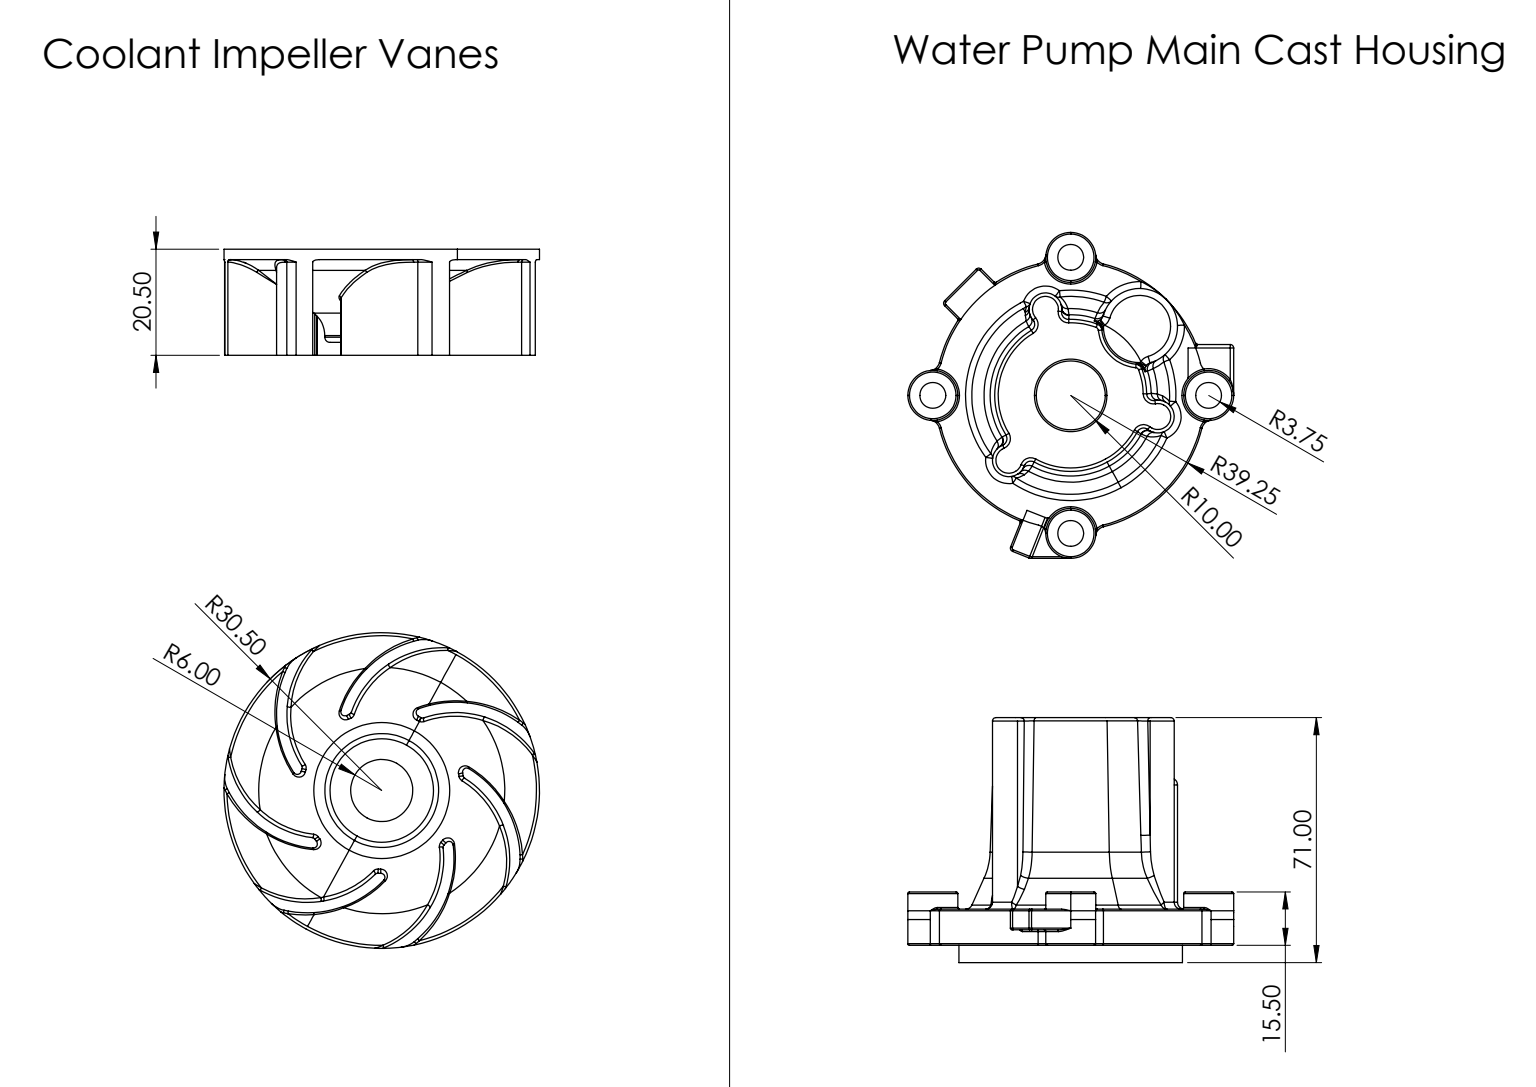
ISO-10303-21;
HEADER;
FILE_DESCRIPTION (('STEP AP214'),
    '1' );
FILE_NAME ('Water Pump Main Cast Housing.step',
    '2026-10-09T13:19:41',
    ( '' ),
    ( '' ),
    'SwSTEP 2.0',
    'SolidWorks 2026',
    '' );
FILE_SCHEMA (( 'AUTOMOTIVE_DESIGN' ));
ENDSEC;

DATA;
#2=DIRECTION ( 'NONE',  ( -1.000000000000000000, 0.000000000000000000, -1.110223024630000146E-15 ) ) ;
#4=CARTESIAN_POINT ( 'NONE',  ( 36.82697894980000086, -80.49999984420000487, -13.57704391360000074 ) ) ;
#5=CARTESIAN_POINT ( 'NONE',  ( 11.49840686428493441, -72.20801872445015590, -27.07840416834825348 ) ) ;
#6=CARTESIAN_POINT ( 'NONE',  ( -18.42950098929999925, -19.15770089200000115, 12.27996177870000061 ) ) ;
#7=ORIENTED_EDGE ( 'NONE', *, *, #8559, .F. ) ;
#11=DIRECTION ( 'NONE',  ( 0.000000000000000000, -1.000000000000000000, 0.000000000000000000 ) ) ;
#15=AXIS2_PLACEMENT_3D ( 'NONE', #13983, #16160, #22740 ) ;
#21=ADVANCED_FACE ( 'NONE', ( #16761 ), #3074, .F. ) ;
#23=CARTESIAN_POINT ( 'NONE',  ( -13.70187146130000144, -57.41946977620000325, 20.98050236089999743 ) ) ;
#24=CARTESIAN_POINT ( 'NONE',  ( -21.94602169939999925, -74.00000000000000000, -32.01791432939999993 ) ) ;
#30=CARTESIAN_POINT ( 'NONE',  ( -7.249922261819999214, -74.00000000000000000, 40.03357376379999977 ) ) ;
#32=CARTESIAN_POINT ( 'NONE',  ( 47.25000000000000000, -79.07667144713899177, -0.2614142261083034491 ) ) ;
#33=ORIENTED_EDGE ( 'NONE', *, *, #25582, .F. ) ;
#35=CARTESIAN_POINT ( 'NONE',  ( 41.00000000000000000, -82.25000000000000000, -10.20110288159999890 ) ) ;
#40=CARTESIAN_POINT ( 'NONE',  ( -38.65569705749999940, -74.00000000000000000, 7.472970580910000216 ) ) ;
#43=ORIENTED_EDGE ( 'NONE', *, *, #10677, .T. ) ;
#49=CARTESIAN_POINT ( 'NONE',  ( 7.691676892869999449, -59.03425911290000272, -22.18797527670000136 ) ) ;
#50=CARTESIAN_POINT ( 'NONE',  ( -12.44168150949999863, -68.42644193349998716, -23.76792160109999585 ) ) ;
#51=CARTESIAN_POINT ( 'NONE',  ( 23.24173891719999929, -63.62917541130000387, -7.733004683649999045 ) ) ;
#52=CARTESIAN_POINT ( 'NONE',  ( 26.61465604159999998, -68.28989644159999273, 0.1578853838729999959 ) ) ;
#53=CARTESIAN_POINT ( 'NONE',  ( 40.75609756099999714, -80.50000000000000000, -7.713029007999999465 ) ) ;
#55=ADVANCED_FACE ( 'NONE', ( #15109 ), #24277, .F. ) ;
#57=FACE_OUTER_BOUND ( 'NONE', #7313, .T. ) ;
#59=ORIENTED_EDGE ( 'NONE', *, *, #8938, .T. ) ;
#63=CIRCLE ( 'NONE', #7047, 3.000000000000002665 ) ;
#65=CARTESIAN_POINT ( 'NONE',  ( 19.49531202280000031, -22.51609091130000095, -8.976487791660000326 ) ) ;
#66=CARTESIAN_POINT ( 'NONE',  ( 22.75333808661257606, -19.47282734142590499, 1.034408943893888599 ) ) ;
#68=ORIENTED_EDGE ( 'NONE', *, *, #28286, .T. ) ;
#69=CARTESIAN_POINT ( 'NONE',  ( 26.87524702870645044, -72.43548166874914784, -11.03468220454692883 ) ) ;
#71=CARTESIAN_POINT ( 'NONE',  ( 8.702528184260000188, -36.35983078039999583, -21.11894135150000196 ) ) ;
#73=PLANE ( 'NONE',  #14194 ) ;
#74=CARTESIAN_POINT ( 'NONE',  ( 22.07903221200000132, -19.15751145089999952, 0.09883320182290000755 ) ) ;
#80=CARTESIAN_POINT ( 'NONE',  ( 7.120909764619999412E-15, -73.00000000000000000, 40.00000000000000000 ) ) ;
#86=TOROIDAL_SURFACE ( 'NONE', #19140, 38.75000000000000000, 0.5000000000000000000 ) ;
#89=CARTESIAN_POINT ( 'NONE',  ( 36.71918983540000880, -74.79610922010000706, -14.73254090590000054 ) ) ;
#90=VECTOR ( 'NONE', #20251, 1000.000000000000000 ) ;
#93=CARTESIAN_POINT ( 'NONE',  ( -13.96596450430000047, -64.58097845250000546, 21.73803617189999926 ) ) ;
#94=CARTESIAN_POINT ( 'NONE',  ( 7.237400523855146872, -74.28469014324819852, 40.42867112560485054 ) ) ;
#96=CARTESIAN_POINT ( 'NONE',  ( 27.02683049547185234, -19.50000000000000000, 2.817888817433860993 ) ) ;
#98=FACE_OUTER_BOUND ( 'NONE', #13994, .T. ) ;
#101=B_SPLINE_CURVE_WITH_KNOTS ( 'NONE', 5,
 ( #4962, #12492, #15099, #10442, #8409, #5814 ),
 .UNSPECIFIED., .F., .F.,
 ( 6, 6 ),
 ( 0.000000000000000000, 1.000000000000000000 ),
 .UNSPECIFIED. ) ;
#102=CARTESIAN_POINT ( 'NONE',  ( 7.432628554159999013, -73.95638562449998687, -39.04162410920000070 ) ) ;
#105=DIRECTION ( 'NONE',  ( -0.7071067811865457964, 0.000000000000000000, -0.7071067811865492381 ) ) ;
#107=CARTESIAN_POINT ( 'NONE',  ( -16.95867319479999935, -74.50000000000000000, 44.10460184009999551 ) ) ;
#108=B_SPLINE_CURVE_WITH_KNOTS ( 'NONE', 3,
 ( #24628, #17928, #4072, #26234, #6261, #26822 ),
 .UNSPECIFIED., .F., .F.,
 ( 4, 2, 4 ),
 ( 0.000000000000000000, 0.5000000000000000000, 1.000000000000000000 ),
 .UNSPECIFIED. ) ;
#110=CARTESIAN_POINT ( 'NONE',  ( -10.71874886979999886, -18.50000000000000000, -18.09957584549999865 ) ) ;
#113=CARTESIAN_POINT ( 'NONE',  ( -13.91698628299999996, -74.00000000000000000, 36.28539016370000070 ) ) ;
#114=FACE_OUTER_BOUND ( 'NONE', #18535, .T. ) ;
#117=ORIENTED_EDGE ( 'NONE', *, *, #9091, .F. ) ;
#120=DIRECTION ( 'NONE',  ( 0.000000000000000000, -1.000000000000000000, 0.000000000000000000 ) ) ;
#122=CARTESIAN_POINT ( 'NONE',  ( 20.98382983661468160, -19.47636826822539646, 9.463978915456744190 ) ) ;
#123=CARTESIAN_POINT ( 'NONE',  ( 23.35514555854173224, -63.53090568636451962, -7.475128354575953260 ) ) ;
#127=CARTESIAN_POINT ( 'NONE',  ( -32.18237743670000128, -74.02983596709999858, -21.99383679990000218 ) ) ;
#131=CARTESIAN_POINT ( 'NONE',  ( -16.95867319479999935, -79.50000000000000000, 44.10460184009999551 ) ) ;
#132=CARTESIAN_POINT ( 'NONE',  ( 19.86285231560000142, -35.99517856170000130, -9.398749189900000189 ) ) ;
#133=CARTESIAN_POINT ( 'NONE',  ( -35.88566914520000495, -79.50000000000000000, -26.69328098980000163 ) ) ;
#134=VERTEX_POINT ( 'NONE', #18050 ) ;
#138=CARTESIAN_POINT ( 'NONE',  ( 30.45033996220000105, -72.00000000000000000, 1.805359716810000181 ) ) ;
#141=CARTESIAN_POINT ( 'NONE',  ( -22.28727701460000077, -80.19684096389998729, -32.37890396869999421 ) ) ;
#142=TOROIDAL_SURFACE ( 'NONE', #23843, 43.34897771020000334, 20.00000000000000000 ) ;
#144=LINE ( 'NONE', #2612, #25776 ) ;
#146=AXIS2_PLACEMENT_3D ( 'NONE', #12009, #28037, #9963 ) ;
#147=ORIENTED_EDGE ( 'NONE', *, *, #2522, .F. ) ;
#150=DIRECTION ( 'NONE',  ( 0.000000000000000000, -1.000000000000000000, 0.000000000000000000 ) ) ;
#151=CARTESIAN_POINT ( 'NONE',  ( -21.99783282880000002, -74.36373701399999447, -32.65606203760000170 ) ) ;
#153=CARTESIAN_POINT ( 'NONE',  ( -27.04683438039999999, -80.00000000000000000, -36.23922253580000330 ) ) ;
#155=CARTESIAN_POINT ( 'NONE',  ( -18.45398243510000214, -18.61794786970000359, 11.31880357350000033 ) ) ;
#160=CARTESIAN_POINT ( 'NONE',  ( 9.189959902346380716, -37.98173178281364670, -22.48186365736571801 ) ) ;
#173=CARTESIAN_POINT ( 'NONE',  ( 5.151434834259999649E-15, -84.50000000000000000, 40.00000000000000000 ) ) ;
#175=EDGE_LOOP ( 'NONE', ( #20884, #12154, #22401, #5530, #9489 ) ) ;
#176=CARTESIAN_POINT ( 'NONE',  ( -12.68423258129999986, -57.45864775709999606, 20.28109956510000345 ) ) ;
#178=VERTEX_POINT ( 'NONE', #329 ) ;
#184=CARTESIAN_POINT ( 'NONE',  ( -11.05730518689999897, -18.50000000000000000, -18.25363368680000065 ) ) ;
#187=FACE_OUTER_BOUND ( 'NONE', #28080, .T. ) ;
#191=EDGE_CURVE ( 'NONE', #3233, #22412, #10451, .T. ) ;
#192=DIRECTION ( 'NONE',  ( 1.000000000000000000, 0.000000000000000000, 0.000000000000000000 ) ) ;
#195=ORIENTED_EDGE ( 'NONE', *, *, #12887, .F. ) ;
#197=CARTESIAN_POINT ( 'NONE',  ( 27.03525773600000193, -69.21553441180000732, 0.3672064477150000505 ) ) ;
#199=CARTESIAN_POINT ( 'NONE',  ( 26.01146028782885011, -74.32246178234187539, -29.34981677889942375 ) ) ;
#200=CARTESIAN_POINT ( 'NONE',  ( 21.14593590499999820, -36.00000000000000000, -10.72085360310000013 ) ) ;
#202=CARTESIAN_POINT ( 'NONE',  ( -11.49099129190000035, -57.47122623430000488, -20.56185124510000151 ) ) ;
#203=EDGE_CURVE ( 'NONE', #6901, #22316, #21214, .T. ) ;
#204=AXIS2_PLACEMENT_3D ( 'NONE', #18687, #25805, #7624 ) ;
#205=B_SPLINE_CURVE_WITH_KNOTS ( 'NONE', 3,
 ( #6928, #20469, #27325, #4883 ),
 .UNSPECIFIED., .F., .F.,
 ( 4, 4 ),
 ( 0.000000000000000000, 1.000000000000000000 ),
 .UNSPECIFIED. ) ;
#206=FACE_OUTER_BOUND ( 'NONE', #10971, .T. ) ;
#208=CYLINDRICAL_SURFACE ( 'NONE', #19119, 0.5000000000000004441 ) ;
#209=ORIENTED_EDGE ( 'NONE', *, *, #22626, .F. ) ;
#212=VERTEX_POINT ( 'NONE', #28690 ) ;
#213=AXIS2_PLACEMENT_3D ( 'NONE', #15083, #23991, #4026 ) ;
#214=CARTESIAN_POINT ( 'NONE',  ( 36.70830968599999977, -79.00000000000000000, -14.75000000000000000 ) ) ;
#219=ORIENTED_EDGE ( 'NONE', *, *, #4229, .F. ) ;
#220=CARTESIAN_POINT ( 'NONE',  ( -3.592524684419479364, -80.18584070972035249, 46.36824188645663014 ) ) ;
#222=CARTESIAN_POINT ( 'NONE',  ( 9.433208476599999059, -36.00000000000000000, -19.93952380609999864 ) ) ;
#223=DIRECTION ( 'NONE',  ( 0.000000000000000000, 1.000000000000000000, 0.000000000000000000 ) ) ;
#226=DIRECTION ( 'NONE',  ( 0.000000000000000000, -1.000000000000000000, 0.000000000000000000 ) ) ;
#227=CARTESIAN_POINT ( 'NONE',  ( 7.460698725479999927E-15, -73.50000000000000000, 40.00000000000000000 ) ) ;
#228=AXIS2_PLACEMENT_3D ( 'NONE', #18983, #14038, #961 ) ;
#232=CARTESIAN_POINT ( 'NONE',  ( -47.25000000000000000, -77.00000000000000000, 3.352534721190000231E-15 ) ) ;
#234=EDGE_CURVE ( 'NONE', #8501, #14143, #28325, .T. ) ;
#236=B_SPLINE_CURVE_WITH_KNOTS ( 'NONE', 5,
 ( #24946, #20125, #22766, #18392, #22315, #639, #13265, #8890, #20574 ),
 .UNSPECIFIED., .F., .F.,
 ( 6, 3, 6 ),
 ( 54.79316277730000451, 55.82679151939999684, 65.31895145690000959 ),
 .UNSPECIFIED. ) ;
#237=CARTESIAN_POINT ( 'NONE',  ( 21.68248887209999864, -36.72282065030000098, -8.793944725010000241 ) ) ;
#238=CARTESIAN_POINT ( 'NONE',  ( -13.11191196370000078, -67.01088404460000447, -22.48946444609999773 ) ) ;
#239=AXIS2_PLACEMENT_3D ( 'NONE', #11995, #25424, #7660 ) ;
#241=CARTESIAN_POINT ( 'NONE',  ( 47.25000000000000000, -82.25000000000000000, 7.327133149349999745E-15 ) ) ;
#242=ORIENTED_EDGE ( 'NONE', *, *, #1523, .T. ) ;
#243=EDGE_CURVE ( 'NONE', #2786, #26473, #23537, .T. ) ;
#246=ORIENTED_EDGE ( 'NONE', *, *, #20790, .F. ) ;
#247=CARTESIAN_POINT ( 'NONE',  ( -14.67079199249999988, -67.87586507669998070, 22.52608771310000080 ) ) ;
#248=CARTESIAN_POINT ( 'NONE',  ( -14.08829788499999935, -63.05022673990000470, 21.64331597370000182 ) ) ;
#249=CARTESIAN_POINT ( 'NONE',  ( 7.244026535080238638, -74.18384006186305157, 40.29424782664090543 ) ) ;
#252=CARTESIAN_POINT ( 'NONE',  ( 20.27618985420000186, -36.00000000000000000, -9.807089787700000727 ) ) ;
#253=CARTESIAN_POINT ( 'NONE',  ( 19.26180799268026078, -18.95847994163547767, 10.44830257471190471 ) ) ;
#254=CARTESIAN_POINT ( 'NONE',  ( -7.325370793560000315, -19.50000000000000000, -24.94672208400000102 ) ) ;
#256=CARTESIAN_POINT ( 'NONE',  ( 20.51180957029163565, -19.46799463732224922, -8.054242869036199792 ) ) ;
#262=ORIENTED_EDGE ( 'NONE', *, *, #10555, .F. ) ;
#266=CIRCLE ( 'NONE', #3945, 6.749999999999999112 ) ;
#267=CARTESIAN_POINT ( 'NONE',  ( 20.31209251039999941, -39.36414254479999641, 10.36558011049999983 ) ) ;
#269=CARTESIAN_POINT ( 'NONE',  ( -7.237400523910141104, -74.28469014252485181, -40.42867112467618540 ) ) ;
#270=CARTESIAN_POINT ( 'NONE',  ( 19.55635611740000002, -19.15716910929999628, 10.13489318640000114 ) ) ;
#271=CARTESIAN_POINT ( 'NONE',  ( -32.83566817454328657, -79.62152845406559720, -22.22906645665674219 ) ) ;
#277=CARTESIAN_POINT ( 'NONE',  ( 21.85414229151949073, -19.48999941750866327, 9.596093625701307417 ) ) ;
#278=CARTESIAN_POINT ( 'NONE',  ( 22.95684285356151122, -62.19234181365079195, -7.315910207710417446 ) ) ;
#279=ORIENTED_EDGE ( 'NONE', *, *, #17232, .T. ) ;
#280=CARTESIAN_POINT ( 'NONE',  ( -37.29988270759999835, -74.00000000000000000, -26.69328098980000163 ) ) ;
#281=ORIENTED_EDGE ( 'NONE', *, *, #28769, .F. ) ;
#285=ORIENTED_EDGE ( 'NONE', *, *, #19460, .T. ) ;
#287=EDGE_CURVE ( 'NONE', #8306, #13803, #18426, .T. ) ;
#288=EDGE_LOOP ( 'NONE', ( #10036, #21342, #22222, #19692, #5253 ) ) ;
#291=DIRECTION ( 'NONE',  ( 0.000000000000000000, -1.000000000000000000, 0.000000000000000000 ) ) ;
#293=DIRECTION ( 'NONE',  ( 0.9704142011833033488, 0.000000000000000000, -0.2414462220490755373 ) ) ;
#297=EDGE_CURVE ( 'NONE', #22756, #7089, #25863, .T. ) ;
#300=VERTEX_POINT ( 'NONE', #17646 ) ;
#301=EDGE_CURVE ( 'NONE', #178, #23662, #773, .T. ) ;
#304=CARTESIAN_POINT ( 'NONE',  ( 0.000000000000000000, -18.50000000000000000, 0.000000000000000000 ) ) ;
#305=CARTESIAN_POINT ( 'NONE',  ( -21.75993564049999662, -74.26505820949999759, -32.61013845149999923 ) ) ;
#311=CARTESIAN_POINT ( 'NONE',  ( 23.49021206360000136, -61.37513324760000444, 10.53893526849999951 ) ) ;
#312=DIRECTION ( 'NONE',  ( 0.9952295494196654602, 0.000000000000000000, -0.09756097560976667582 ) ) ;
#315=CARTESIAN_POINT ( 'NONE',  ( 47.13373881900000129, -79.60558632359999365, -1.850014393339999952 ) ) ;
#319=ORIENTED_EDGE ( 'NONE', *, *, #5451, .T. ) ;
#321=VERTEX_POINT ( 'NONE', #13849 ) ;
#322=CARTESIAN_POINT ( 'NONE',  ( 22.48431106502128785, -26.11410610478370131, 9.982359961558207928 ) ) ;
#323=CARTESIAN_POINT ( 'NONE',  ( 32.39999999999999858, -89.50000000000000000, 3.967724586379999025E-15 ) ) ;
#329=CARTESIAN_POINT ( 'NONE',  ( 32.25000000000000000, -74.00000000000000000, 1.484822157706350179E-15 ) ) ;
#330=DIRECTION ( 'NONE',  ( -0.9993816408608721114, 0.000000000000000000, 0.03516156865429608674 ) ) ;
#331=EDGE_CURVE ( 'NONE', #2214, #4550, #8167, .T. ) ;
#332=CARTESIAN_POINT ( 'NONE',  ( -10.44633092189999957, -19.46971296670000129, -20.02005348129999973 ) ) ;
#333=ORIENTED_EDGE ( 'NONE', *, *, #19304, .T. ) ;
#334=ADVANCED_FACE ( 'NONE', ( #7744 ), #22137, .T. ) ;
#336=CARTESIAN_POINT ( 'NONE',  ( -20.38472824830307317, -61.37133910092857292, 12.44426916512128223 ) ) ;
#338=ORIENTED_EDGE ( 'NONE', *, *, #4914, .F. ) ;
#341=CARTESIAN_POINT ( 'NONE',  ( -22.62548402540000225, -71.48510949040000639, 17.99032368389999803 ) ) ;
#342=ORIENTED_EDGE ( 'NONE', *, *, #9374, .T. ) ;
#345=CARTESIAN_POINT ( 'NONE',  ( 25.28766026403006961, -74.25610482756999886, -29.93611247388432162 ) ) ;
#346=CARTESIAN_POINT ( 'NONE',  ( -19.90266458460165566, -57.44036973094087273, 14.20824301555132152 ) ) ;
#347=CARTESIAN_POINT ( 'NONE',  ( 22.71963930829999967, -57.44066855169999997, -9.099147364980002095 ) ) ;
#361=DIRECTION ( 'NONE',  ( 0.000000000000000000, -1.000000000000000000, 0.000000000000000000 ) ) ;
#363=CARTESIAN_POINT ( 'NONE',  ( 8.154561305720001485, -36.99980119890000196, -21.51307946880000088 ) ) ;
#364=EDGE_CURVE ( 'NONE', #27046, #11872, #7856, .T. ) ;
#365=CARTESIAN_POINT ( 'NONE',  ( 8.054097215812880961, -19.46843057288947421, -20.48836643782571443 ) ) ;
#378=CARTESIAN_POINT ( 'NONE',  ( 26.29305724443631220, -63.71690337527751069, 1.488180441977877466 ) ) ;
#381=CARTESIAN_POINT ( 'NONE',  ( -10.61287167059999881, -19.46510050329999686, 19.30934957549999709 ) ) ;
#383=CARTESIAN_POINT ( 'NONE',  ( 36.31166979920000415, -74.62997809459999132, -14.90098611910000059 ) ) ;
#387=CARTESIAN_POINT ( 'NONE',  ( -12.68423313600000135, -57.45864720369999645, 20.28110700490000085 ) ) ;
#388=CARTESIAN_POINT ( 'NONE',  ( -1.314504061159999897E-13, -19.50000000000000000, -1.119104808819999722E-13 ) ) ;
#390=CARTESIAN_POINT ( 'NONE',  ( 18.71434861636577907, -18.49999996077436037, 10.15134080778569370 ) ) ;
#392=B_SPLINE_CURVE_WITH_KNOTS ( 'NONE', 5,
 ( #381, #18132, #9225, #11262, #10956, #27029 ),
 .UNSPECIFIED., .F., .F.,
 ( 6, 6 ),
 ( 0.000000000000000000, 1.000000000000000000 ),
 .UNSPECIFIED. ) ;
#394=ORIENTED_EDGE ( 'NONE', *, *, #12962, .T. ) ;
#395=CARTESIAN_POINT ( 'NONE',  ( -7.253647055860000137, -74.31845592130000000, -40.32201634399999790 ) ) ;
#396=CARTESIAN_POINT ( 'NONE',  ( 30.63887047069549752, -74.17816095543288668, -24.34389095944435155 ) ) ;
#404=DIRECTION ( 'NONE',  ( 0.000000000000000000, 0.000000000000000000, -1.000000000000000000 ) ) ;
#405=CARTESIAN_POINT ( 'NONE',  ( 7.670973119660000172, -34.59820496239999699, -21.21808926809999818 ) ) ;
#409=CARTESIAN_POINT ( 'NONE',  ( -1.598721155459999804E-14, -84.50000000000000000, 7.105427357599999217E-15 ) ) ;
#413=CARTESIAN_POINT ( 'NONE',  ( -12.08584015490000141, -69.49854784190000601, -25.11440668759999895 ) ) ;
#414=CARTESIAN_POINT ( 'NONE',  ( -9.356041104380000917, -74.50000000000000000, -37.60355029590000697 ) ) ;
#419=EDGE_CURVE ( 'NONE', #9997, #22379, #25806, .T. ) ;
#423=B_SPLINE_CURVE_WITH_KNOTS ( 'NONE', 5,
 ( #28794, #10856, #8982, #22117, #26629, #17888, #2016, #26198, #19767 ),
 .UNSPECIFIED., .F., .F.,
 ( 6, 3, 6 ),
 ( 0.000000000000000000, 0.2815520576815128129, 1.000000000000000000 ),
 .UNSPECIFIED. ) ;
#425=B_SPLINE_CURVE_WITH_KNOTS ( 'NONE', 3,
 ( #6749, #17383, #15612, #10933, #24370, #2227, #8482, #26130 ),
 .UNSPECIFIED., .F., .F.,
 ( 4, 2, 2, 4 ),
 ( 0.000000000000000000, 0.5000000000000000000, 0.7500000000000000000, 1.000000000000000000 ),
 .UNSPECIFIED. ) ;
#426=CARTESIAN_POINT ( 'NONE',  ( -10.50000000000000000, -89.00000000000000000, 6.411537967209999764E-15 ) ) ;
#428=ORIENTED_EDGE ( 'NONE', *, *, #14886, .F. ) ;
#431=ORIENTED_EDGE ( 'NONE', *, *, #22851, .T. ) ;
#434=CARTESIAN_POINT ( 'NONE',  ( 47.03393487260000683, -74.30497055530000239, -1.819362492409999810 ) ) ;
#437=CARTESIAN_POINT ( 'NONE',  ( -11.33957729739370635, -60.31986010322346203, 20.76858926670032446 ) ) ;
#442=CARTESIAN_POINT ( 'NONE',  ( 36.44627168800000305, -74.06782051840001202, -14.22901210950000106 ) ) ;
#444=CARTESIAN_POINT ( 'NONE',  ( -39.96417052329999819, -74.08839659379999887, 7.268571389559999929 ) ) ;
#445=CARTESIAN_POINT ( 'NONE',  ( -21.96029098729999873, -74.01681409379999366, -32.14278154310000701 ) ) ;
#448=TOROIDAL_SURFACE ( 'NONE', #14380, 3.500000000000000000, 0.5000000000000000000 ) ;
#451=CARTESIAN_POINT ( 'NONE',  ( -18.42673315119999700, -19.46723765599999822, 12.71460005940000038 ) ) ;
#452=VERTEX_POINT ( 'NONE', #2600 ) ;
#453=CIRCLE ( 'NONE', #16705, 25.14975229270000057 ) ;
#455=DIRECTION ( 'NONE',  ( 0.9952295494196655712, 0.000000000000000000, -0.09756097560976655092 ) ) ;
#458=CARTESIAN_POINT ( 'NONE',  ( 23.02872706139999792, -64.78279487710000240, 10.89319034239999873 ) ) ;
#461=CYLINDRICAL_SURFACE ( 'NONE', #14611, 7.250000000000004441 ) ;
#462=EDGE_LOOP ( 'NONE', ( #7534, #13266, #11753, #16100 ) ) ;
#464=CARTESIAN_POINT ( 'NONE',  ( -14.29547445250000060, -74.00000000000000000, 45.69901703040000029 ) ) ;
#466=CARTESIAN_POINT ( 'NONE',  ( -11.32870268019999926, -60.33034294469999992, -22.21640803110000206 ) ) ;
#468=CARTESIAN_POINT ( 'NONE',  ( 25.82404717150000195, -69.73911356650000926, -8.782782835009999900 ) ) ;
#469=DIRECTION ( 'NONE',  ( 1.000000000000000000, 0.000000000000000000, 0.000000000000000000 ) ) ;
#470=ORIENTED_EDGE ( 'NONE', *, *, #14294, .F. ) ;
#471=CARTESIAN_POINT ( 'NONE',  ( 7.815970093360001426E-15, -84.50000000000000000, -40.00000000000000000 ) ) ;
#472=TOROIDAL_SURFACE ( 'NONE', #16728, 1.500000000000000000, 0.5000000000000000000 ) ;
#473=ORIENTED_EDGE ( 'NONE', *, *, #11539, .F. ) ;
#478=CIRCLE ( 'NONE', #7895, 3.000000000000000000 ) ;
#479=CIRCLE ( 'NONE', #4152, 28.68388914670000034 ) ;
#480=PLANE ( 'NONE',  #18583 ) ;
#482=CARTESIAN_POINT ( 'NONE',  ( -10.10487300439999991, -18.62107971969999909, -21.27518202489999766 ) ) ;
#483=CARTESIAN_POINT ( 'NONE',  ( 21.51792335492191199, -37.40300027226001589, -7.702379948524843201 ) ) ;
#486=CARTESIAN_POINT ( 'NONE',  ( -20.39638010391581702, -61.43221488831640897, 12.45288284519579314 ) ) ;
#495=CARTESIAN_POINT ( 'NONE',  ( -20.45998242170000125, -52.56313962710000709, 14.78974999389999923 ) ) ;
#496=CARTESIAN_POINT ( 'NONE',  ( -19.95527577780000072, -57.47855601759999900, 12.14622656770000120 ) ) ;
#498=CARTESIAN_POINT ( 'NONE',  ( 22.40625751809999855, -60.56287431679999855, -8.064917839230000496 ) ) ;
#499=EDGE_CURVE ( 'NONE', #18811, #12707, #22077, .T. ) ;
#500=CARTESIAN_POINT ( 'NONE',  ( 27.49606017789999868, -67.46051290640001241, 1.934794646639999893 ) ) ;
#501=CARTESIAN_POINT ( 'NONE',  ( -10.27945668490000131, -18.50000000000000000, 18.70272521329999904 ) ) ;
#504=EDGE_LOOP ( 'NONE', ( #699, #16423, #5514, #12046 ) ) ;
#505=CARTESIAN_POINT ( 'NONE',  ( 10.20110288159999890, -74.50000000000000000, -41.00000000000000000 ) ) ;
#510=CARTESIAN_POINT ( 'NONE',  ( 7.323170304809999642, -73.87254094300001839, 39.07240670449999698 ) ) ;
#515=CARTESIAN_POINT ( 'NONE',  ( 26.80884837331130655, -72.62863614316471228, -10.52387429041271538 ) ) ;
#517=CARTESIAN_POINT ( 'NONE',  ( 8.994939661169999212, -36.15004583290000539, -20.77616074780000233 ) ) ;
#518=CARTESIAN_POINT ( 'NONE',  ( 8.620126422187169624, -19.47938362974832316, -19.97534244429069616 ) ) ;
#522=CARTESIAN_POINT ( 'NONE',  ( 36.28164458690000060, -74.50000000000000000, -14.97346873880000118 ) ) ;
#524=CARTESIAN_POINT ( 'NONE',  ( -2.568686407175419184, -19.48618186047746548, -23.50321383691693100 ) ) ;
#525=CYLINDRICAL_SURFACE ( 'NONE', #18143, 7.249999999999999112 ) ;
#527=DIRECTION ( 'NONE',  ( 1.000000000000000000, 0.000000000000000000, 0.000000000000000000 ) ) ;
#528=CARTESIAN_POINT ( 'NONE',  ( -39.10791602276640333, -73.54003775238672347, 7.198125313980217932 ) ) ;
#529=DIRECTION ( 'NONE',  ( -0.2414462220490760924, 0.000000000000000000, -0.9704142011833030157 ) ) ;
#532=ORIENTED_EDGE ( 'NONE', *, *, #4377, .T. ) ;
#533=ADVANCED_FACE ( 'NONE', ( #11147 ), #17891, .T. ) ;
#534=CARTESIAN_POINT ( 'NONE',  ( 36.25731322790000632, -74.69416361989999587, -15.03231676859999943 ) ) ;
#535=CARTESIAN_POINT ( 'NONE',  ( -22.29222582179728107, -79.74578553650356127, -32.80938733156981613 ) ) ;
#537=AXIS2_PLACEMENT_3D ( 'NONE', #16966, #27223, #1016 ) ;
#538=EDGE_CURVE ( 'NONE', #11457, #18344, #12745, .T. ) ;
#540=CARTESIAN_POINT ( 'NONE',  ( -11.41594931139999858, -19.46510050329999686, -18.84569254350000023 ) ) ;
#541=CARTESIAN_POINT ( 'NONE',  ( 19.99082350619999815, -35.29518274429999991, -8.963945870050000764 ) ) ;
#544=DIRECTION ( 'NONE',  ( 0.000000000000000000, -1.000000000000000000, 0.000000000000000000 ) ) ;
#548=CARTESIAN_POINT ( 'NONE',  ( 21.56931449510000220, -36.56979901409999911, -6.850353628320000610 ) ) ;
#553=LINE ( 'NONE', #19920, #16709 ) ;
#554=DIRECTION ( 'NONE',  ( 1.000000000000000000, 0.000000000000000000, 0.000000000000000000 ) ) ;
#556=AXIS2_PLACEMENT_3D ( 'NONE', #15444, #1512, #21732 ) ;
#559=VECTOR ( 'NONE', #7059, 1000.000000000000000 ) ;
#560=CARTESIAN_POINT ( 'NONE',  ( -13.82310862920000005, -74.00000000000000000, 36.20061004779999791 ) ) ;
#561=CARTESIAN_POINT ( 'NONE',  ( -21.72229115340000050, -67.06690763590000870, 14.40139912269999911 ) ) ;
#563=EDGE_LOOP ( 'NONE', ( #25536, #17511, #4054, #11653 ) ) ;
#564=CARTESIAN_POINT ( 'NONE',  ( -12.47289874710000035, -69.87861895790000233, -24.46965691790000363 ) ) ;
#565=EDGE_CURVE ( 'NONE', #21465, #19989, #2562, .T. ) ;
#566=DIRECTION ( 'NONE',  ( 0.000000000000000000, 1.000000000000000000, 0.000000000000000000 ) ) ;
#568=DIRECTION ( 'NONE',  ( 0.000000000000000000, -1.000000000000000000, 0.000000000000000000 ) ) ;
#569=CARTESIAN_POINT ( 'NONE',  ( 7.135467692469593892, -73.63089972761061119, -38.71641001238787538 ) ) ;
#574=EDGE_CURVE ( 'NONE', #4330, #15463, #9981, .T. ) ;
#580=ORIENTED_EDGE ( 'NONE', *, *, #6138, .F. ) ;
#582=CARTESIAN_POINT ( 'NONE',  ( -16.86265888959999870, -79.50000000000000000, 45.21850545039999503 ) ) ;
#583=CARTESIAN_POINT ( 'NONE',  ( 10.08829703670000022, -36.00000000000000000, -20.49602678049999938 ) ) ;
#585=CARTESIAN_POINT ( 'NONE',  ( 7.246063797170706700, -73.82871504787716788, -39.75929607700521018 ) ) ;
#586=CARTESIAN_POINT ( 'NONE',  ( -11.50280172684225732, -61.70151683873936577, 21.01880821135103972 ) ) ;
#587=ORIENTED_EDGE ( 'NONE', *, *, #16283, .F. ) ;
#588=CARTESIAN_POINT ( 'NONE',  ( 22.44118743278407280, -65.00127796776330058, 11.39886732859506502 ) ) ;
#591=CARTESIAN_POINT ( 'NONE',  ( -2.675358685650000012, -67.79480919600000277, -26.71434926430000090 ) ) ;
#592=PLANE ( 'NONE',  #25559 ) ;
#593=CARTESIAN_POINT ( 'NONE',  ( -15.48552837409999938, -71.82739780379999672, 23.60563397449999812 ) ) ;
#595=DIRECTION ( 'NONE',  ( 1.000000000000000000, 0.000000000000000000, 0.000000000000000000 ) ) ;
#597=CARTESIAN_POINT ( 'NONE',  ( 25.46032906830000186, -64.78279197330000727, 0.8694561931790000253 ) ) ;
#598=CARTESIAN_POINT ( 'NONE',  ( -21.94602169939999925, -74.00000000000000000, -32.01791432939999993 ) ) ;
#600=CARTESIAN_POINT ( 'NONE',  ( -19.61617179850000170, -45.99935878759999497, 11.93235644279999974 ) ) ;
#601=VECTOR ( 'NONE', #24406, 1000.000000000000000 ) ;
#603=CARTESIAN_POINT ( 'NONE',  ( -18.66344010299999923, -18.85523519099999845, 11.44727505870000073 ) ) ;
#607=EDGE_CURVE ( 'NONE', #27919, #28507, #7827, .T. ) ;
#608=DIRECTION ( 'NONE',  ( 0.3388759126238506392, 0.000000000000000000, -0.9408310772095872521 ) ) ;
#609=CARTESIAN_POINT ( 'NONE',  ( 8.964388214039999525, -35.14340553630000130, -19.96644199109999818 ) ) ;
#611=DIRECTION ( 'NONE',  ( 0.000000000000000000, 1.000000000000000000, 0.000000000000000000 ) ) ;
#613=CARTESIAN_POINT ( 'NONE',  ( 47.25000000000000000, -79.00000000000000000, -7.713829575100000215E-13 ) ) ;
#615=CARTESIAN_POINT ( 'NONE',  ( -11.81677247600000058, -62.06858034060000762, -21.05646513629999816 ) ) ;
#616=CARTESIAN_POINT ( 'NONE',  ( 25.13747520559999771, -67.81660459209999203, -9.975487151870000346 ) ) ;
#617=CARTESIAN_POINT ( 'NONE',  ( 9.475766568499999210, -35.50000000000000000, -19.97576656850000276 ) ) ;
#619=DIRECTION ( 'NONE',  ( 0.000000000000000000, 1.000000000000000000, 0.000000000000000000 ) ) ;
#624=AXIS2_PLACEMENT_3D ( 'NONE', #1463, #10304, #17029 ) ;
#625=CARTESIAN_POINT ( 'NONE',  ( -2.579145438419999881, -53.53226321310000202, -25.13754169039999908 ) ) ;
#626=EDGE_CURVE ( 'NONE', #27517, #13659, #27786, .T. ) ;
#628=CARTESIAN_POINT ( 'NONE',  ( -10.49491320851042708, -19.48298603870330581, -20.96686108838342832 ) ) ;
#631=CARTESIAN_POINT ( 'NONE',  ( 47.24130919904909121, -79.14360025649037311, -0.4895094584727857079 ) ) ;
#634=CARTESIAN_POINT ( 'NONE',  ( -20.38860325545200070, -61.39165777032547311, 12.44713039966608292 ) ) ;
#635=DIRECTION ( 'NONE',  ( 0.000000000000000000, 1.000000000000000000, 0.000000000000000000 ) ) ;
#637=DIRECTION ( 'NONE',  ( -1.000000000000000000, 0.000000000000000000, 0.000000000000000000 ) ) ;
#639=CARTESIAN_POINT ( 'NONE',  ( 7.235472567440000446, -61.68715554919999988, -22.75972229710000150 ) ) ;
#643=DIRECTION ( 'NONE',  ( 0.000000000000000000, 1.000000000000000000, 0.000000000000000000 ) ) ;
#644=CARTESIAN_POINT ( 'NONE',  ( 22.30843460160000191, -36.00000000000000000, -11.28235740200000059 ) ) ;
#645=CARTESIAN_POINT ( 'NONE',  ( 23.70193923009999892, -61.68490361759999985, -9.613352042829999888 ) ) ;
#647=CARTESIAN_POINT ( 'NONE',  ( 25.12978992150000224, -65.01950800350000748, 0.1513709550449999774 ) ) ;
#648=DIRECTION ( 'NONE',  ( 1.000000000000000000, 0.000000000000000000, 0.000000000000000000 ) ) ;
#650=CARTESIAN_POINT ( 'NONE',  ( -19.68803156824991163, -18.87168151093004198, 14.53288012867929702 ) ) ;
#654=CARTESIAN_POINT ( 'NONE',  ( 7.135467526410000261, -73.50000000000000000, 38.71641004229999794 ) ) ;
#655=CARTESIAN_POINT ( 'NONE',  ( 7.383549334360000493, -18.50000000000000000, -19.69582310909999734 ) ) ;
#656=CARTESIAN_POINT ( 'NONE',  ( 23.35112319427650007, -19.48210987405916583, 1.375628917947436136 ) ) ;
#659=CARTESIAN_POINT ( 'NONE',  ( 9.018047497980001381, -36.17942459150000190, -20.85226661109999924 ) ) ;
#660=AXIS2_PLACEMENT_3D ( 'NONE', #6377, #25920, #4047 ) ;
#663=EDGE_CURVE ( 'NONE', #10505, #5317, #25363, .T. ) ;
#666=CARTESIAN_POINT ( 'NONE',  ( 21.48302338326642413, -36.56890885472610364, -7.253824468342653375 ) ) ;
#668=DIRECTION ( 'NONE',  ( -0.7071067811865470176, 0.000000000000000000, 0.7071067811865480168 ) ) ;
#671=CARTESIAN_POINT ( 'NONE',  ( -0.8441209747499999194, -45.99930305819999887, -22.94698520209999870 ) ) ;
#674=DIRECTION ( 'NONE',  ( 0.000000000000000000, 1.000000000000000000, 0.000000000000000000 ) ) ;
#675=AXIS2_PLACEMENT_3D ( 'NONE', #1404, #7809, #1680 ) ;
#676=CARTESIAN_POINT ( 'NONE',  ( 41.00000000000000000, -74.50000000000000000, 10.20110288159999890 ) ) ;
#677=CARTESIAN_POINT ( 'NONE',  ( 22.20693316850000087, -40.71455396009999816, -8.968806686309999776 ) ) ;
#678=CARTESIAN_POINT ( 'NONE',  ( 19.97576656849999921, -72.00000000000000000, -19.97576656849999921 ) ) ;
#680=ORIENTED_EDGE ( 'NONE', *, *, #13024, .F. ) ;
#681=CARTESIAN_POINT ( 'NONE',  ( 36.59408416780000550, -74.85684975549999365, -14.74361069959999959 ) ) ;
#682=CARTESIAN_POINT ( 'NONE',  ( -32.66809844459999823, -74.41869006989999491, -22.00101410510000122 ) ) ;
#684=AXIS2_PLACEMENT_3D ( 'NONE', #27269, #20999, #20718 ) ;
#686=CARTESIAN_POINT ( 'NONE',  ( 9.004237477329999351, -35.65077419509999146, -19.54737253879999770 ) ) ;
#687=CARTESIAN_POINT ( 'NONE',  ( 23.18812391385057126, -58.58546841852697895, 10.40058855015711892 ) ) ;
#688=CARTESIAN_POINT ( 'NONE',  ( 20.11250903250000022, -36.00000000000000000, -9.561259576869998611 ) ) ;
#689=CARTESIAN_POINT ( 'NONE',  ( 21.16767063019999995, -36.23936169889999803, -8.913590358700000493 ) ) ;
#693=ORIENTED_EDGE ( 'NONE', *, *, #2892, .T. ) ;
#699=ORIENTED_EDGE ( 'NONE', *, *, #16855, .F. ) ;
#700=EDGE_CURVE ( 'NONE', #27146, #28156, #13733, .T. ) ;
#702=DIRECTION ( 'NONE',  ( 0.000000000000000000, 0.000000000000000000, -1.000000000000000000 ) ) ;
#705=CARTESIAN_POINT ( 'NONE',  ( -7.250038883930940870, -73.95086734744796786, -39.95935625309049755 ) ) ;
#706=ADVANCED_FACE ( 'NONE', ( #3044 ), #14624, .F. ) ;
#707=CARTESIAN_POINT ( 'NONE',  ( -14.57729759870000130, -74.12911414260001663, 36.26887511289999821 ) ) ;
#708=CARTESIAN_POINT ( 'NONE',  ( -21.87632299289999693, -67.55173099820000004, 16.08189821899999927 ) ) ;
#710=ORIENTED_EDGE ( 'NONE', *, *, #14232, .F. ) ;
#711=CARTESIAN_POINT ( 'NONE',  ( -12.46915732870000149, -70.42119542689999889, -24.73933575500000259 ) ) ;
#712=CARTESIAN_POINT ( 'NONE',  ( 8.142471319829999388, -22.47117226119999955, -20.59194991089999860 ) ) ;
#713=DIRECTION ( 'NONE',  ( 0.9295286103719528903, 0.000000000000000000, 0.3687499999999813705 ) ) ;
#714=CARTESIAN_POINT ( 'NONE',  ( 19.96073932771978221, -19.46608320370787482, 9.833604944531050052 ) ) ;
#716=ORIENTED_EDGE ( 'NONE', *, *, #14608, .F. ) ;
#717=CIRCLE ( 'NONE', #12731, 2.000000035459998493 ) ;
#719=CARTESIAN_POINT ( 'NONE',  ( -2.487950882160000265, -57.83919435140000331, -24.63540447140000111 ) ) ;
#723=VERTEX_POINT ( 'NONE', #5055 ) ;
#728=CARTESIAN_POINT ( 'NONE',  ( 21.09474350280000010, -36.06031159909999673, -9.858094216790000530 ) ) ;
#729=ADVANCED_FACE ( 'NONE', ( #27924 ), #23339, .F. ) ;
#730=CARTESIAN_POINT ( 'NONE',  ( 47.14031554959999681, -74.51859318479999672, -1.361887490440000015 ) ) ;
#732=CARTESIAN_POINT ( 'NONE',  ( 7.250349464191871540, -73.96150430845511892, -39.97648509748324130 ) ) ;
#733=CARTESIAN_POINT ( 'NONE',  ( -11.45517213598250095, -61.33682282352064874, 20.94728758455344675 ) ) ;
#734=EDGE_CURVE ( 'NONE', #9200, #23505, #24513, .T. ) ;
#735=CARTESIAN_POINT ( 'NONE',  ( 24.22382764319999993, -64.24504439390000243, 10.76339940740000145 ) ) ;
#737=CARTESIAN_POINT ( 'NONE',  ( -2.901733356760000326, -65.28594186040000125, -26.69036142120000221 ) ) ;
#738=ADVANCED_FACE ( 'NONE', ( #6191 ), #18923, .F. ) ;
#741=ORIENTED_EDGE ( 'NONE', *, *, #6844, .T. ) ;
#742=EDGE_CURVE ( 'NONE', #12644, #2204, #16508, .T. ) ;
#743=CARTESIAN_POINT ( 'NONE',  ( 36.61501056740000593, -74.18926003920000767, -14.42630212289999925 ) ) ;
#745=CARTESIAN_POINT ( 'NONE',  ( 25.05740514639999716, -58.84796781909999908, 1.374148744239999997 ) ) ;
#746=CARTESIAN_POINT ( 'NONE',  ( -20.94815322850000072, -63.05060005210000185, 15.10280677179999920 ) ) ;
#750=CARTESIAN_POINT ( 'NONE',  ( 36.73784911806745868, -74.38638021456385729, -14.53963971729679017 ) ) ;
#751=ORIENTED_EDGE ( 'NONE', *, *, #16283, .T. ) ;
#753=CARTESIAN_POINT ( 'NONE',  ( 20.73451516309999931, -60.34941021230000047, 11.32693620240000065 ) ) ;
#754=CARTESIAN_POINT ( 'NONE',  ( -2.664535259099999805E-15, -84.00000000000000000, -40.00000000000000000 ) ) ;
#756=CARTESIAN_POINT ( 'NONE',  ( -4.459621975350000156, -72.00000000000000000, -28.73485931899999812 ) ) ;
#757=ORIENTED_EDGE ( 'NONE', *, *, #538, .T. ) ;
#758=CARTESIAN_POINT ( 'NONE',  ( 46.85840109400000131, -80.01819416290000220, -2.680681327329999863 ) ) ;
#759=CARTESIAN_POINT ( 'NONE',  ( -11.12510688389999913, -19.15751128430000350, 19.07158749389999741 ) ) ;
#760=CARTESIAN_POINT ( 'NONE',  ( -12.19871700799999914, -59.03921360480000402, -19.98710743599999873 ) ) ;
#761=CARTESIAN_POINT ( 'NONE',  ( 37.10328156088058194, -79.93994609586795264, -14.09141366765611636 ) ) ;
#762=CARTESIAN_POINT ( 'NONE',  ( 24.78973582949999965, -64.24504403269999386, -10.08507979989999903 ) ) ;
#766=DIRECTION ( 'NONE',  ( -1.000000000000000000, 0.000000000000000000, -1.224606353820000075E-16 ) ) ;
#768=CARTESIAN_POINT ( 'NONE',  ( 22.78965548680000097, -53.78538132969999452, 10.19408277159999976 ) ) ;
#771=CARTESIAN_POINT ( 'NONE',  ( 45.89652019488737977, -80.18584073604786511, -4.323399995959095854 ) ) ;
#773=CIRCLE ( 'NONE', #24460, 7.750000000000000000 ) ;
#774=ORIENTED_EDGE ( 'NONE', *, *, #17934, .T. ) ;
#775=FACE_OUTER_BOUND ( 'NONE', #22718, .T. ) ;
#776=CARTESIAN_POINT ( 'NONE',  ( 40.00000000000000000, -80.50000000000000000, 0.000000000000000000 ) ) ;
#777=CARTESIAN_POINT ( 'NONE',  ( 13.75178900340000077, -72.82938648530000592, 25.17248092229999656 ) ) ;
#778=CARTESIAN_POINT ( 'NONE',  ( -10.38787484979999931, -19.16887642500000055, -20.73616781340000159 ) ) ;
#779=CARTESIAN_POINT ( 'NONE',  ( 46.40218322401350548, -80.00000000000000000, -4.271240362889383135 ) ) ;
#780=ORIENTED_EDGE ( 'NONE', *, *, #25866, .T. ) ;
#781=CARTESIAN_POINT ( 'NONE',  ( -32.25831118210000170, -80.18584106479998752, -22.46797580029999963 ) ) ;
#782=CARTESIAN_POINT ( 'NONE',  ( -20.68567502208468767, -62.76183479546326538, 12.67672343809073254 ) ) ;
#783=CARTESIAN_POINT ( 'NONE',  ( 46.25000000000000000, -74.00000000000000000, -4.582575694960000057 ) ) ;
#785=ORIENTED_EDGE ( 'NONE', *, *, #21487, .T. ) ;
#787=DIRECTION ( 'NONE',  ( 1.000000000000000000, 0.000000000000000000, 0.000000000000000000 ) ) ;
#789=CARTESIAN_POINT ( 'NONE',  ( -16.04004518150000180, -79.50000000000000000, 40.43303297039999933 ) ) ;
#792=CARTESIAN_POINT ( 'NONE',  ( -19.54048411309999977, -52.63055504180000099, 12.61913916920000034 ) ) ;
#794=CARTESIAN_POINT ( 'NONE',  ( -19.68647263592396257, -57.47571017175199160, 12.70082573817182592 ) ) ;
#796=ADVANCED_FACE ( 'NONE', ( #21061 ), #26133, .F. ) ;
#797=CARTESIAN_POINT ( 'NONE',  ( 26.57205606840000200, -68.20221627489999605, 0.6012252253150000003 ) ) ;
#798=ORIENTED_EDGE ( 'NONE', *, *, #9993, .T. ) ;
#799=CARTESIAN_POINT ( 'NONE',  ( 20.49657866619999780, -57.47855601759999900, 11.20866246179999948 ) ) ;
#800=DIRECTION ( 'NONE',  ( 1.000000000000000000, 0.000000000000000000, -1.165696672470000011E-15 ) ) ;
#804=CYLINDRICAL_SURFACE ( 'NONE', #2762, 4.750000000000001776 ) ;
#806=EDGE_CURVE ( 'NONE', #21652, #15706, #7691, .T. ) ;
#809=FACE_OUTER_BOUND ( 'NONE', #5937, .T. ) ;
#812=CYLINDRICAL_SURFACE ( 'NONE', #25089, 3.749999999999996447 ) ;
#814=CARTESIAN_POINT ( 'NONE',  ( -40.29424782663165416, -74.18384006185542034, 7.244026535080610785 ) ) ;
#817=ORIENTED_EDGE ( 'NONE', *, *, #25510, .T. ) ;
#818=CARTESIAN_POINT ( 'NONE',  ( -2.235159051901111749, -19.47504441211092896, -22.82101578340120795 ) ) ;
#819=CYLINDRICAL_SURFACE ( 'NONE', #10657, 0.4999999999999967804 ) ;
#820=CARTESIAN_POINT ( 'NONE',  ( -2.495716009669999735, -52.58489974409999945, -24.49317771890000017 ) ) ;
#822=FACE_OUTER_BOUND ( 'NONE', #17874, .T. ) ;
#823=CARTESIAN_POINT ( 'NONE',  ( 21.79230230059999940, -37.95144147500000287, -8.472395268590000583 ) ) ;
#826=EDGE_LOOP ( 'NONE', ( #24817, #21134, #2537, #3950, #25575 ) ) ;
#827=CARTESIAN_POINT ( 'NONE',  ( -32.69645381549999286, -74.45114023669999881, -21.71458329279999688 ) ) ;
#830=ADVANCED_FACE ( 'NONE', ( #5326 ), #25668, .F. ) ;
#831=CARTESIAN_POINT ( 'NONE',  ( -13.39422214930000088, -65.52751332760001901, 21.76797051860000209 ) ) ;
#832=CARTESIAN_POINT ( 'NONE',  ( 20.42417383799999797, -34.94312134569999984, -8.791129100729998314 ) ) ;
#834=EDGE_CURVE ( 'NONE', #24358, #3863, #28590, .T. ) ;
#835=CARTESIAN_POINT ( 'NONE',  ( -1.158253037810001107, -52.63055504179944677, -23.23212522879996556 ) ) ;
#836=CARTESIAN_POINT ( 'NONE',  ( 18.48933855830000184, -18.50000000000000000, 10.02928721039999971 ) ) ;
#839=ORIENTED_EDGE ( 'NONE', *, *, #4007, .T. ) ;
#845=CARTESIAN_POINT ( 'NONE',  ( -7.243718123969999922, -73.71457659610000235, 39.57993253109999898 ) ) ;
#847=CIRCLE ( 'NONE', #11969, 3.500000000000003109 ) ;
#849=CARTESIAN_POINT ( 'NONE',  ( -21.66710847110000060, -65.28157844300000079, 15.85023555240000093 ) ) ;
#851=B_SPLINE_SURFACE_WITH_KNOTS ( 'NONE', 5, 5, ( 
 ( #9154, #9307, #24622, #7287, #11483, #27396 ),
 ( #27108, #18362, #11342, #26963, #9456, #7147 ),
 ( #20248, #7000, #20389, #758, #9603, #18502 ),
 ( #7444, #315, #4654, #13978, #13830, #13530 ),
 ( #24773, #18061, #4810, #18210, #24919, #11631 ),
 ( #16304, #4949, #22735, #2776, #20541, #613 ) ),
 .UNSPECIFIED., .F., .F., .F.,
 ( 6, 6 ),
 ( 6, 6 ),
 ( 5.157533855050000504, 12.02487295920000143 ),
 ( 0.000000000000000000, 0.5000000000000000000 ),
 .UNSPECIFIED. ) ;
#853=CARTESIAN_POINT ( 'NONE',  ( -12.27142156090000036, -72.55115057349999574, -25.88050564190000102 ) ) ;
#854=CARTESIAN_POINT ( 'NONE',  ( 7.670974394469999957, -34.59820524359999894, -21.21808786259999735 ) ) ;
#858=ORIENTED_EDGE ( 'NONE', *, *, #20790, .T. ) ;
#860=EDGE_LOOP ( 'NONE', ( #15145, #21340, #10745, #11214 ) ) ;
#861=EDGE_CURVE ( 'NONE', #22467, #9596, #19286, .T. ) ;
#862=EDGE_CURVE ( 'NONE', #12242, #19473, #26277, .T. ) ;
#864=AXIS2_PLACEMENT_3D ( 'NONE', #14681, #1447, #3755 ) ;
#865=EDGE_CURVE ( 'NONE', #22913, #452, #1848, .T. ) ;
#868=ADVANCED_FACE ( 'NONE', ( #21197 ), #23938, .T. ) ;
#870=CARTESIAN_POINT ( 'NONE',  ( -20.32218854209832060, -45.95049969750532171, 14.70359657038399170 ) ) ;
#871=ORIENTED_EDGE ( 'NONE', *, *, #18136, .T. ) ;
#873=CARTESIAN_POINT ( 'NONE',  ( 21.87060598609999928, -37.33944922150000423, -8.721288104830000165 ) ) ;
#875=ORIENTED_EDGE ( 'NONE', *, *, #26119, .T. ) ;
#876=CARTESIAN_POINT ( 'NONE',  ( 7.245634850458852583, -74.15297958040834203, -40.25190969039465472 ) ) ;
#879=CARTESIAN_POINT ( 'NONE',  ( -14.59919365920000089, -79.49999999010000806, 36.80099835649999562 ) ) ;
#880=CARTESIAN_POINT ( 'NONE',  ( -1.061008937839999833, -66.63438074019998680, -25.83911337500000016 ) ) ;
#881=FACE_OUTER_BOUND ( 'NONE', #22917, .T. ) ;
#883=CARTESIAN_POINT ( 'NONE',  ( 36.54773082250000016, -74.06528849890000288, -14.18451747229999960 ) ) ;
#885=CARTESIAN_POINT ( 'NONE',  ( 23.41606623399999876, -59.03785532109999679, -0.2656050083209999801 ) ) ;
#886=CARTESIAN_POINT ( 'NONE',  ( -20.94814304569999663, -64.78279493969998271, 14.49686735409999905 ) ) ;
#887=ORIENTED_EDGE ( 'NONE', *, *, #2613, .F. ) ;
#889=CARTESIAN_POINT ( 'NONE',  ( -2.199195337949999995, -18.50000000000000000, -21.72398268019999890 ) ) ;
#890=CARTESIAN_POINT ( 'NONE',  ( 36.58027808493192623, -74.13071341588579344, -14.24617784392711428 ) ) ;
#892=CARTESIAN_POINT ( 'NONE',  ( -12.57512920220000119, -18.50000000000000000, 18.22246578589999899 ) ) ;
#894=CARTESIAN_POINT ( 'NONE',  ( 8.963580768319998171, -35.44265701029999605, -20.01429411819999871 ) ) ;
#896=EDGE_CURVE ( 'NONE', #22615, #26338, #2075, .T. ) ;
#897=CARTESIAN_POINT ( 'NONE',  ( -13.44405788329999929, -68.28990366489999531, 22.97003105929999833 ) ) ;
#898=VERTEX_POINT ( 'NONE', #25850 ) ;
#899=EDGE_CURVE ( 'NONE', #18945, #25813, #27579, .T. ) ;
#903=CARTESIAN_POINT ( 'NONE',  ( -11.09626372079999967, -18.85488200820000060, 18.94417954700000450 ) ) ;
#904=CARTESIAN_POINT ( 'NONE',  ( -11.93805380160000063, -59.03785532109999679, -20.14610571120000060 ) ) ;
#905=FACE_OUTER_BOUND ( 'NONE', #21357, .T. ) ;
#907=EDGE_CURVE ( 'NONE', #16270, #7945, #3697, .T. ) ;
#908=ORIENTED_EDGE ( 'NONE', *, *, #7129, .F. ) ;
#910=ORIENTED_EDGE ( 'NONE', *, *, #10616, .T. ) ;
#911=( GEOMETRIC_REPRESENTATION_CONTEXT ( 3 ) GLOBAL_UNCERTAINTY_ASSIGNED_CONTEXT ( ( #21125 ) ) GLOBAL_UNIT_ASSIGNED_CONTEXT ( ( #27847, #5964, #28255 ) ) REPRESENTATION_CONTEXT ( 'NONE', 'WORKASPACE' ) );
#912=CARTESIAN_POINT ( 'NONE',  ( -11.61449144829999902, -19.46147648009999997, 19.01640067170000137 ) ) ;
#916=CARTESIAN_POINT ( 'NONE',  ( 39.12175830329999826, -73.75838856969998858, 7.250123850439999629 ) ) ;
#917=CARTESIAN_POINT ( 'NONE',  ( -10.51912179628067179, -19.48459656375596083, -21.06649659360595805 ) ) ;
#919=CARTESIAN_POINT ( 'NONE',  ( 26.64667610715658341, -68.06111924181846007, 1.045321110801250342 ) ) ;
#920=CARTESIAN_POINT ( 'NONE',  ( 9.822722921346285219, -62.32592447406135960, -24.20923697715459255 ) ) ;
#921=ORIENTED_EDGE ( 'NONE', *, *, #8543, .F. ) ;
#922=TOROIDAL_SURFACE ( 'NONE', #1351, 3.500000000000000000, 0.5000000000000000000 ) ;
#923=CARTESIAN_POINT ( 'NONE',  ( -32.73892504640000567, -79.66744423050000989, -22.13232332860000184 ) ) ;
#928=CARTESIAN_POINT ( 'NONE',  ( -2.207587960610000177, -80.12576929450000307, 46.98911235669999797 ) ) ;
#929=CARTESIAN_POINT ( 'NONE',  ( 7.687068830730000357, -29.55373640999999907, -21.02495470140000222 ) ) ;
#930=LINE ( 'NONE', #25388, #17766 ) ;
#931=EDGE_LOOP ( 'NONE', ( #13783, #10024, #26286, #1881 ) ) ;
#934=CARTESIAN_POINT ( 'NONE',  ( -18.92959878400000306, -32.71502530480000104, 13.33075250369999942 ) ) ;
#935=SPHERICAL_SURFACE ( 'NONE', #9109, 2.000000494509999616 ) ;
#937=CARTESIAN_POINT ( 'NONE',  ( 22.38224740400000101, -58.97930424469999622, -8.613459702469999257 ) ) ;
#939=CARTESIAN_POINT ( 'NONE',  ( 26.59217027070000228, -67.24447298400001216, 1.343207599729999924 ) ) ;
#944=AXIS2_PLACEMENT_3D ( 'NONE', #27835, #25652, #10173 ) ;
#946=DIRECTION ( 'NONE',  ( 0.000000000000000000, -1.000000000000000000, 0.000000000000000000 ) ) ;
#947=DIRECTION ( 'NONE',  ( -0.000000000000000000, 1.000000000000000000, 0.000000000000000000 ) ) ;
#948=CARTESIAN_POINT ( 'NONE',  ( -7.325370793560000315, -19.50000000000000000, -24.94672208400000102 ) ) ;
#949=CARTESIAN_POINT ( 'NONE',  ( 21.79230281499999933, -37.95144146749999692, -8.472394310150001218 ) ) ;
#952=DIRECTION ( 'NONE',  ( 0.000000000000000000, 0.000000000000000000, -1.000000000000000000 ) ) ;
#953=CARTESIAN_POINT ( 'NONE',  ( 47.16788169050000334, -74.59616887820000386, -1.399136062990000040 ) ) ;
#956=CARTESIAN_POINT ( 'NONE',  ( 40.65853658540000026, -84.50000000000000000, -6.717799458580000049 ) ) ;
#957=CARTESIAN_POINT ( 'NONE',  ( -36.23922253580000330, -74.50000000000000000, -27.04683438039999999 ) ) ;
#960=EDGE_LOOP ( 'NONE', ( #25413, #1869, #2126, #4112 ) ) ;
#961=DIRECTION ( 'NONE',  ( 0.3687499999999825917, 0.000000000000000000, -0.9295286103719523352 ) ) ;
#962=EDGE_CURVE ( 'NONE', #25324, #23580, #23376, .T. ) ;
#966=CARTESIAN_POINT ( 'NONE',  ( -14.24982662769999919, -74.06193868690000670, 36.58417219249999874 ) ) ;
#968=CARTESIAN_POINT ( 'NONE',  ( -2.594576081490000075, -26.05152176759999705, -23.77804158390000211 ) ) ;
#969=CARTESIAN_POINT ( 'NONE',  ( 41.00000000000000000, -84.50000000000000000, -10.20110288159999890 ) ) ;
#970=CIRCLE ( 'NONE', #26038, 7.750000000000000000 ) ;
#972=CARTESIAN_POINT ( 'NONE',  ( 40.70731707320000226, -82.25000000000000000, 7.215414233289999757 ) ) ;
#973=CARTESIAN_POINT ( 'NONE',  ( 22.03392159830000097, -53.29669431010000125, -7.317502146920000783 ) ) ;
#981=DIRECTION ( 'NONE',  ( 1.000000000000000000, 0.000000000000000000, 0.000000000000000000 ) ) ;
#982=CARTESIAN_POINT ( 'NONE',  ( 36.82697894980000086, -80.49999984420000487, -13.57704391360000074 ) ) ;
#985=CARTESIAN_POINT ( 'NONE',  ( -16.49390888960000368, -77.00000000000000000, 44.28897684009999836 ) ) ;
#986=AXIS2_PLACEMENT_3D ( 'NONE', #22602, #25076, #15579 ) ;
#991=ORIENTED_EDGE ( 'NONE', *, *, #7736, .F. ) ;
#993=EDGE_CURVE ( 'NONE', #10427, #13587, #7237, .T. ) ;
#994=CARTESIAN_POINT ( 'NONE',  ( -7.228306055930000085, -73.78142915380000488, 38.95667586449999931 ) ) ;
#996=CARTESIAN_POINT ( 'NONE',  ( 20.30102379280000235, -72.00000000000000000, -30.97095677779999789 ) ) ;
#1000=CARTESIAN_POINT ( 'NONE',  ( 8.118248377169999586, -31.57154383349999804, -20.94291994239999966 ) ) ;
#1001=CARTESIAN_POINT ( 'NONE',  ( 0.000000000000000000, -18.50000000000000000, 0.000000000000000000 ) ) ;
#1005=ORIENTED_EDGE ( 'NONE', *, *, #21842, .F. ) ;
#1006=AXIS2_PLACEMENT_3D ( 'NONE', #8762, #26564, #6605 ) ;
#1008=AXIS2_PLACEMENT_3D ( 'NONE', #14537, #28360, #12892 ) ;
#1010=CARTESIAN_POINT ( 'NONE',  ( -2.487211299430000189, -58.24783479010000065, -24.65535445909999979 ) ) ;
#1014=ORIENTED_EDGE ( 'NONE', *, *, #20847, .T. ) ;
#1016=DIRECTION ( 'NONE',  ( -0.2414462220490755373, 0.000000000000000000, -0.9704142011833033488 ) ) ;
#1018=VERTEX_POINT ( 'NONE', #11526 ) ;
#1022=AXIS2_PLACEMENT_3D ( 'NONE', #25105, #14175, #648 ) ;
#1023=AXIS2_PLACEMENT_3D ( 'NONE', #5325, #23241, #26231 ) ;
#1024=CARTESIAN_POINT ( 'NONE',  ( -14.40567825890000009, -79.99130678609999734, 36.71221731090000873 ) ) ;
#1027=CARTESIAN_POINT ( 'NONE',  ( -0.9701699858879999638, -66.11532834579999474, -25.60589938009999855 ) ) ;
#1028=AXIS2_PLACEMENT_3D ( 'NONE', #28773, #22096, #8961 ) ;
#1030=CARTESIAN_POINT ( 'NONE',  ( -16.27748161719999942, -72.55114741090000052, 23.56761092880000064 ) ) ;
#1031=ORIENTED_EDGE ( 'NONE', *, *, #24472, .F. ) ;
#1032=EDGE_CURVE ( 'NONE', #16440, #21679, #3049, .T. ) ;
#1035=CARTESIAN_POINT ( 'NONE',  ( 25.24156424050000069, -64.93834664010000779, 0.4035716298300000560 ) ) ;
#1036=CARTESIAN_POINT ( 'NONE',  ( 36.26491344080000090, -73.99869055300000298, -14.02738897890000125 ) ) ;
#1038=CARTESIAN_POINT ( 'NONE',  ( 7.347638122930000545E-15, -79.00000000000000000, -40.00000000000000000 ) ) ;
#1039=ADVANCED_FACE ( 'NONE', ( #9787 ), #6268, .T. ) ;
#1040=CARTESIAN_POINT ( 'NONE',  ( -7.288905194729153436, -73.99994620308055460, 39.62752846077490432 ) ) ;
#1042=EDGE_LOOP ( 'NONE', ( #18545, #11786 ) ) ;
#1044=FACE_OUTER_BOUND ( 'NONE', #23374, .T. ) ;
#1046=CARTESIAN_POINT ( 'NONE',  ( 36.71918983540000880, -74.79610922010000706, -14.73254090590000054 ) ) ;
#1049=VECTOR ( 'NONE', #16313, 1000.000000000000000 ) ;
#1053=CARTESIAN_POINT ( 'NONE',  ( 47.25000000000000000, -75.00000000000000000, -1.242228542250000064E-12 ) ) ;
#1055=CARTESIAN_POINT ( 'NONE',  ( -10.70549402610000023, -27.06641747000000109, 19.56133743230000022 ) ) ;
#1061=CARTESIAN_POINT ( 'NONE',  ( 40.03809227200000009, -73.97913911259999509, 7.260235792989999659 ) ) ;
#1062=CARTESIAN_POINT ( 'NONE',  ( -10.64840607053500854, -19.46749811384168893, -19.68096147938357277 ) ) ;
#1063=CARTESIAN_POINT ( 'NONE',  ( 24.98800475346121175, -67.64340390318518814, -8.269946471920237130 ) ) ;
#1065=VECTOR ( 'NONE', #27100, 1000.000000000000000 ) ;
#1066=CARTESIAN_POINT ( 'NONE',  ( 46.77002716385706549, -79.85430130744032340, -3.262371211140790539 ) ) ;
#1068=ADVANCED_FACE ( 'NONE', ( #9500, #27594, #25400, #14021, #7488, #27729 ), #16055, .F. ) ;
#1069=CARTESIAN_POINT ( 'NONE',  ( -32.70203577369999692, -80.13412001289999864, -21.70611439569999845 ) ) ;
#1070=CARTESIAN_POINT ( 'NONE',  ( -41.00000000000000000, -74.50000000000000000, 10.20110288159999890 ) ) ;
#1072=ORIENTED_EDGE ( 'NONE', *, *, #1722, .F. ) ;
#1073=CARTESIAN_POINT ( 'NONE',  ( -3.653527383279999707, -80.06168500389999565, 46.47637748780000067 ) ) ;
#1074=CARTESIAN_POINT ( 'NONE',  ( -13.17060483900000101, -68.28989248250000799, -23.12790341000000183 ) ) ;
#1077=CARTESIAN_POINT ( 'NONE',  ( -6.717799458580000049, -84.00000000000000000, -40.65853658540000026 ) ) ;
#1078=CARTESIAN_POINT ( 'NONE',  ( -19.73214627109999952, -19.39383846099999786, 14.41763749569999931 ) ) ;
#1080=CARTESIAN_POINT ( 'NONE',  ( 29.01006767000000153, -74.25055803479999383, -26.50048742260000267 ) ) ;
#1081=CARTESIAN_POINT ( 'NONE',  ( -14.92146038114265316, -71.38375628612867274, 23.72383756696897450 ) ) ;
#1082=CARTESIAN_POINT ( 'NONE',  ( 26.61464584169999981, -68.28989939179999169, 0.1578490469770000015 ) ) ;
#1086=LINE ( 'NONE', #18838, #1922 ) ;
#1087=CARTESIAN_POINT ( 'NONE',  ( -38.81101221975856674, -73.50000015768027595, -7.152485405736775270 ) ) ;
#1088=CARTESIAN_POINT ( 'NONE',  ( 20.73023592270000037, -36.12634066420000067, -8.988673776420000650 ) ) ;
#1089=DIRECTION ( 'NONE',  ( -0.3447001089730665213, 0.000000000000000000, 0.9387128607161809857 ) ) ;
#1090=ORIENTED_EDGE ( 'NONE', *, *, #9403, .T. ) ;
#1091=CARTESIAN_POINT ( 'NONE',  ( 46.25000000000000000, -74.00000000000000000, -4.582575694960000057 ) ) ;
#1092=CARTESIAN_POINT ( 'NONE',  ( -15.70782602609999756, -68.38632221809999123, 23.02257119289999920 ) ) ;
#1093=FACE_OUTER_BOUND ( 'NONE', #11606, .T. ) ;
#1094=CARTESIAN_POINT ( 'NONE',  ( 6.890073352990000011, -40.75155002679999683, -21.70991749099999879 ) ) ;
#1096=EDGE_LOOP ( 'NONE', ( #26180, #28223, #1259, #7233 ) ) ;
#1097=ADVANCED_FACE ( 'NONE', ( #2970 ), #25823, .T. ) ;
#1098=CARTESIAN_POINT ( 'NONE',  ( -39.84605369636123129, -73.88016183364008782, 7.248366623731184788 ) ) ;
#1099=CARTESIAN_POINT ( 'NONE',  ( 24.39453504989999999, -19.39368411259999903, 1.460252184429999822 ) ) ;
#1102=CARTESIAN_POINT ( 'NONE',  ( 19.92601281039999961, -18.61945110180000285, -8.242644266630000160 ) ) ;
#1106=AXIS2_PLACEMENT_3D ( 'NONE', #6041, #26597, #12868 ) ;
#1107=CARTESIAN_POINT ( 'NONE',  ( -2.573836319060000211, -39.29539198449999304, -24.78771587189999792 ) ) ;
#1109=EDGE_CURVE ( 'NONE', #25360, #10596, #7633, .T. ) ;
#1112=CARTESIAN_POINT ( 'NONE',  ( 21.84994998139999822, -44.93330283399999558, -6.931585813899999948 ) ) ;
#1116=CARTESIAN_POINT ( 'NONE',  ( -32.73892506530000190, -74.45114023669999881, -22.13232332709999994 ) ) ;
#1118=VECTOR ( 'NONE', #7360, 1000.000000000000000 ) ;
#1120=CARTESIAN_POINT ( 'NONE',  ( 20.76917594449999882, -34.61672939740000032, -8.508194273930000051 ) ) ;
#1121=CARTESIAN_POINT ( 'NONE',  ( 7.135467526410000261, -73.50000000000000000, 38.71641004229999794 ) ) ;
#1124=AXIS2_PLACEMENT_3D ( 'NONE', #20115, #24488, #15589 ) ;
#1126=CARTESIAN_POINT ( 'NONE',  ( 20.15266352549999951, -28.56548694950000211, -8.805377537309999170 ) ) ;
#1130=ORIENTED_EDGE ( 'NONE', *, *, #22043, .T. ) ;
#1133=EDGE_CURVE ( 'NONE', #17770, #10479, #13657, .T. ) ;
#1137=AXIS2_PLACEMENT_3D ( 'NONE', #6987, #7132, #23919 ) ;
#1139=DIRECTION ( 'NONE',  ( 1.256627704189999682E-15, 0.000000000000000000, 1.000000000000000000 ) ) ;
#1140=CARTESIAN_POINT ( 'NONE',  ( 25.08083557389999996, -74.00200704200000246, -30.10596417070000186 ) ) ;
#1141=EDGE_CURVE ( 'NONE', #11892, #3141, #15331, .T. ) ;
#1144=PLANE ( 'NONE',  #4134 ) ;
#1146=DIRECTION ( 'NONE',  ( 1.000000000000000000, 0.000000000000000000, 0.000000000000000000 ) ) ;
#1147=ORIENTED_EDGE ( 'NONE', *, *, #17104, .T. ) ;
#1153=CARTESIAN_POINT ( 'NONE',  ( 9.270563563040001398, -37.35781407409999844, -22.45851363030000059 ) ) ;
#1155=ORIENTED_EDGE ( 'NONE', *, *, #25039, .F. ) ;
#1156=B_SPLINE_CURVE_WITH_KNOTS ( 'NONE', 5,
 ( #23277, #12450, #10265, #1421, #25605, #23417 ),
 .UNSPECIFIED., .F., .F.,
 ( 6, 6 ),
 ( 0.000000000000000000, 1.000000000000000000 ),
 .UNSPECIFIED. ) ;
#1161=CARTESIAN_POINT ( 'NONE',  ( 0.000000000000000000, -82.50000000000000000, 0.000000000000000000 ) ) ;
#1162=CARTESIAN_POINT ( 'NONE',  ( 9.009289338599998587, -35.83210504610000413, -20.15582154950000060 ) ) ;
#1164=CARTESIAN_POINT ( 'NONE',  ( -21.99985828019999801, -74.00000000000000000, -31.89935321680000158 ) ) ;
#1165=VERTEX_POINT ( 'NONE', #25529 ) ;
#1168=CARTESIAN_POINT ( 'NONE',  ( 24.90432507590000455, -60.33034294479999460, 1.297259702619999899 ) ) ;
#1169=CARTESIAN_POINT ( 'NONE',  ( -20.31915794119999674, -62.12743832499999996, 12.73748489189999944 ) ) ;
#1172=CARTESIAN_POINT ( 'NONE',  ( 23.93312658989999875, -65.07443093669999712, -7.727579958389999781 ) ) ;
#1173=CARTESIAN_POINT ( 'NONE',  ( -7.258712132442814990, -74.00006796125886410, 39.81159221151552430 ) ) ;
#1175=VERTEX_POINT ( 'NONE', #1628 ) ;
#1176=B_SPLINE_CURVE_WITH_KNOTS ( 'NONE', 3,
 ( #23554, #16856, #14788, #12593, #8521, #3457, #12323, #25746, #6787, #4303, #11276, #20033, #22529, #19876, #28761, #256, #17713 ),
 .UNSPECIFIED., .F., .F.,
 ( 4, 2, 2, 2, 1, 1, 1, 2, 2, 4 ),
 ( 0.000000000000000000, 0.2499999999998541722, 0.3749999999997812861, 0.4374999999997471467, 0.4687499999997326028, 0.4843749999997279954, 0.4921874999997256639, 0.4960937499997272182, 0.4999999999997287725, 1.000000000000000000 ),
 .UNSPECIFIED. ) ;
#1178=CARTESIAN_POINT ( 'NONE',  ( -31.89935321680000158, -74.00000000000000000, -21.99985828019999801 ) ) ;
#1179=CARTESIAN_POINT ( 'NONE',  ( 36.65640604229999866, -79.86805848820000620, -14.39612937579999929 ) ) ;
#1183=ADVANCED_FACE ( 'NONE', ( #3658 ), #21474, .T. ) ;
#1184=VECTOR ( 'NONE', #12556, 1000.000000000000000 ) ;
#1185=CARTESIAN_POINT ( 'NONE',  ( -2.679427010961042299, -80.39259899117686814, 46.73670472467608761 ) ) ;
#1189=ORIENTED_EDGE ( 'NONE', *, *, #11802, .T. ) ;
#1190=VECTOR ( 'NONE', #1655, 1000.000000000000000 ) ;
#1191=CARTESIAN_POINT ( 'NONE',  ( 22.76317971519999972, -52.57401960349999825, 10.17780311019999928 ) ) ;
#1193=EDGE_CURVE ( 'NONE', #6398, #23740, #108, .T. ) ;
#1197=CARTESIAN_POINT ( 'NONE',  ( 38.68350846249999364, -73.93831524339999817, 7.318371247189999984 ) ) ;
#1199=CARTESIAN_POINT ( 'NONE',  ( -11.90443957499999961, -64.24504445130001784, -23.68393584109999850 ) ) ;
#1200=CARTESIAN_POINT ( 'NONE',  ( 47.01215786981062195, -79.64739487177904209, -2.324349206678411939 ) ) ;
#1202=DIRECTION ( 'NONE',  ( 0.000000000000000000, 1.000000000000000000, 0.000000000000000000 ) ) ;
#1203=DIRECTION ( 'NONE',  ( 0.7071067811865470176, 0.000000000000000000, 0.7071067811865480168 ) ) ;
#1207=VECTOR ( 'NONE', #24957, 1000.000000000000000 ) ;
#1214=CARTESIAN_POINT ( 'NONE',  ( 30.21390923379999904, -74.22140788000000100, -25.07573566509999807 ) ) ;
#1215=CARTESIAN_POINT ( 'NONE',  ( -14.49981904734982585, -70.55987052708249507, 23.54264869499610313 ) ) ;
#1217=ORIENTED_EDGE ( 'NONE', *, *, #10543, .T. ) ;
#1218=CARTESIAN_POINT ( 'NONE',  ( 21.39481749499999808, -35.54838723460000693, -7.344946279170000203 ) ) ;
#1219=ADVANCED_FACE ( 'NONE', ( #5396 ), #28141, .T. ) ;
#1225=B_SPLINE_CURVE_WITH_KNOTS ( 'NONE', 5,
 ( #21036, #1092, #5574, #21170, #5707, #20892 ),
 .UNSPECIFIED., .F., .F.,
 ( 6, 6 ),
 ( 0.000000000000000000, 1.000000000000000000 ),
 .UNSPECIFIED. ) ;
#1226=DIRECTION ( 'NONE',  ( 0.09756097560976760563, 0.000000000000000000, 0.9952295494196654602 ) ) ;
#1227=DIRECTION ( 'NONE',  ( -0.7071067811865470176, 0.000000000000000000, 0.7071067811865480168 ) ) ;
#1233=DIRECTION ( 'NONE',  ( 1.000000000000000000, 0.000000000000000000, 0.000000000000000000 ) ) ;
#1236=CARTESIAN_POINT ( 'NONE',  ( -14.04941245390000049, -74.01263034700001242, 36.28249488850000404 ) ) ;
#1241=CARTESIAN_POINT ( 'NONE',  ( 21.75421831149999718, -44.93343662089999668, -7.233371418780000006 ) ) ;
#1243=CARTESIAN_POINT ( 'NONE',  ( -11.04661350269999964, -27.06679042429999882, -19.46499051269999825 ) ) ;
#1244=ORIENTED_EDGE ( 'NONE', *, *, #11232, .T. ) ;
#1245=DIRECTION ( 'NONE',  ( -1.000000000000000000, 0.000000000000000000, 0.000000000000000000 ) ) ;
#1247=ADVANCED_FACE ( 'NONE', ( #16022 ), #20850, .T. ) ;
#1248=VECTOR ( 'NONE', #13164, 1000.000000000000114 ) ;
#1251=CARTESIAN_POINT ( 'NONE',  ( 8.985156090609999424, -35.55399656489999671, -19.52064371570000034 ) ) ;
#1253=LINE ( 'NONE', #23245, #1839 ) ;
#1257=B_SPLINE_SURFACE_WITH_KNOTS ( 'NONE', 5, 5, ( 
 ( #7609, #16473, #20997, #25376, #27970, #8008 ),
 ( #18816, #9618, #23463, #10166, #12229, #27704 ),
 ( #1061, #7743, #9900, #16610, #27411, #19085 ),
 ( #21269, #7463, #3502, #12360, #20857, #25504 ),
 ( #16322, #25233, #916, #23048, #3091, #5539 ),
 ( #9759, #14427, #21140, #1197, #10032, #18946 ) ),
 .UNSPECIFIED., .F., .F., .F.,
 ( 6, 6 ),
 ( 6, 6 ),
 ( 9.300133431499999221E-14, 3.318582255960000005 ),
 ( 0.000000000000000000, 0.5000000000000000000 ),
 .UNSPECIFIED. ) ;
#1259=ORIENTED_EDGE ( 'NONE', *, *, #23716, .F. ) ;
#1260=CARTESIAN_POINT ( 'NONE',  ( 21.56931447779999900, -36.56979901409999911, -6.850353625240000355 ) ) ;
#1261=FACE_OUTER_BOUND ( 'NONE', #13577, .T. ) ;
#1263=CARTESIAN_POINT ( 'NONE',  ( -13.18221367349999973, -68.65989719860000662, -23.31533323539999714 ) ) ;
#1265=B_SPLINE_CURVE_WITH_KNOTS ( 'NONE', 3,
 ( #13229, #2179, #13678, #8853 ),
 .UNSPECIFIED., .F., .F.,
 ( 4, 4 ),
 ( 0.000000000000000000, 1.000000000000000000 ),
 .UNSPECIFIED. ) ;
#1266=DIRECTION ( 'NONE',  ( 1.000000000000000000, 0.000000000000000000, -1.203338504109999799E-16 ) ) ;
#1272=DIRECTION ( 'NONE',  ( 1.000000000000000000, 0.000000000000000000, 0.000000000000000000 ) ) ;
#1276=EDGE_LOOP ( 'NONE', ( #8134, #14105, #8144, #14741 ) ) ;
#1277=DIRECTION ( 'NONE',  ( 1.000000000000000000, 0.000000000000000000, -5.551115123130000643E-17 ) ) ;
#1278=EDGE_CURVE ( 'NONE', #22412, #22777, #20587, .T. ) ;
#1279=EDGE_LOOP ( 'NONE', ( #21889, #21162, #7938, #25017 ) ) ;
#1280=CARTESIAN_POINT ( 'NONE',  ( -14.01337423630000067, -80.50000000000000000, 36.66316738249999929 ) ) ;
#1282=CARTESIAN_POINT ( 'NONE',  ( -19.81272040990000249, -52.63293862069999562, 12.05498172269999912 ) ) ;
#1283=ORIENTED_EDGE ( 'NONE', *, *, #9843, .F. ) ;
#1284=DIRECTION ( 'NONE',  ( 0.4794255386042036160, 0.000000000000000000, 0.8775825618903723147 ) ) ;
#1287=DIRECTION ( 'NONE',  ( -0.4692400087391606633, 0.000000000000000000, 0.8830706733883038062 ) ) ;
#1290=CARTESIAN_POINT ( 'NONE',  ( -17.47679617029999832, -18.50000000000000000, 12.54464522169999796 ) ) ;
#1291=ORIENTED_EDGE ( 'NONE', *, *, #22231, .F. ) ;
#1293=AXIS2_PLACEMENT_3D ( 'NONE', #11079, #4557, #24376 ) ;
#1295=CARTESIAN_POINT ( 'NONE',  ( -32.02433178753376808, -74.00000000000001421, -22.03106757217172884 ) ) ;
#1296=CARTESIAN_POINT ( 'NONE',  ( -21.20809654359999641, -65.04696944340000186, 13.49691729160000087 ) ) ;
#1297=EDGE_CURVE ( 'NONE', #15559, #11794, #14645, .T. ) ;
#1300=CARTESIAN_POINT ( 'NONE',  ( -1.804107087350000027, -18.50000000000000000, -21.15426956649999823 ) ) ;
#1302=ORIENTED_EDGE ( 'NONE', *, *, #17974, .F. ) ;
#1304=TOROIDAL_SURFACE ( 'NONE', #15678, 43.34897771020000334, 20.00000000000000000 ) ;
#1305=CYLINDRICAL_SURFACE ( 'NONE', #864, 0.4999999999999982236 ) ;
#1306=CARTESIAN_POINT ( 'NONE',  ( 37.14416535689999677, -79.97680490119999774, -14.02189532789999937 ) ) ;
#1311=CARTESIAN_POINT ( 'NONE',  ( -9.356041104380000917, -84.50000000000000000, -37.60355029590000697 ) ) ;
#1313=CIRCLE ( 'NONE', #17574, 11.00000000000000000 ) ;
#1315=CARTESIAN_POINT ( 'NONE',  ( 46.50724168351928967, -73.67599622268748760, -3.197465198608631987 ) ) ;
#1316=ORIENTED_EDGE ( 'NONE', *, *, #18744, .F. ) ;
#1319=ORIENTED_EDGE ( 'NONE', *, *, #10244, .F. ) ;
#1321=DIRECTION ( 'NONE',  ( 0.000000000000000000, -1.000000000000000000, 0.000000000000000000 ) ) ;
#1322=B_SPLINE_CURVE_WITH_KNOTS ( 'NONE', 3,
 ( #23215, #18848, #20749, #25270, #16205, #16643 ),
 .UNSPECIFIED., .F., .F.,
 ( 4, 2, 4 ),
 ( 0.000000000000000000, 0.5000000000000000000, 1.000000000000000000 ),
 .UNSPECIFIED. ) ;
#1325=CARTESIAN_POINT ( 'NONE',  ( 9.027382853569999810, -36.23976085289999816, -21.24216557319999765 ) ) ;
#1326=DIRECTION ( 'NONE',  ( 0.000000000000000000, 1.000000000000000000, 0.000000000000000000 ) ) ;
#1327=CARTESIAN_POINT ( 'NONE',  ( 9.993770587066137523, -63.70931641282978575, -24.60213562706236345 ) ) ;
#1331=EDGE_CURVE ( 'NONE', #15974, #19973, #5320, .T. ) ;
#1333=CARTESIAN_POINT ( 'NONE',  ( -2.579354798150000239, -53.77454410920000072, -25.14349222919999960 ) ) ;
#1334=CARTESIAN_POINT ( 'NONE',  ( -2.180054726419999866, -80.20928067410000040, 46.97828202600000225 ) ) ;
#1340=DIRECTION ( 'NONE',  ( 0.000000000000000000, 1.000000000000000000, 0.000000000000000000 ) ) ;
#1343=ADVANCED_FACE ( 'NONE', ( #6078 ), #19840, .T. ) ;
#1345=ORIENTED_EDGE ( 'NONE', *, *, #4475, .F. ) ;
#1346=CARTESIAN_POINT ( 'NONE',  ( 20.95510899789999826, -35.33620304099999743, -8.408939718540000996 ) ) ;
#1347=CARTESIAN_POINT ( 'NONE',  ( 20.41714882420000166, -35.80913068420000656, -8.862965437090000620 ) ) ;
#1349=VERTEX_POINT ( 'NONE', #16743 ) ;
#1351=AXIS2_PLACEMENT_3D ( 'NONE', #26615, #26327, #12885 ) ;
#1355=CARTESIAN_POINT ( 'NONE',  ( 7.482057485060000346, -36.56833510180000246, -21.43629755389999758 ) ) ;
#1361=CARTESIAN_POINT ( 'NONE',  ( 25.88476489150000148, -71.55793241529998738, 11.20710331009999905 ) ) ;
#1364=CARTESIAN_POINT ( 'NONE',  ( 20.47461295229999934, -19.46889316100000045, -8.153555280290001761 ) ) ;
#1365=ADVANCED_FACE ( 'NONE', ( #10434 ), #14955, .T. ) ;
#1367=CARTESIAN_POINT ( 'NONE',  ( -14.65665286289999969, -74.43375220249998847, 36.94583910070000599 ) ) ;
#1368=CARTESIAN_POINT ( 'NONE',  ( 46.25000000000000000, -74.00000000000000000, -9.166287847479999584 ) ) ;
#1375=CARTESIAN_POINT ( 'NONE',  ( 7.452486935440000515, -63.63835192340000191, -23.33420648839999956 ) ) ;
#1376=CARTESIAN_POINT ( 'NONE',  ( -39.69297836749999675, -73.74954830059999722, -7.260231713199999604 ) ) ;
#1378=FACE_OUTER_BOUND ( 'NONE', #27136, .T. ) ;
#1379=CARTESIAN_POINT ( 'NONE',  ( 40.65508461000000295, -75.00000000000000000, -13.75000000000000000 ) ) ;
#1388=DIRECTION ( 'NONE',  ( 1.000000000000000000, 0.000000000000000000, 0.000000000000000000 ) ) ;
#1395=DIRECTION ( 'NONE',  ( 0.000000000000000000, 1.000000000000000000, 0.000000000000000000 ) ) ;
#1397=ORIENTED_EDGE ( 'NONE', *, *, #8218, .F. ) ;
#1398=DIRECTION ( 'NONE',  ( 0.000000000000000000, -1.000000000000000000, 0.000000000000000000 ) ) ;
#1400=AXIS2_PLACEMENT_3D ( 'NONE', #15830, #25329, #20664 ) ;
#1404=CARTESIAN_POINT ( 'NONE',  ( 41.00000000000000000, -74.00000000000000000, 10.20110288159999890 ) ) ;
#1405=CARTESIAN_POINT ( 'NONE',  ( 25.07614445930000002, -74.11216212930001745, -30.15806252000000143 ) ) ;
#1407=CARTESIAN_POINT ( 'NONE',  ( -22.88338618799999935, -72.19388347460001398, 16.81479657839999931 ) ) ;
#1411=CARTESIAN_POINT ( 'NONE',  ( -13.49020432579999884, -18.50000000000000000, 18.73880173299999896 ) ) ;
#1413=EDGE_CURVE ( 'NONE', #19124, #14119, #21633, .T. ) ;
#1414=CARTESIAN_POINT ( 'NONE',  ( 9.463625755926194927, -35.99991740498153092, -20.02750111241616437 ) ) ;
#1416=VECTOR ( 'NONE', #19385, 1000.000000000000000 ) ;
#1418=CARTESIAN_POINT ( 'NONE',  ( -1.172419020520000021, -61.85641277710000452, -23.98846277950000072 ) ) ;
#1419=CARTESIAN_POINT ( 'NONE',  ( 9.497542575549999810, -37.06806481049999746, -22.65555190710000133 ) ) ;
#1420=DIRECTION ( 'NONE',  ( 0.09756097560976760563, 0.000000000000000000, 0.9952295494196654602 ) ) ;
#1421=CARTESIAN_POINT ( 'NONE',  ( 20.52569424150000188, -35.38531346950000511, -8.770435587459999738 ) ) ;
#1422=ORIENTED_EDGE ( 'NONE', *, *, #9345, .F. ) ;
#1423=CARTESIAN_POINT ( 'NONE',  ( 21.51138255720000103, -35.67530038919999669, -6.929578944110000194 ) ) ;
#1425=CARTESIAN_POINT ( 'NONE',  ( 25.26718046270000073, -19.50000000000000000, 6.129403842640000377 ) ) ;
#1426=CARTESIAN_POINT ( 'NONE',  ( 9.061401562000000354, -35.89920192559999634, -20.19233861389999873 ) ) ;
#1427=CARTESIAN_POINT ( 'NONE',  ( -4.459621975350000156, -72.00000000000000000, -28.73485931899999812 ) ) ;
#1430=AXIS2_PLACEMENT_3D ( 'NONE', #3345, #20696, #14129 ) ;
#1431=CARTESIAN_POINT ( 'NONE',  ( -22.19637807654410366, -74.23987217703098906, -32.69975610228092933 ) ) ;
#1435=CIRCLE ( 'NONE', #21428, 1.000000000000000888 ) ;
#1436=DIRECTION ( 'NONE',  ( 0.000000000000000000, 1.000000000000000000, 0.000000000000000000 ) ) ;
#1440=B_SPLINE_CURVE_WITH_KNOTS ( 'NONE', 3,
 ( #6733, #19970, #24055, #15598 ),
 .UNSPECIFIED., .F., .F.,
 ( 4, 4 ),
 ( -6.855861996829999860, 0.000000000000000000 ),
 .UNSPECIFIED. ) ;
#1442=CARTESIAN_POINT ( 'NONE',  ( -2.021043494270000185, -18.61827554290000108, -21.98709576639999952 ) ) ;
#1444=ORIENTED_EDGE ( 'NONE', *, *, #27666, .F. ) ;
#1445=ADVANCED_FACE ( 'NONE', ( #15233 ), #10997, .F. ) ;
#1447=DIRECTION ( 'NONE',  ( -0.7071067811865475727, 0.000000000000000000, 0.7071067811865475727 ) ) ;
#1448=CARTESIAN_POINT ( 'NONE',  ( 36.93448770119999836, -79.95108530920001044, -14.10799736659999937 ) ) ;
#1452=CARTESIAN_POINT ( 'NONE',  ( -2.671186077582594631, -80.39081555798996703, 46.73997660184883784 ) ) ;
#1453=AXIS2_PLACEMENT_3D ( 'NONE', #10854, #6519, #15376 ) ;
#1460=FACE_OUTER_BOUND ( 'NONE', #5969, .T. ) ;
#1461=ORIENTED_EDGE ( 'NONE', *, *, #16424, .F. ) ;
#1463=CARTESIAN_POINT ( 'NONE',  ( 0.000000000000000000, -65.07443093669999712, 0.000000000000000000 ) ) ;
#1465=CARTESIAN_POINT ( 'NONE',  ( 9.885503724449998586, -36.00000000000000000, -20.33566493500000050 ) ) ;
#1467=CARTESIAN_POINT ( 'NONE',  ( -3.807886452449999570, -80.00000000000000000, 46.75000000000000000 ) ) ;
#1468=EDGE_LOOP ( 'NONE', ( #2304, #3722, #15574, #8835 ) ) ;
#1469=DIRECTION ( 'NONE',  ( 0.000000000000000000, 1.000000000000000000, 0.000000000000000000 ) ) ;
#1474=CARTESIAN_POINT ( 'NONE',  ( -0.8459307125330000066, -55.05548131569999981, -23.26322409530000002 ) ) ;
#1475=AXIS2_PLACEMENT_3D ( 'NONE', #5724, #19825, #15149 ) ;
#1476=CARTESIAN_POINT ( 'NONE',  ( -1.501869189730000054, -79.88809860310000488, 47.16627303149999761 ) ) ;
#1477=CARTESIAN_POINT ( 'NONE',  ( -2.578307999469999778, -52.56313962710000709, -25.11373953509999879 ) ) ;
#1483=CARTESIAN_POINT ( 'NONE',  ( 28.89564796280000181, -73.80968813319999811, -26.61317346570000097 ) ) ;
#1484=CARTESIAN_POINT ( 'NONE',  ( -15.78701020529999965, -72.82938648530000592, 23.94860758700000147 ) ) ;
#1486=B_SPLINE_SURFACE_WITH_KNOTS ( 'NONE', 5, 5, ( 
 ( #7989, #6067, #28222, #14410, #12758, #5658 ),
 ( #10149, #16596, #21390, #5799, #23854, #14682 ),
 ( #3895, #21669, #23574, #12620, #16882, #1719 ),
 ( #23299, #10559, #14539, #5522, #19070, #12211 ),
 ( #5927, #21122, #1179, #8126, #3617, #12476 ),
 ( #19345, #1448, #23447, #17016, #10018, #21531 ),
 ( #1306, #18932, #14811, #7853, #16736, #23713 ),
 ( #3756, #17151, #25629, #28787, #10850, #28506 ),
 ( #28362, #23996, #8393, #24142, #1865, #2011 ) ),
 .UNSPECIFIED., .F., .F., .F.,
 ( 6, 3, 6 ),
 ( 6, 6 ),
 ( 4.463004670310000144, 6.097538245950000046, 7.424416524390000660 ),
 ( 0.000000000000000000, 0.5000000000000000000 ),
 .UNSPECIFIED. ) ;
#1490=CARTESIAN_POINT ( 'NONE',  ( 21.47791254800000260, -36.56811099849999636, -7.356933688149999817 ) ) ;
#1491=ORIENTED_EDGE ( 'NONE', *, *, #7558, .T. ) ;
#1492=ADVANCED_FACE ( 'NONE', ( #12008 ), #27763, .T. ) ;
#1493=CARTESIAN_POINT ( 'NONE',  ( 21.47791242350000118, -36.56811125149999953, -7.356933663620000452 ) ) ;
#1495=ORIENTED_EDGE ( 'NONE', *, *, #6337, .T. ) ;
#1499=ORIENTED_EDGE ( 'NONE', *, *, #10277, .F. ) ;
#1501=B_SPLINE_CURVE_WITH_KNOTS ( 'NONE', 3,
 ( #14967, #8273, #19495, #21410, #23733, #3777, #2029, #1467 ),
 .UNSPECIFIED., .F., .F.,
 ( 4, 2, 2, 4 ),
 ( 0.000000000000000000, 0.4999999999999997780, 0.7499999999999998890, 1.000000000000000000 ),
 .UNSPECIFIED. ) ;
#1502=CARTESIAN_POINT ( 'NONE',  ( 9.486381418089997908, -49.04525650320000807, -23.29174250550000025 ) ) ;
#1504=ORIENTED_EDGE ( 'NONE', *, *, #6819, .F. ) ;
#1509=CARTESIAN_POINT ( 'NONE',  ( 20.14564099000000041, -18.61853073029999805, -7.938153854090000294 ) ) ;
#1510=CARTESIAN_POINT ( 'NONE',  ( -14.76202981470000175, -74.22231530550000400, 36.28478801819999688 ) ) ;
#1512=DIRECTION ( 'NONE',  ( 0.000000000000000000, 1.000000000000000000, 0.000000000000000000 ) ) ;
#1515=CARTESIAN_POINT ( 'NONE',  ( 7.150868990479999354, -60.60240929710000302, -22.51513940059999896 ) ) ;
#1516=CARTESIAN_POINT ( 'NONE',  ( 7.627566167509999495, -74.00000000000000000, -38.62788938250000115 ) ) ;
#1517=CARTESIAN_POINT ( 'NONE',  ( 20.85556312030000115, -57.91337896769999816, 10.70610008499999921 ) ) ;
#1518=PLANE ( 'NONE',  #7141 ) ;
#1523=EDGE_CURVE ( 'NONE', #10585, #11090, #26766, .T. ) ;
#1527=CARTESIAN_POINT ( 'NONE',  ( 34.89999999999999858, -84.50000000000000000, 4.273876174839999917E-15 ) ) ;
#1529=EDGE_CURVE ( 'NONE', #23252, #17228, #8426, .T. ) ;
#1530=CARTESIAN_POINT ( 'NONE',  ( -7.196178079599999222, -73.81415926540000783, -38.70548889989999708 ) ) ;
#1538=CONICAL_SURFACE ( 'NONE', #624, 25.14975229270001833, 0.4276056667390000787 ) ;
#1539=ADVANCED_FACE ( 'NONE', ( #21064 ), #9057, .T. ) ;
#1542=CARTESIAN_POINT ( 'NONE',  ( -11.25859204269364078, -19.46519122827088566, 19.08718618545535861 ) ) ;
#1545=CARTESIAN_POINT ( 'NONE',  ( 27.75394116159999669, -74.50000000000000000, -27.75394116159999669 ) ) ;
#1546=CARTESIAN_POINT ( 'NONE',  ( -22.41375146320000056, -69.63326797740000984, 15.46718870090000131 ) ) ;
#1549=DIRECTION ( 'NONE',  ( 0.000000000000000000, 0.000000000000000000, -1.000000000000000000 ) ) ;
#1550=DIRECTION ( 'NONE',  ( 1.000000000000000000, 0.000000000000000000, 0.000000000000000000 ) ) ;
#1551=CARTESIAN_POINT ( 'NONE',  ( 7.044629870050000520, -36.15937179259999823, -21.49951968199999897 ) ) ;
#1553=ORIENTED_EDGE ( 'NONE', *, *, #13410, .T. ) ;
#1554=DIRECTION ( 'NONE',  ( -0.9952295494196655712, 0.000000000000000000, -0.09756097560976655092 ) ) ;
#1556=ORIENTED_EDGE ( 'NONE', *, *, #10088, .F. ) ;
#1557=AXIS2_PLACEMENT_3D ( 'NONE', #12996, #1958, #1287 ) ;
#1558=ORIENTED_EDGE ( 'NONE', *, *, #9808, .F. ) ;
#1560=CARTESIAN_POINT ( 'NONE',  ( 10.41102187780000143, -36.06096454729999579, -21.78369632219999730 ) ) ;
#1562=DIRECTION ( 'NONE',  ( 0.000000000000000000, -1.000000000000000000, 0.000000000000000000 ) ) ;
#1566=ORIENTED_EDGE ( 'NONE', *, *, #11570, .T. ) ;
#1568=CARTESIAN_POINT ( 'NONE',  ( 21.31951852150000093, -34.95415007660000128, -7.429758059829999262 ) ) ;
#1569=VERTEX_POINT ( 'NONE', #9962 ) ;
#1570=CARTESIAN_POINT ( 'NONE',  ( 11.31764174110000098, -38.00000000000000000, -22.43277175240000076 ) ) ;
#1571=EDGE_CURVE ( 'NONE', #1349, #23532, #266, .T. ) ;
#1572=B_SPLINE_CURVE_WITH_KNOTS ( 'NONE', 3,
 ( #2936, #15721, #4666, #5811, #27560, #14690 ),
 .UNSPECIFIED., .F., .F.,
 ( 4, 2, 4 ),
 ( 0.000000000000000000, 0.5000000000000000000, 1.000000000000000000 ),
 .UNSPECIFIED. ) ;
#1574=CARTESIAN_POINT ( 'NONE',  ( -22.13204528394974346, -74.08924643999768023, -32.43483521824870053 ) ) ;
#1575=CARTESIAN_POINT ( 'NONE',  ( 21.85035090750000109, -18.50000000000000000, 8.503095831829998730 ) ) ;
#1576=CARTESIAN_POINT ( 'NONE',  ( -32.64229262974771473, -74.19321449783478784, -22.18246179812063090 ) ) ;
#1577=CARTESIAN_POINT ( 'NONE',  ( -20.58900368409999970, -58.81362829640000456, 14.87320149399999991 ) ) ;
#1581=CARTESIAN_POINT ( 'NONE',  ( -0.5753802177429999665, -18.61794786970000359, -21.64101937650000096 ) ) ;
#1583=ORIENTED_EDGE ( 'NONE', *, *, #25734, .F. ) ;
#1585=TOROIDAL_SURFACE ( 'NONE', #2055, 21.03431122519999974, 1.000000000000000000 ) ;
#1586=CARTESIAN_POINT ( 'NONE',  ( 10.34250236315985028, -65.75540811119959983, -25.31863394739911399 ) ) ;
#1587=CARTESIAN_POINT ( 'NONE',  ( -5.329070518200000398E-15, -19.46510050329999686, 0.000000000000000000 ) ) ;
#1590=AXIS2_PLACEMENT_3D ( 'NONE', #2444, #11741, #28782 ) ;
#1591=ORIENTED_EDGE ( 'NONE', *, *, #15954, .F. ) ;
#1594=CARTESIAN_POINT ( 'NONE',  ( 47.25009368219999573, -74.76204734789999407, -0.5461026333709999570 ) ) ;
#1596=CARTESIAN_POINT ( 'NONE',  ( 21.08559791560000107, -57.47122622300000216, 10.49905601410000067 ) ) ;
#1598=CARTESIAN_POINT ( 'NONE',  ( 1.421085471519999843E-14, -69.00000000000000000, 46.75000000000000000 ) ) ;
#1601=CARTESIAN_POINT ( 'NONE',  ( 41.00000000000000000, -84.00000000000000000, -10.20110288159999890 ) ) ;
#1602=EDGE_CURVE ( 'NONE', #4968, #212, #2098, .T. ) ;
#1604=CARTESIAN_POINT ( 'NONE',  ( -22.43272078519999724, -80.50000000000000000, -32.20769377289999369 ) ) ;
#1606=CARTESIAN_POINT ( 'NONE',  ( -0.5590517731190000061, -18.50000000000000000, -21.02688049580000040 ) ) ;
#1607=ORIENTED_EDGE ( 'NONE', *, *, #22080, .T. ) ;
#1612=VERTEX_POINT ( 'NONE', #20289 ) ;
#1613=VECTOR ( 'NONE', #24837, 1000.000000000000000 ) ;
#1614=CARTESIAN_POINT ( 'NONE',  ( 10.81555269790697871, -72.52478263476059794, -26.82924833248659624 ) ) ;
#1615=CARTESIAN_POINT ( 'NONE',  ( -19.73459502929999587, -19.18584080579999807, 14.41863472910000077 ) ) ;
#1617=DIRECTION ( 'NONE',  ( 0.3687499999999814260, 0.000000000000000000, -0.9295286103719527793 ) ) ;
#1619=CARTESIAN_POINT ( 'NONE',  ( -18.87406717280000024, -19.42987840520000020, 13.82478526419999909 ) ) ;
#1622=CARTESIAN_POINT ( 'NONE',  ( 27.75394116159999669, -74.50000000000000000, -27.75394116159999669 ) ) ;
#1624=VECTOR ( 'NONE', #20003, 1000.000000000000114 ) ;
#1627=CARTESIAN_POINT ( 'NONE',  ( 36.24656994149999889, -82.25000000000000000, -15.05817610060000078 ) ) ;
#1628=CARTESIAN_POINT ( 'NONE',  ( -38.08875739639999836, -74.50000000000000000, -9.476764215410000247 ) ) ;
#1630=CARTESIAN_POINT ( 'NONE',  ( 21.54829813079999923, -37.62468161500000008, -7.859468734160000025 ) ) ;
#1631=CARTESIAN_POINT ( 'NONE',  ( 9.323408666494477970, -35.97776767532982234, -19.72111573045538790 ) ) ;
#1633=EDGE_CURVE ( 'NONE', #14431, #13203, #23844, .T. ) ;
#1636=B_SPLINE_CURVE_WITH_KNOTS ( 'NONE', 3,
 ( #8884, #8309, #22760, #7311, #782, #9037, #11212, #5125, #4677, #486, #634, #336, #9482, #13406, #24493, #2356, #20724, #26984, #9179, #9624 ),
 .UNSPECIFIED., .F., .F.,
 ( 4, 2, 2, 1, 1, 1, 1, 1, 1, 2, 2, 2, 4 ),
 ( 0.000000000000000000, 0.2499999999997837841, 0.3749999999996731503, 0.4374999999996190270, 0.4687499999995919375, 0.4843749999995772271, 0.4921874999995687339, 0.4960937499995645705, 0.4980468749995613509, 0.4990234374995608513, 0.4999999999995603517, 0.7499999999997800648, 1.000000000000000000 ),
 .UNSPECIFIED. ) ;
#1638=ORIENTED_EDGE ( 'NONE', *, *, #14608, .T. ) ;
#1639=AXIS2_PLACEMENT_3D ( 'NONE', #14487, #7674, #5464 ) ;
#1641=CARTESIAN_POINT ( 'NONE',  ( 20.76917537309745043, -34.61672842233151215, -8.508194708340036883 ) ) ;
#1643=ORIENTED_EDGE ( 'NONE', *, *, #23439, .F. ) ;
#1646=CARTESIAN_POINT ( 'NONE',  ( 25.35362416179999911, -70.54208558190001099, 11.30155583190000002 ) ) ;
#1650=DIRECTION ( 'NONE',  ( 0.000000000000000000, 1.000000000000000000, 0.000000000000000000 ) ) ;
#1651=CARTESIAN_POINT ( 'NONE',  ( -14.03661932880000052, -74.01263034700001242, 36.31171197689999985 ) ) ;
#1652=LINE ( 'NONE', #10076, #25553 ) ;
#1655=DIRECTION ( 'NONE',  ( -1.000000000000000000, 0.000000000000000000, 0.000000000000000000 ) ) ;
#1657=CARTESIAN_POINT ( 'NONE',  ( 9.133379025440000021, -64.81170986960000846, -23.88371660259999985 ) ) ;
#1659=CARTESIAN_POINT ( 'NONE',  ( 20.71609666450000020, -58.79428935229999098, 10.97841134070000102 ) ) ;
#1660=CARTESIAN_POINT ( 'NONE',  ( -11.05584978989999989, -26.99662418170000322, -22.00022356550000069 ) ) ;
#1661=ORIENTED_EDGE ( 'NONE', *, *, #15036, .F. ) ;
#1666=CARTESIAN_POINT ( 'NONE',  ( 21.76289735059999941, -18.50000000000000000, 1.487608604080000063 ) ) ;
#1667=CARTESIAN_POINT ( 'NONE',  ( 5.326862811529999898E-15, -69.50000000000000000, -32.75000000000000000 ) ) ;
#1670=CARTESIAN_POINT ( 'NONE',  ( 20.26062886849999956, -31.59895360039999801, -8.804563333769998223 ) ) ;
#1674=CARTESIAN_POINT ( 'NONE',  ( 7.670973119660000172, -34.59820496239999699, -21.21808926809999818 ) ) ;
#1680=DIRECTION ( 'NONE',  ( 1.000000000000000000, 0.000000000000000000, 0.000000000000000000 ) ) ;
#1682=CARTESIAN_POINT ( 'NONE',  ( -22.52719173530000063, -71.34739024110000116, 17.13464880949999980 ) ) ;
#1683=EDGE_CURVE ( 'NONE', #16368, #27297, #20268, .T. ) ;
#1685=CARTESIAN_POINT ( 'NONE',  ( -12.89904887990000049, -65.07443093669999712, -21.58991473350000234 ) ) ;
#1686=CARTESIAN_POINT ( 'NONE',  ( 7.248976484529999098, -36.19499434569999607, -21.47059228039999823 ) ) ;
#1689=EDGE_LOOP ( 'NONE', ( #7473, #20189, #20911 ) ) ;
#1691=VERTEX_POINT ( 'NONE', #20747 ) ;
#1692=CARTESIAN_POINT ( 'NONE',  ( 21.46129390369999967, -36.00000000000000000, -10.95532196250000112 ) ) ;
#1695=CARTESIAN_POINT ( 'NONE',  ( 7.253824468913529167, -36.56890885699328209, -21.48302338317096272 ) ) ;
#1697=CARTESIAN_POINT ( 'NONE',  ( 19.97576656849999921, -72.00000000000000000, -19.97576656849999921 ) ) ;
#1698=CARTESIAN_POINT ( 'NONE',  ( -19.65068252670001669, -52.63280639840017017, 12.32128691209999971 ) ) ;
#1701=DIRECTION ( 'NONE',  ( 1.000000000000000000, 0.000000000000000000, 0.000000000000000000 ) ) ;
#1702=DIRECTION ( 'NONE',  ( -0.9952295494196654602, 0.000000000000000000, 0.09756097560976770278 ) ) ;
#1703=ORIENTED_EDGE ( 'NONE', *, *, #11122, .T. ) ;
#1705=ORIENTED_EDGE ( 'NONE', *, *, #7502, .F. ) ;
#1706=CARTESIAN_POINT ( 'NONE',  ( 39.48500436340665232, -74.13942000237629770, 7.435977657333745938 ) ) ;
#1709=CARTESIAN_POINT ( 'NONE',  ( -19.68101754359999944, -59.01563984649999384, 13.03622722340000095 ) ) ;
#1716=EDGE_CURVE ( 'NONE', #21012, #3837, #1830, .T. ) ;
#1718=CARTESIAN_POINT ( 'NONE',  ( -32.46211842109999424, -74.14773635299999910, -21.81756538839999848 ) ) ;
#1719=CARTESIAN_POINT ( 'NONE',  ( 36.27185351749999853, -79.54415414250000538, -14.99731109350000047 ) ) ;
#1722=EDGE_CURVE ( 'NONE', #27046, #26262, #25796, .T. ) ;
#1724=CARTESIAN_POINT ( 'NONE',  ( -1.738885961541629666, -80.13325245167779087, 47.03841520617770300 ) ) ;
#1727=EDGE_LOOP ( 'NONE', ( #27654, #27698, #9884 ) ) ;
#1728=CARTESIAN_POINT ( 'NONE',  ( 20.64374438970000014, -57.47815920199999340, 10.93952083480000148 ) ) ;
#1729=CARTESIAN_POINT ( 'NONE',  ( -10.20110288159999890, -74.50000000000000000, -41.00000000000000000 ) ) ;
#1730=ORIENTED_EDGE ( 'NONE', *, *, #25632, .T. ) ;
#1734=CARTESIAN_POINT ( 'NONE',  ( 22.48186363828591894, -37.98173178126330640, -9.189959888866203741 ) ) ;
#1735=CARTESIAN_POINT ( 'NONE',  ( -11.62178420722295691, -60.93032377504753327, -22.92104515723715608 ) ) ;
#1738=FACE_OUTER_BOUND ( 'NONE', #12011, .T. ) ;
#1740=DIRECTION ( 'NONE',  ( -0.5439177849611204207, 0.000000000000000000, 0.8391385125251898947 ) ) ;
#1744=FACE_OUTER_BOUND ( 'NONE', #12394, .T. ) ;
#1745=EDGE_LOOP ( 'NONE', ( #28367, #3983, #28795, #25857, #18074, #16586 ) ) ;
#1748=CARTESIAN_POINT ( 'NONE',  ( 8.677144207910000517, -37.95796631070000160, -21.92880662259999980 ) ) ;
#1749=CARTESIAN_POINT ( 'NONE',  ( 38.71641001238787538, -73.63089972761061119, 7.135467692469591228 ) ) ;
#1756=DIRECTION ( 'NONE',  ( 0.3687499999999825917, 0.000000000000000000, -0.9295286103719523352 ) ) ;
#1758=B_SPLINE_CURVE_WITH_KNOTS ( 'NONE', 3,
 ( #21021, #28254, #17188, #26076, #23337, #25524, #6108, #3384, #14982, #1215, #1081, #10050, #18964 ),
 .UNSPECIFIED., .F., .F.,
 ( 4, 2, 1, 1, 1, 2, 2, 4 ),
 ( 0.000000000000000000, 0.2500000000000480171, 0.3750000000000684452, 0.4375000000000789369, 0.4687500000000875411, 0.4843750000000882627, 0.5000000000000889289, 1.000000000000000000 ),
 .UNSPECIFIED. ) ;
#1759=CARTESIAN_POINT ( 'NONE',  ( 20.08451038129999944, -35.57151704429999484, -8.961080048699999523 ) ) ;
#1761=CARTESIAN_POINT ( 'NONE',  ( 21.38844997820000060, -36.30219044460000077, -7.879643458169998560 ) ) ;
#1762=CARTESIAN_POINT ( 'NONE',  ( 9.405437324544319466, -35.99659153760200780, -19.87545419078008635 ) ) ;
#1772=ORIENTED_EDGE ( 'NONE', *, *, #19405, .T. ) ;
#1775=CARTESIAN_POINT ( 'NONE',  ( 22.29336127690000069, -27.06642317520000063, -0.5094344447499999928 ) ) ;
#1776=CARTESIAN_POINT ( 'NONE',  ( 24.56539770530000055, -65.28594186049998882, 10.83220590859999888 ) ) ;
#1779=CARTESIAN_POINT ( 'NONE',  ( 25.26718046270000073, -19.50000000000000000, 6.129403842640000377 ) ) ;
#1780=CARTESIAN_POINT ( 'NONE',  ( 46.25000000000000000, -75.00000000000000000, -14.75000000000000000 ) ) ;
#1781=DIRECTION ( 'NONE',  ( 1.000000000000000000, 0.000000000000000000, 0.000000000000000000 ) ) ;
#1782=CARTESIAN_POINT ( 'NONE',  ( -10.20110288159999890, -84.50000000000000000, 41.00000000000000000 ) ) ;
#1783=ORIENTED_EDGE ( 'NONE', *, *, #3085, .F. ) ;
#1785=DIRECTION ( 'NONE',  ( 0.000000000000000000, -1.000000000000000000, 0.000000000000000000 ) ) ;
#1788=CARTESIAN_POINT ( 'NONE',  ( 10.08508133319999978, -64.24504434620000382, -24.78974410990000266 ) ) ;
#1790=CARTESIAN_POINT ( 'NONE',  ( -7.135467526410000261, -73.50000000000000000, -38.71641004229999794 ) ) ;
#1808=( LENGTH_UNIT ( ) NAMED_UNIT ( * ) SI_UNIT ( .MILLI., .METRE. ) );
#1813=CARTESIAN_POINT ( 'NONE',  ( -38.08875739639999836, -84.00000000000000000, -9.476764215410000247 ) ) ;
#1814=CARTESIAN_POINT ( 'NONE',  ( -38.62788938250000115, -74.00000000000000000, -7.627566167509999495 ) ) ;
#1816=CARTESIAN_POINT ( 'NONE',  ( 24.78974732560000405, -64.24504771300000527, -10.08508462690000052 ) ) ;
#1817=EDGE_LOOP ( 'NONE', ( #741, #20053, #4243, #19995 ) ) ;
#1818=DIRECTION ( 'NONE',  ( -0.5301416321220535632, 0.000000000000000000, -0.8479091047340895360 ) ) ;
#1823=AXIS2_PLACEMENT_3D ( 'NONE', #14152, #18674, #23052 ) ;
#1826=CARTESIAN_POINT ( 'NONE',  ( -18.60622341941390800, -19.47370675684462427, 13.24439685365035757 ) ) ;
#1827=CARTESIAN_POINT ( 'NONE',  ( 7.356933014059999998, -36.56811127230000125, -21.47791253540000156 ) ) ;
#1828=DIRECTION ( 'NONE',  ( 1.000000000000000000, 0.000000000000000000, 0.000000000000000000 ) ) ;
#1829=ORIENTED_EDGE ( 'NONE', *, *, #7541, .F. ) ;
#1830=B_SPLINE_CURVE_WITH_KNOTS ( 'NONE', 5,
 ( #7638, #953, #18842, #18258, #21168, #9645, #7194, #14027, #1091 ),
 .UNSPECIFIED., .F., .F.,
 ( 6, 3, 6 ),
 ( 0.000000000000000000, 0.3540406197649746955, 1.000000000000000000 ),
 .UNSPECIFIED. ) ;
#1832=CARTESIAN_POINT ( 'NONE',  ( 36.50549972520000352, -74.62369755570000507, -14.71598444119999982 ) ) ;
#1833=CARTESIAN_POINT ( 'NONE',  ( -2.637362731009999628, -63.41849336990000552, -25.81630194210000084 ) ) ;
#1835=CARTESIAN_POINT ( 'NONE',  ( 9.119206670260000536, -37.35114128690000257, -22.23223931510000284 ) ) ;
#1837=CARTESIAN_POINT ( 'NONE',  ( -20.05193632720000352, -56.21886023140000077, 14.45194103890000115 ) ) ;
#1838=CARTESIAN_POINT ( 'NONE',  ( -7.325370793560000315, -18.50000000000000000, -24.94672208400000102 ) ) ;
#1839=VECTOR ( 'NONE', #23657, 1000.000000000000000 ) ;
#1842=ORIENTED_EDGE ( 'NONE', *, *, #21864, .F. ) ;
#1847=CARTESIAN_POINT ( 'NONE',  ( -14.01337419900000114, -80.50000122480000186, 36.66316728649999845 ) ) ;
#1848=B_SPLINE_CURVE_WITH_KNOTS ( 'NONE', 3,
 ( #17090, #4113, #21330, #21747 ),
 .UNSPECIFIED., .F., .F.,
 ( 4, 4 ),
 ( 43.40831274110000493, 64.82354956899999365 ),
 .UNSPECIFIED. ) ;
#1849=CARTESIAN_POINT ( 'NONE',  ( 21.68822907590000071, -32.69575302460000188, 9.703736337280000512 ) ) ;
#1852=CARTESIAN_POINT ( 'NONE',  ( -22.17746619903529393, -74.18074980451231681, -32.62167336490611547 ) ) ;
#1853=CARTESIAN_POINT ( 'NONE',  ( 21.93023569320000021, -18.86697026210000061, 9.455903453530000391 ) ) ;
#1854=CARTESIAN_POINT ( 'NONE',  ( -32.27586754510721789, -74.04145547921538650, -22.09313380603792965 ) ) ;
#1855=FACE_OUTER_BOUND ( 'NONE', #11619, .T. ) ;
#1857=CARTESIAN_POINT ( 'NONE',  ( -11.35954001540000036, -77.00000000000000000, 47.25000000000000000 ) ) ;
#1864=CARTESIAN_POINT ( 'NONE',  ( -32.72159597179999935, -74.32000120609998817, -21.62349002899999917 ) ) ;
#1865=CARTESIAN_POINT ( 'NONE',  ( 36.82697887429999639, -80.34292022450000559, -13.57704389889999952 ) ) ;
#1866=ORIENTED_EDGE ( 'NONE', *, *, #9808, .T. ) ;
#1869=ORIENTED_EDGE ( 'NONE', *, *, #16399, .F. ) ;
#1872=CARTESIAN_POINT ( 'NONE',  ( 20.80630267519999776, -56.26441942339999969, 10.67761382389999980 ) ) ;
#1876=AXIS2_PLACEMENT_3D ( 'NONE', #18888, #21344, #19160 ) ;
#1878=DIRECTION ( 'NONE',  ( 0.000000000000000000, 1.000000000000000000, 0.000000000000000000 ) ) ;
#1879=VECTOR ( 'NONE', #28593, 1000.000000000000000 ) ;
#1880=EDGE_CURVE ( 'NONE', #10144, #21742, #24393, .T. ) ;
#1881=ORIENTED_EDGE ( 'NONE', *, *, #16956, .T. ) ;
#1883=CARTESIAN_POINT ( 'NONE',  ( 8.677144179139999025, -37.95796631150000167, -21.92880660169999985 ) ) ;
#1884=EDGE_CURVE ( 'NONE', #18491, #14378, #5952, .T. ) ;
#1890=CARTESIAN_POINT ( 'NONE',  ( 43.75000000000000000, -69.00000000000000000, 5.357814579270000097E-15 ) ) ;
#1891=CARTESIAN_POINT ( 'NONE',  ( -1.456904695340000000, -52.62618816519999854, -23.34673678599999747 ) ) ;
#1893=CARTESIAN_POINT ( 'NONE',  ( -19.28592236889999612, -18.62259217289999924, 14.63927399419999986 ) ) ;
#1894=ORIENTED_EDGE ( 'NONE', *, *, #28364, .T. ) ;
#1895=CARTESIAN_POINT ( 'NONE',  ( 21.87916729830000051, -37.95567969540000064, -8.611777603180000185 ) ) ;
#1903=CARTESIAN_POINT ( 'NONE',  ( 0.000000000000000000, -82.50000000000000000, 0.000000000000000000 ) ) ;
#1904=ORIENTED_EDGE ( 'NONE', *, *, #14580, .T. ) ;
#1906=ORIENTED_EDGE ( 'NONE', *, *, #23202, .T. ) ;
#1907=CARTESIAN_POINT ( 'NONE',  ( 21.49312271550000020, -37.09790470500000481, -7.530701653909999571 ) ) ;
#1908=CARTESIAN_POINT ( 'NONE',  ( -27.40038777100000189, -79.50000000000000000, -36.59277592640000165 ) ) ;
#1911=ADVANCED_FACE ( 'NONE', ( #6716 ), #17337, .T. ) ;
#1912=CARTESIAN_POINT ( 'NONE',  ( -3.380041727002253360, -68.16711249679821094, -27.59188392963350722 ) ) ;
#1916=DIRECTION ( 'NONE',  ( 1.000000000000000000, 0.000000000000000000, 0.000000000000000000 ) ) ;
#1917=CARTESIAN_POINT ( 'NONE',  ( 7.877988450750000204, -44.92713668140000038, -21.74683343669999758 ) ) ;
#1918=CARTESIAN_POINT ( 'NONE',  ( -10.30842662390000086, -18.85738404119999956, -19.98383211290000006 ) ) ;
#1919=AXIS2_PLACEMENT_3D ( 'NONE', #17218, #19402, #17074 ) ;
#1921=ORIENTED_EDGE ( 'NONE', *, *, #12161, .F. ) ;
#1922=VECTOR ( 'NONE', #14020, 1000.000000000000000 ) ;
#1923=EDGE_CURVE ( 'NONE', #25992, #4890, #20258, .T. ) ;
#1924=CARTESIAN_POINT ( 'NONE',  ( 38.08875739639999836, -80.50000000000000000, -9.476764215410000247 ) ) ;
#1925=CIRCLE ( 'NONE', #12587, 0.5000000000000027756 ) ;
#1926=CYLINDRICAL_SURFACE ( 'NONE', #6555, 2.999999999999996447 ) ;
#1927=CARTESIAN_POINT ( 'NONE',  ( 25.61816187999999883, -70.36214388610000015, 11.04518488439999935 ) ) ;
#1934=CARTESIAN_POINT ( 'NONE',  ( 28.11846399170000055, -70.41239039510000453, 2.285062484099999569 ) ) ;
#1936=CARTESIAN_POINT ( 'NONE',  ( 8.064915741549999240, -60.56337174330000295, -22.40630470649999850 ) ) ;
#1937=DIRECTION ( 'NONE',  ( 0.000000000000000000, -1.000000000000000000, 0.000000000000000000 ) ) ;
#1938=CARTESIAN_POINT ( 'NONE',  ( 7.100559683520000220, -35.25283571269999783, -21.44183144160000154 ) ) ;
#1939=CARTESIAN_POINT ( 'NONE',  ( 24.33707037739999990, -62.95235822580000473, -9.864745197619999573 ) ) ;
#1943=AXIS2_PLACEMENT_3D ( 'NONE', #22771, #11669, #20426 ) ;
#1946=CARTESIAN_POINT ( 'NONE',  ( 21.21808891099999883, -34.59820414320000026, -7.670974023059999425 ) ) ;
#1948=DIRECTION ( 'NONE',  ( 0.000000000000000000, 1.000000000000000000, 0.000000000000000000 ) ) ;
#1951=EDGE_CURVE ( 'NONE', #11794, #15559, #4788, .T. ) ;
#1952=CARTESIAN_POINT ( 'NONE',  ( 47.25000000000000000, -82.25000000000000000, -2.331807164890000089E-15 ) ) ;
#1954=VERTEX_POINT ( 'NONE', #25078 ) ;
#1955=LINE ( 'NONE', #3984, #21735 ) ;
#1958=DIRECTION ( 'NONE',  ( 0.000000000000000000, -1.000000000000000000, 0.000000000000000000 ) ) ;
#1962=CARTESIAN_POINT ( 'NONE',  ( 21.95427213460000004, -18.85488210659999808, 0.1375582407400000040 ) ) ;
#1963=CARTESIAN_POINT ( 'NONE',  ( -38.70686962976382972, -73.76099270142834996, -7.188502612221714827 ) ) ;
#1964=AXIS2_PLACEMENT_3D ( 'NONE', #16281, #18341, #9721 ) ;
#1966=B_SPLINE_CURVE_WITH_KNOTS ( 'NONE', 3,
 ( #12469, #3105, #929, #21380 ),
 .UNSPECIFIED., .F., .F.,
 ( 4, 4 ),
 ( 12.39809316140000028, 33.81329059560000161 ),
 .UNSPECIFIED. ) ;
#1967=ORIENTED_EDGE ( 'NONE', *, *, #10658, .F. ) ;
#1970=FACE_OUTER_BOUND ( 'NONE', #5837, .T. ) ;
#1973=CARTESIAN_POINT ( 'NONE',  ( -12.41808103320000001, -68.06111992670000177, -23.59934042399999754 ) ) ;
#1975=CARTESIAN_POINT ( 'NONE',  ( 19.08554773649999703, -23.77700550180000150, -9.011477467469999780 ) ) ;
#1977=CARTESIAN_POINT ( 'NONE',  ( 8.477761133450002262, -18.62065275650000018, -19.62439763160000084 ) ) ;
#1979=CARTESIAN_POINT ( 'NONE',  ( 22.43277176080000146, -36.00000000000000000, -11.31764183710000005 ) ) ;
#1980=TOROIDAL_SURFACE ( 'NONE', #18270, 3.500000000000000000, 0.5000000000000000000 ) ;
#1981=CARTESIAN_POINT ( 'NONE',  ( -0.5884599110899999541, -61.88564085890000399, -23.95484640009999922 ) ) ;
#1982=CARTESIAN_POINT ( 'NONE',  ( 9.276353521389999912, -36.53050716039999912, -21.68616227190000245 ) ) ;
#1984=AXIS2_PLACEMENT_3D ( 'NONE', #28253, #19510, #26226 ) ;
#1986=LINE ( 'NONE', #6486, #21980 ) ;
#1989=CARTESIAN_POINT ( 'NONE',  ( 21.18700933639999917, -34.99644735399999718, -7.990241917319999665 ) ) ;
#1990=CARTESIAN_POINT ( 'NONE',  ( 7.250122995579999952, -74.26794181930000605, -40.35968420239999688 ) ) ;
#1991=ORIENTED_EDGE ( 'NONE', *, *, #2998, .F. ) ;
#1993=EDGE_CURVE ( 'NONE', #12701, #3611, #23180, .T. ) ;
#1995=CARTESIAN_POINT ( 'NONE',  ( 22.75370980639999985, -39.29539198459999483, 10.16485029849999933 ) ) ;
#1997=CARTESIAN_POINT ( 'NONE',  ( 20.89748452499999942, -18.85965710059999978, 9.255084173580000240 ) ) ;
#1998=CARTESIAN_POINT ( 'NONE',  ( -31.64302845809999809, -80.00000000000000000, -31.64302845809999809 ) ) ;
#2000=EDGE_LOOP ( 'NONE', ( #9337, #20592, #14416, #15306 ) ) ;
#2003=DIRECTION ( 'NONE',  ( 0.000000000000000000, 1.000000000000000000, 0.000000000000000000 ) ) ;
#2007=CARTESIAN_POINT ( 'NONE',  ( 22.26662627820000040, -57.47855601759999900, -7.066909182079999852 ) ) ;
#2008=EDGE_LOOP ( 'NONE', ( #908, #8153, #15070, #18161 ) ) ;
#2009=EDGE_CURVE ( 'NONE', #27945, #3729, #16402, .T. ) ;
#2010=CARTESIAN_POINT ( 'NONE',  ( -32.65293188559999749, -74.37556698459998472, -21.99847587569999874 ) ) ;
#2011=CARTESIAN_POINT ( 'NONE',  ( 36.82697887990000396, -80.49999984420000487, -13.57704388640000026 ) ) ;
#2014=CARTESIAN_POINT ( 'NONE',  ( 28.69894351740000360, -74.00000000000000000, -10.33698117210000156 ) ) ;
#2015=CARTESIAN_POINT ( 'NONE',  ( -11.91266501540000000, -74.00000000000000000, 46.64429291560000479 ) ) ;
#2016=CARTESIAN_POINT ( 'NONE',  ( -0.6273717453279999967, -62.97603269449999885, -24.27362655359999977 ) ) ;
#2022=VERTEX_POINT ( 'NONE', #18224 ) ;
#2029=CARTESIAN_POINT ( 'NONE',  ( -3.501402190497391764, -79.99970154920160326, 46.83644880644524022 ) ) ;
#2030=VERTEX_POINT ( 'NONE', #22749 ) ;
#2031=DIRECTION ( 'NONE',  ( 0.000000000000000000, -1.000000000000000000, 0.000000000000000000 ) ) ;
#2034=CARTESIAN_POINT ( 'NONE',  ( -2.565581297390000071, -56.20810645120000260, -24.89562038480000083 ) ) ;
#2035=CIRCLE ( 'NONE', #21558, 3.750000000000000000 ) ;
#2036=CARTESIAN_POINT ( 'NONE',  ( 21.91842626080000045, -37.33819205729999879, -8.685017708060000174 ) ) ;
#2037=CARTESIAN_POINT ( 'NONE',  ( 11.35129741066615772, -72.28566294331933761, -26.99897349783034173 ) ) ;
#2038=DIRECTION ( 'NONE',  ( 1.000000000000000000, 0.000000000000000000, 0.000000000000000000 ) ) ;
#2045=EDGE_CURVE ( 'NONE', #2214, #18911, #16432, .T. ) ;
#2047=CARTESIAN_POINT ( 'NONE',  ( 23.35417726369999869, -57.47855601759999900, -0.5711878298099999363 ) ) ;
#2049=CYLINDRICAL_SURFACE ( 'NONE', #16359, 7.249999999999999112 ) ;
#2051=ORIENTED_EDGE ( 'NONE', *, *, #10364, .F. ) ;
#2054=EDGE_LOOP ( 'NONE', ( #13030, #5016, #1072, #11165 ) ) ;
#2055=AXIS2_PLACEMENT_3D ( 'NONE', #20796, #27499, #3031 ) ;
#2056=CARTESIAN_POINT ( 'NONE',  ( -13.24460949610000071, -57.44036993110000111, 20.55651328140000089 ) ) ;
#2057=CARTESIAN_POINT ( 'NONE',  ( 7.734359568749999525, -19.46510050329999686, -20.63161913629999944 ) ) ;
#2060=CARTESIAN_POINT ( 'NONE',  ( -3.158285342964013864, -66.99924750834972542, -27.22922173955624103 ) ) ;
#2065=CARTESIAN_POINT ( 'NONE',  ( 7.554088719370000149, -44.93138465010000004, -21.71814693689999842 ) ) ;
#2071=CARTESIAN_POINT ( 'NONE',  ( 23.77822920909999738, -34.63364287800000341, 1.297513282619999986 ) ) ;
#2072=DIRECTION ( 'NONE',  ( 0.000000000000000000, -1.000000000000000000, 0.000000000000000000 ) ) ;
#2073=CARTESIAN_POINT ( 'NONE',  ( 39.68146194264046045, -73.78481856921511906, 7.243236069894346763 ) ) ;
#2075=CIRCLE ( 'NONE', #15073, 1.000000000000000888 ) ;
#2076=CARTESIAN_POINT ( 'NONE',  ( -38.62788659690000515, -74.00000000000000000, 7.627568735119999666 ) ) ;
#2079=ORIENTED_EDGE ( 'NONE', *, *, #21648, .T. ) ;
#2080=CARTESIAN_POINT ( 'NONE',  ( 28.64987595179999857, -71.11747349450000399, 2.769230177229999867 ) ) ;
#2083=CARTESIAN_POINT ( 'NONE',  ( 7.066909115259999652, -57.47855582819999398, -22.26662700550000196 ) ) ;
#2084=CARTESIAN_POINT ( 'NONE',  ( -12.80265261289999934, -69.66305826589999128, -24.04850811530000243 ) ) ;
#2086=CARTESIAN_POINT ( 'NONE',  ( -11.38378090099999973, -42.27112620159999778, -19.87481931789999834 ) ) ;
#2088=ADVANCED_FACE ( 'NONE', ( #9471 ), #18377, .F. ) ;
#2089=CARTESIAN_POINT ( 'NONE',  ( 26.96515717169932458, -69.06126107724072938, 0.3323215380678566366 ) ) ;
#2090=DIRECTION ( 'NONE',  ( 0.000000000000000000, -1.000000000000000000, 0.000000000000000000 ) ) ;
#2096=AXIS2_PLACEMENT_3D ( 'NONE', #17159, #12767, #26049 ) ;
#2098=LINE ( 'NONE', #24516, #20244 ) ;
#2102=CIRCLE ( 'NONE', #21640, 34.89999999999999858 ) ;
#2103=CARTESIAN_POINT ( 'NONE',  ( 47.25000000000000000, -80.00000000000000000, 8.881784196999999612E-15 ) ) ;
#2106=CARTESIAN_POINT ( 'NONE',  ( 8.882291244119999263, -35.85669613890000562, -20.42811047029999827 ) ) ;
#2107=CARTESIAN_POINT ( 'NONE',  ( 9.356041104380000917, -74.00000000000000000, 37.60355029590000697 ) ) ;
#2110=CARTESIAN_POINT ( 'NONE',  ( 21.84042253680000201, -18.61797548019999837, 0.5293533609709999421 ) ) ;
#2111=CARTESIAN_POINT ( 'NONE',  ( -12.11328434900106288, -19.47102482557679437, 19.13567261410544162 ) ) ;
#2116=CARTESIAN_POINT ( 'NONE',  ( 6.974892859179999682, -49.11505549650000546, -21.98941332900000134 ) ) ;
#2119=DIRECTION ( 'NONE',  ( 0.000000000000000000, 1.000000000000000000, 0.000000000000000000 ) ) ;
#2124=CARTESIAN_POINT ( 'NONE',  ( 8.426926234210000644, -18.85979317139999978, -20.10370215430000229 ) ) ;
#2125=EDGE_CURVE ( 'NONE', #5033, #6426, #24805, .T. ) ;
#2126=ORIENTED_EDGE ( 'NONE', *, *, #907, .F. ) ;
#2127=CARTESIAN_POINT ( 'NONE',  ( -13.64611331559999918, -63.24140639400000197, 21.34096686680000232 ) ) ;
#2129=DIRECTION ( 'NONE',  ( 0.9993816408608722224, 0.000000000000000000, -0.03516156865429610756 ) ) ;
#2130=VERTEX_POINT ( 'NONE', #7867 ) ;
#2133=ORIENTED_EDGE ( 'NONE', *, *, #9374, .F. ) ;
#2135=FACE_OUTER_BOUND ( 'NONE', #19826, .T. ) ;
#2136=CARTESIAN_POINT ( 'NONE',  ( 21.33821989950000031, -45.98073373389999574, 9.994986904390001925 ) ) ;
#2140=CARTESIAN_POINT ( 'NONE',  ( 19.85636362560000023, -19.46458168450000059, 9.829421693009999572 ) ) ;
#2141=CARTESIAN_POINT ( 'NONE',  ( 9.797124920099999912, -69.55058719230000008, -25.58514975119999946 ) ) ;
#2143=EDGE_LOOP ( 'NONE', ( #25750, #28206, #7134, #28651 ) ) ;
#2144=CARTESIAN_POINT ( 'NONE',  ( -11.78425688200000110, -72.00000000000000000, -26.58404760160000180 ) ) ;
#2146=CARTESIAN_POINT ( 'NONE',  ( -23.16986609970000188, -72.82938648530000592, 16.90925194980000157 ) ) ;
#2147=CARTESIAN_POINT ( 'NONE',  ( 23.17288685498201417, -62.96215878643922537, -7.400562784300776187 ) ) ;
#2148=VERTEX_POINT ( 'NONE', #14824 ) ;
#2151=CARTESIAN_POINT ( 'NONE',  ( -32.57680276909999151, -74.14930846740000447, -22.16666910030000182 ) ) ;
#2156=DIRECTION ( 'NONE',  ( 0.000000000000000000, 1.000000000000000000, 0.000000000000000000 ) ) ;
#2157=B_SPLINE_CURVE_WITH_KNOTS ( 'NONE', 3,
 ( #26786, #13497, #22405, #6667, #4181, #13052, #21965, #15532, #15680, #2158, #20211 ),
 .UNSPECIFIED., .F., .F.,
 ( 4, 1, 1, 1, 2, 2, 4 ),
 ( 0.000000000000000000, 0.2500000000000006661, 0.3750000000000009992, 0.4375000000000008882, 0.4687500000000011102, 0.5000000000000013323, 1.000000000000000000 ),
 .UNSPECIFIED. ) ;
#2158=CARTESIAN_POINT ( 'NONE',  ( 24.55110012684054865, -25.78856419227151164, 1.431078990032156772 ) ) ;
#2159=CARTESIAN_POINT ( 'NONE',  ( -22.46797588158592163, -80.18584073532525736, -32.25831116885107264 ) ) ;
#2162=VERTEX_POINT ( 'NONE', #14555 ) ;
#2164=CARTESIAN_POINT ( 'NONE',  ( 46.12332287689999788, -74.00000000000000000, -4.489694494070000097 ) ) ;
#2166=CARTESIAN_POINT ( 'NONE',  ( 22.02882315030000271, -19.46510050329999686, -0.4636558402470000173 ) ) ;
#2171=LINE ( 'NONE', #24755, #20845 ) ;
#2172=ORIENTED_EDGE ( 'NONE', *, *, #2522, .T. ) ;
#2173=CARTESIAN_POINT ( 'NONE',  ( 36.22844186549999534, -74.00000000000000000, -13.75000000000000000 ) ) ;
#2177=CARTESIAN_POINT ( 'NONE',  ( 19.97576656849999921, -38.00000000000000000, -19.97576656849999921 ) ) ;
#2178=CARTESIAN_POINT ( 'NONE',  ( 11.27834831967279250, -72.32257210994342245, -26.96386658466257913 ) ) ;
#2179=CARTESIAN_POINT ( 'NONE',  ( 21.46816240343896354, -36.17003871385012559, -7.279245513745156160 ) ) ;
#2182=CARTESIAN_POINT ( 'NONE',  ( 20.34468230811009803, -73.94794535334492025, -32.44681540213797888 ) ) ;
#2184=CARTESIAN_POINT ( 'NONE',  ( 7.105427357599999217E-15, -74.50000000000000000, 3.552713678799999608E-15 ) ) ;
#2186=DIRECTION ( 'NONE',  ( 0.1988145312159089739, -0.9099612708765829616, 0.3639275582888334415 ) ) ;
#2187=B_SPLINE_SURFACE_WITH_KNOTS ( 'NONE', 5, 5, ( 
 ( #13574, #501, #20282, #2968, #3113, #12250 ),
 ( #9497, #20880, #7328, #21024, #27590, #16631 ),
 ( #5563, #20841, #13834, #903, #759, #11633 ),
 ( #9745, #25066, #27251, #27553, #5098, #7447 ),
 ( #7732, #23169, #7290, #16599, #16305, #16158 ),
 ( #9605, #20392, #28608, #8639, #26577, #2249 ),
 ( #10812, #15329, #4719, #20160, #4870, #13300 ),
 ( #13448, #8776, #24246, #26733, #9218, #4284 ),
 ( #11092, #11255, #22508, #2552, #17689, #7064 ) ),
 .UNSPECIFIED., .F., .F., .F.,
 ( 6, 3, 6 ),
 ( 6, 6 ),
 ( 4.255758722390000039E-16, 2.251105601749999963, 5.576980223840000583 ),
 ( 0.000000000000000000, 1.000000000000000000 ),
 .UNSPECIFIED. ) ;
#2189=DIRECTION ( 'NONE',  ( 0.000000000000000000, -1.000000000000000000, 0.000000000000000000 ) ) ;
#2193=CARTESIAN_POINT ( 'NONE',  ( 19.97576656849999921, -72.00000000000000000, -19.97576656849999921 ) ) ;
#2201=CARTESIAN_POINT ( 'NONE',  ( 26.98670340789999855, -72.82938977469999031, -9.720255250690000182 ) ) ;
#2204=VERTEX_POINT ( 'NONE', #8142 ) ;
#2206=CARTESIAN_POINT ( 'NONE',  ( 24.43813899739999940, -34.61119146829999238, 1.434554263020000109 ) ) ;
#2207=CARTESIAN_POINT ( 'NONE',  ( -14.57962358425329441, -80.29877500280160518, 36.44181020648760949 ) ) ;
#2209=ORIENTED_EDGE ( 'NONE', *, *, #11403, .F. ) ;
#2210=EDGE_CURVE ( 'NONE', #14378, #14143, #26484, .T. ) ;
#2211=CARTESIAN_POINT ( 'NONE',  ( -40.70731707320000226, -82.25000000000000000, 7.215414233289999757 ) ) ;
#2214=VERTEX_POINT ( 'NONE', #13064 ) ;
#2215=TOROIDAL_SURFACE ( 'NONE', #6375, 10.50000000000000000, 0.5000000000000000000 ) ;
#2218=CARTESIAN_POINT ( 'NONE',  ( 11.81986579350000000, -72.00000321289999761, -27.35691362350000233 ) ) ;
#2219=CARTESIAN_POINT ( 'NONE',  ( -12.21349012499999986, -68.60731645090001507, -24.28095208079999878 ) ) ;
#2220=CARTESIAN_POINT ( 'NONE',  ( 23.83794015770000030, -65.05904285249999930, -7.999567420579999144 ) ) ;
#2221=FACE_OUTER_BOUND ( 'NONE', #24886, .T. ) ;
#2222=CARTESIAN_POINT ( 'NONE',  ( 0.000000000000000000, -19.46510050329999686, 0.000000000000000000 ) ) ;
#2224=ORIENTED_EDGE ( 'NONE', *, *, #23202, .F. ) ;
#2227=CARTESIAN_POINT ( 'NONE',  ( 7.561758309989084381, -74.02518802157058531, 38.96765197712635143 ) ) ;
#2228=ORIENTED_EDGE ( 'NONE', *, *, #26230, .F. ) ;
#2229=CARTESIAN_POINT ( 'NONE',  ( 36.24656994149999889, -79.00000000000000000, -15.05817610060000078 ) ) ;
#2231=AXIS2_PLACEMENT_3D ( 'NONE', #13767, #5179, #7226 ) ;
#2234=CARTESIAN_POINT ( 'NONE',  ( 26.85898284228529675, -72.46277288053744314, -10.97019792874640842 ) ) ;
#2236=CARTESIAN_POINT ( 'NONE',  ( 9.259752875310001130, -35.97005431750000071, -20.12202164109999813 ) ) ;
#2237=EDGE_CURVE ( 'NONE', #7849, #25813, #19774, .T. ) ;
#2238=CARTESIAN_POINT ( 'NONE',  ( 21.49223700067187082, -35.65578321604039758, -6.986316714794048366 ) ) ;
#2242=B_SPLINE_CURVE_WITH_KNOTS ( 'NONE', 3,
 ( #21844, #19936, #8856, #6845, #24321, #17919, #22143, #2182, #22283, #15709 ),
 .UNSPECIFIED., .F., .F.,
 ( 4, 2, 2, 2, 4 ),
 ( 0.000000000000000000, 0.2500000000000000000, 0.5000000000000000000, 0.7500000000000000000, 1.000000000000000000 ),
 .UNSPECIFIED. ) ;
#2243=CARTESIAN_POINT ( 'NONE',  ( 21.12093416029999915, -18.50000000000000000, 0.3961283385739999829 ) ) ;
#2249=CARTESIAN_POINT ( 'NONE',  ( -12.75967654059999923, -19.47871525829999939, 19.36958737249999984 ) ) ;
#2253=DIRECTION ( 'NONE',  ( 0.4794255386042036160, 0.000000000000000000, 0.8775825618903723147 ) ) ;
#2259=CARTESIAN_POINT ( 'NONE',  ( 7.938154596009999509, -18.61853073680000037, -20.14564044980000190 ) ) ;
#2261=AXIS2_PLACEMENT_3D ( 'NONE', #18980, #20753, #19117 ) ;
#2264=CARTESIAN_POINT ( 'NONE',  ( -13.24460878530000052, -57.44036942000000323, 20.55651963289999884 ) ) ;
#2265=DIRECTION ( 'NONE',  ( 1.000000000000000000, 0.000000000000000000, 0.000000000000000000 ) ) ;
#2266=PRODUCT_DEFINITION_FORMATION_WITH_SPECIFIED_SOURCE ( 'ANY', '', #26438, .NOT_KNOWN. ) ;
#2268=CARTESIAN_POINT ( 'NONE',  ( -20.56017862280000230, -57.40875702389999446, 14.85415739589999973 ) ) ;
#2269=CARTESIAN_POINT ( 'NONE',  ( -12.17175180279999935, -57.47855601759999900, -19.93971687999999887 ) ) ;
#2270=ORIENTED_EDGE ( 'NONE', *, *, #11763, .T. ) ;
#2271=CARTESIAN_POINT ( 'NONE',  ( -7.229383731089999543, -73.50070240710000746, -39.23650411529999360 ) ) ;
#2272=CARTESIAN_POINT ( 'NONE',  ( 29.82081051618066780, -74.26904473745747737, -25.43758724625505252 ) ) ;
#2274=ORIENTED_EDGE ( 'NONE', *, *, #28406, .F. ) ;
#2276=ORIENTED_EDGE ( 'NONE', *, *, #15508, .F. ) ;
#2278=AXIS2_PLACEMENT_3D ( 'NONE', #10141, #21663, #14531 ) ;
#2279=CARTESIAN_POINT ( 'NONE',  ( 22.76317971519999972, -52.57401960329947599, 10.17780311019999040 ) ) ;
#2281=CARTESIAN_POINT ( 'NONE',  ( 22.02546240290000057, -32.68478243020000207, 9.763264387630000485 ) ) ;
#2284=EDGE_CURVE ( 'NONE', #11938, #13357, #2873, .T. ) ;
#2285=CARTESIAN_POINT ( 'NONE',  ( -13.92979211509999971, -74.00000000010000178, 36.25622248599999864 ) ) ;
#2289=DIRECTION ( 'NONE',  ( 0.09756097560976655092, 0.000000000000000000, 0.9952295494196655712 ) ) ;
#2291=CARTESIAN_POINT ( 'NONE',  ( -11.35954001540000036, -74.50000000000000000, 45.25000000000000000 ) ) ;
#2292=FACE_OUTER_BOUND ( 'NONE', #7261, .T. ) ;
#2293=CARTESIAN_POINT ( 'NONE',  ( -40.32207487330000362, -74.31847293650000097, -7.253641904939999385 ) ) ;
#2294=ORIENTED_EDGE ( 'NONE', *, *, #16116, .F. ) ;
#2297=ORIENTED_EDGE ( 'NONE', *, *, #25993, .T. ) ;
#2298=AXIS2_PLACEMENT_3D ( 'NONE', #13070, #4488, #6535 ) ;
#2302=DIRECTION ( 'NONE',  ( 0.000000000000000000, 1.000000000000000000, 0.000000000000000000 ) ) ;
#2304=ORIENTED_EDGE ( 'NONE', *, *, #4696, .T. ) ;
#2307=CARTESIAN_POINT ( 'NONE',  ( 46.58837163849999996, -73.69423725189999175, -3.076420046560000010 ) ) ;
#2309=DIRECTION ( 'NONE',  ( 0.7071067811865474617, 0.000000000000000000, 0.7071067811865474617 ) ) ;
#2311=ADVANCED_FACE ( 'NONE', ( #26636 ), #23665, .T. ) ;
#2313=CARTESIAN_POINT ( 'NONE',  ( 8.564557077759998194, -37.33500411810000230, -21.83114817979999955 ) ) ;
#2320=CARTESIAN_POINT ( 'NONE',  ( -39.92836808239999868, -74.14144860030000928, 7.283536107469999799 ) ) ;
#2321=CARTESIAN_POINT ( 'NONE',  ( -13.16183723299999997, -70.12921532840000793, -24.09258145020000086 ) ) ;
#2325=CARTESIAN_POINT ( 'NONE',  ( 7.435977656837697403, -74.13942000216081851, -39.48500436385279500 ) ) ;
#2326=EDGE_LOOP ( 'NONE', ( #7698, #1566, #991, #23620, #5841, #13146 ) ) ;
#2327=DIRECTION ( 'NONE',  ( 1.000000000000000000, 0.000000000000000000, 0.000000000000000000 ) ) ;
#2331=DIRECTION ( 'NONE',  ( 0.9704142011833033488, 0.000000000000000000, -0.2414462220490755373 ) ) ;
#2333=EDGE_CURVE ( 'NONE', #15756, #5488, #26795, .T. ) ;
#2335=CARTESIAN_POINT ( 'NONE',  ( 23.90606521969999676, -57.45864773929999814, 0.8443132633689999222 ) ) ;
#2337=CARTESIAN_POINT ( 'NONE',  ( -11.35954001540000036, -80.00000000000000000, 46.75000000000000000 ) ) ;
#2338=TOROIDAL_SURFACE ( 'NONE', #13961, 3.750000000000000000, 1.000000000000000000 ) ;
#2340=DIRECTION ( 'NONE',  ( 0.000000000000000000, 1.000000000000000000, 0.000000000000000000 ) ) ;
#2343=CARTESIAN_POINT ( 'NONE',  ( -13.15709823100000087, -49.83805748250000534, 20.35711383789999829 ) ) ;
#2344=ORIENTED_EDGE ( 'NONE', *, *, #10399, .F. ) ;
#2353=CARTESIAN_POINT ( 'NONE',  ( 47.19173749819621122, -79.33634930001392149, -1.160608118433608560 ) ) ;
#2356=CARTESIAN_POINT ( 'NONE',  ( -20.29409717112922706, -60.89354426525722630, 12.37746592674120905 ) ) ;
#2358=ORIENTED_EDGE ( 'NONE', *, *, #19305, .T. ) ;
#2360=CARTESIAN_POINT ( 'NONE',  ( -11.46863496920000003, -57.40875702469999453, -22.62382260909999943 ) ) ;
#2365=CARTESIAN_POINT ( 'NONE',  ( 27.04142406090000250, -68.97505732880000551, 1.205035742480000005 ) ) ;
#2366=AXIS2_PLACEMENT_3D ( 'NONE', #17586, #15526, #8822 ) ;
#2369=CARTESIAN_POINT ( 'NONE',  ( -46.75000000000000000, -69.50000000000000000, -1.262878690509999918E-15 ) ) ;
#2370=CARTESIAN_POINT ( 'NONE',  ( 23.84797911320000097, -63.15653191699999525, -9.592766500679999808 ) ) ;
#2372=DIRECTION ( 'NONE',  ( 0.000000000000000000, 1.000000000000000000, 0.000000000000000000 ) ) ;
#2379=ORIENTED_EDGE ( 'NONE', *, *, #8825, .F. ) ;
#2380=CIRCLE ( 'NONE', #3760, 38.75000000000000000 ) ;
#2385=CARTESIAN_POINT ( 'NONE',  ( 23.50367701526724673, -19.48459430185724273, 1.423420176684405902 ) ) ;
#2388=DIRECTION ( 'NONE',  ( 0.2414462220490755373, 0.000000000000000000, -0.9704142011833033488 ) ) ;
#2391=CARTESIAN_POINT ( 'NONE',  ( 8.690400270730000543, -36.30003840290000028, -21.06640817119999554 ) ) ;
#2392=CARTESIAN_POINT ( 'NONE',  ( 21.55117138126461995, -36.19847887270072562, -6.864724801166914858 ) ) ;
#2400=CARTESIAN_POINT ( 'NONE',  ( 6.850353625200000351, -36.56979901409999911, -21.56931447779999900 ) ) ;
#2401=CARTESIAN_POINT ( 'NONE',  ( 36.34915583725175026, -75.00000019643333360, -14.88857262638677703 ) ) ;
#2402=CARTESIAN_POINT ( 'NONE',  ( 25.87390537659780776, -62.05304730950737024, 1.417947247737919358 ) ) ;
#2404=DIRECTION ( 'NONE',  ( 0.4794255386042040601, 0.000000000000000000, 0.8775825618903720926 ) ) ;
#2405=CIRCLE ( 'NONE', #6097, 3.000000000000000888 ) ;
#2406=ORIENTED_EDGE ( 'NONE', *, *, #16021, .T. ) ;
#2407=CIRCLE ( 'NONE', #24256, 30.50381168839999901 ) ;
#2408=CARTESIAN_POINT ( 'NONE',  ( -32.20769385759999892, -80.50000045429999318, -22.43272066369999962 ) ) ;
#2410=EDGE_CURVE ( 'NONE', #5413, #723, #6976, .T. ) ;
#2414=CARTESIAN_POINT ( 'NONE',  ( -13.55408830789999897, -67.56935268729999677, 22.52790492979999826 ) ) ;
#2421=CIRCLE ( 'NONE', #22430, 32.39999999999999858 ) ;
#2422=CARTESIAN_POINT ( 'NONE',  ( -11.31871641743052415, -57.41946977428668930, -22.35641880394745939 ) ) ;
#2423=ORIENTED_EDGE ( 'NONE', *, *, #27873, .F. ) ;
#2424=CARTESIAN_POINT ( 'NONE',  ( -7.196178079599999222, -73.81415926540000783, -38.70548889989999708 ) ) ;
#2425=CARTESIAN_POINT ( 'NONE',  ( 30.59674585478018116, -74.18273825083886663, -24.40299353443661445 ) ) ;
#2428=VECTOR ( 'NONE', #3553, 1000.000000000000000 ) ;
#2429=CARTESIAN_POINT ( 'NONE',  ( -15.42363691649999957, -19.50000000000000000, 22.84488648889999851 ) ) ;
#2430=ORIENTED_EDGE ( 'NONE', *, *, #15609, .T. ) ;
#2433=CARTESIAN_POINT ( 'NONE',  ( 22.34015708469999950, -32.67314204010000367, 9.890958026079999854 ) ) ;
#2435=CARTESIAN_POINT ( 'NONE',  ( -7.248366623730185587, -73.88016183361062872, -39.84605369631500338 ) ) ;
#2436=CARTESIAN_POINT ( 'NONE',  ( 22.14322190709999916, -64.99357404969998697, 11.84671812930000101 ) ) ;
#2437=CARTESIAN_POINT ( 'NONE',  ( 9.855634484279999441, -64.48636388919999263, -24.31831199750000039 ) ) ;
#2439=B_SPLINE_SURFACE_WITH_KNOTS ( 'NONE', 5, 5, ( 
 ( #4421, #4123, #23560, #24238, #8627, #22058, #7835, #3594, #7972 ),
 ( #21908, #16716, #6310, #2106, #10653, #17681, #16862, #26569, #24086 ),
 ( #10129, #15469, #1162, #18914, #25752, #21106, #9999, #27794, #5642 ),
 ( #14521, #23424, #3463, #19712, #12329, #28599, #21237, #19050, #5777 ),
 ( #14665, #21370, #1426, #19570, #28457, #8493, #17393, #20295, #22196 ),
 ( #18414, #24823, #2541, #4861, #2391, #22498, #363, #13742, #15917 ),
 ( #27011, #24522, #19998, #9069, #24966, #20151, #22788, #27303, #22343 ),
 ( #13292, #11082, #11689, #11394, #71, #4558, #24674, #20447, #25119 ),
 ( #13886, #7341, #15622, #17826, #20600, #11246, #7054, #7198, #6904 ),
 ( #8917, #2236, #26721, #16207, #4710, #15768, #6760, #13437, #26865 ),
 ( #222, #17971, #9208, #517, #16064, #13590, #4996, #18118, #22642 ),
 ( #9512, #2681, #2827, #659, #11538, #9364, #18265, #27158, #21303 ) ),
 .UNSPECIFIED., .F., .F., .F.,
 ( 6, 3, 3, 6 ),
 ( 6, 3, 6 ),
 ( 8.754352264609998713, 10.05054279850000043, 10.42202991689999969, 11.17956741670000120 ),
 ( 0.000000000000000000, 1.000000000000000000, 2.000000000000000000 ),
 .UNSPECIFIED. ) ;
#2441=DIRECTION ( 'NONE',  ( 1.000000000000000000, 0.000000000000000000, 1.224606353820001308E-16 ) ) ;
#2442=CARTESIAN_POINT ( 'NONE',  ( 27.35691632010000163, -72.00000328939999861, -11.81987169600000165 ) ) ;
#2444=CARTESIAN_POINT ( 'NONE',  ( 40.00000000000000000, -82.25000000000000000, 0.000000000000000000 ) ) ;
#2445=CARTESIAN_POINT ( 'NONE',  ( 22.76364019028259023, -61.39309059898780419, -7.242868441357485310 ) ) ;
#2446=ORIENTED_EDGE ( 'NONE', *, *, #3753, .F. ) ;
#2447=B_SPLINE_CURVE_WITH_KNOTS ( 'NONE', 3,
 ( #11671, #20582, #16192, #7483, #16345, #25253, #15902, #24809, #4846, #13725, #20427, #18247, #7183, #16050, #24952, #5963, #9920, #12248, #27990, #7764, #10459, #14445, #21285, #16914, #14578, #5836, #3797, #25667, #25810, #19377, #19102, #21160 ),
 .UNSPECIFIED., .F., .F.,
 ( 4, 2, 2, 1, 1, 2, 2, 2, 1, 1, 1, 2, 2, 2, 1, 1, 1, 2, 2, 4 ),
 ( 0.000000000000000000, 0.1250000000000721367, 0.1875000000001230960, 0.2187500000001387501, 0.2343750000001453282, 0.2421875000001490752, 0.2500000000001527667, 0.3750000000000960343, 0.4375000000000670575, 0.4687500000000578981, 0.4843750000000533462, 0.4921875000000504596, 0.5000000000000475175, 0.6250000000000074385, 0.6874999999999900080, 0.7187499999999837907, 0.7343749999999824585, 0.7421874999999835687, 0.7499999999999845679, 1.000000000000000000 ),
 .UNSPECIFIED. ) ;
#2449=ORIENTED_EDGE ( 'NONE', *, *, #24039, .F. ) ;
#2450=AXIS2_PLACEMENT_3D ( 'NONE', #8942, #11416, #6635 ) ;
#2454=CARTESIAN_POINT ( 'NONE',  ( -7.325370793560000315, -19.50000000000000000, -24.94672208400000102 ) ) ;
#2455=CARTESIAN_POINT ( 'NONE',  ( 20.06309763089999620, -36.00000000000000000, -9.476129751679998492 ) ) ;
#2459=ORIENTED_EDGE ( 'NONE', *, *, #8543, .T. ) ;
#2460=CARTESIAN_POINT ( 'NONE',  ( -21.35786096709999882, -65.07443093669999712, 13.27975207949999970 ) ) ;
#2463=ORIENTED_EDGE ( 'NONE', *, *, #9703, .F. ) ;
#2465=CARTESIAN_POINT ( 'NONE',  ( -22.00249006139999963, -79.69117347819999964, -32.67527200749999849 ) ) ;
#2469=TOROIDAL_SURFACE ( 'NONE', #20611, 2.500000000000000000, 0.5000000000000000000 ) ;
#2471=ORIENTED_EDGE ( 'NONE', *, *, #13476, .F. ) ;
#2474=CARTESIAN_POINT ( 'NONE',  ( -39.04179453189999549, -73.95640471630001400, 7.432602092579998931 ) ) ;
#2475=CARTESIAN_POINT ( 'NONE',  ( -22.22906645670000003, -74.50000000000000000, -32.83566817450000030 ) ) ;
#2477=FACE_OUTER_BOUND ( 'NONE', #6147, .T. ) ;
#2478=CARTESIAN_POINT ( 'NONE',  ( -7.557074492643517161, -73.99988188839131453, 38.78621575433889035 ) ) ;
#2481=FACE_OUTER_BOUND ( 'NONE', #14830, .T. ) ;
#2482=CARTESIAN_POINT ( 'NONE',  ( 8.508194257199999555, -34.61672919229999934, -20.76917589150000154 ) ) ;
#2484=EDGE_CURVE ( 'NONE', #19473, #26756, #19205, .T. ) ;
#2486=CARTESIAN_POINT ( 'NONE',  ( 20.34628061889999984, -52.63293862049999916, 11.13082833170000008 ) ) ;
#2492=CARTESIAN_POINT ( 'NONE',  ( 3.551183598479999925E-15, -73.00000000000000000, -32.75000000000000000 ) ) ;
#2493=EDGE_CURVE ( 'NONE', #14660, #16936, #15966, .T. ) ;
#2496=EDGE_LOOP ( 'NONE', ( #17005, #22893, #7729, #27076 ) ) ;
#2497=CARTESIAN_POINT ( 'NONE',  ( -11.20604483669999851, -42.27289973529999401, 19.89334194550000134 ) ) ;
#2499=CARTESIAN_POINT ( 'NONE',  ( 8.607507029887250027, -36.72040101226378539, -21.55953479827181951 ) ) ;
#2500=AXIS2_PLACEMENT_3D ( 'NONE', #304, #150, #9143 ) ;
#2502=CARTESIAN_POINT ( 'NONE',  ( 9.698193454340000130, -36.00000000010000178, -20.58262106160000116 ) ) ;
#2503=CARTESIAN_POINT ( 'NONE',  ( 26.13446004556505287, -70.56829302196123876, -9.039107915225594425 ) ) ;
#2504=CARTESIAN_POINT ( 'NONE',  ( -10.43683906909999948, -19.16174980609999778, -20.01792584879999737 ) ) ;
#2505=CARTESIAN_POINT ( 'NONE',  ( 21.59423340250210543, -37.77125957295557868, -8.020740188427190276 ) ) ;
#2507=DIRECTION ( 'NONE',  ( 0.000000000000000000, -1.000000000000000000, 0.000000000000000000 ) ) ;
#2509=CARTESIAN_POINT ( 'NONE',  ( -31.89935321680000158, -74.00000000000000000, -21.99985828019999801 ) ) ;
#2511=CIRCLE ( 'NONE', #27652, 4.750000000000000888 ) ;
#2512=DIRECTION ( 'NONE',  ( -5.788992577199999305E-17, 0.000000000000000000, 1.000000000000000000 ) ) ;
#2519=CARTESIAN_POINT ( 'NONE',  ( 22.79517987939305002, -74.07354942525847719, -31.66438262344599508 ) ) ;
#2521=CARTESIAN_POINT ( 'NONE',  ( -11.18016183240000139, -57.44036992910000095, -21.74842400150000188 ) ) ;
#2522=EDGE_CURVE ( 'NONE', #1018, #22701, #8968, .T. ) ;
#2523=CIRCLE ( 'NONE', #19242, 0.5000000000000004441 ) ;
#2525=AXIS2_PLACEMENT_3D ( 'NONE', #24621, #4504, #24469 ) ;
#2526=B_SPLINE_CURVE_WITH_KNOTS ( 'NONE', 2,
 ( #25786, #8006, #12910 ),
 .UNSPECIFIED., .F., .F.,
 ( 3, 3 ),
 ( 0.000000000000000000, 1.000000000000000000 ),
 .UNSPECIFIED. ) ;
#2529=ORIENTED_EDGE ( 'NONE', *, *, #27466, .F. ) ;
#2531=CARTESIAN_POINT ( 'NONE',  ( 23.17395180239999775, -18.50000000000000000, 2.380615958829999990 ) ) ;
#2532=DIRECTION ( 'NONE',  ( 0.000000000000000000, 1.000000000000000000, 0.000000000000000000 ) ) ;
#2533=DIRECTION ( 'NONE',  ( 0.7071067811865474617, 0.000000000000000000, 0.7071067811865474617 ) ) ;
#2535=CARTESIAN_POINT ( 'NONE',  ( 22.10171175959985845, -19.46474104946126005, 0.03556608548572790657 ) ) ;
#2537=ORIENTED_EDGE ( 'NONE', *, *, #16918, .T. ) ;
#2538=FACE_OUTER_BOUND ( 'NONE', #3298, .T. ) ;
#2541=CARTESIAN_POINT ( 'NONE',  ( 9.085163553980001083, -35.93116987310000354, -20.23957076829999835 ) ) ;
#2542=CARTESIAN_POINT ( 'NONE',  ( 8.280691199402831160, -19.47200836853050632, -20.32438904306839333 ) ) ;
#2543=ORIENTED_EDGE ( 'NONE', *, *, #21487, .F. ) ;
#2546=DIRECTION ( 'NONE',  ( 0.000000000000000000, -1.000000000000000000, 0.000000000000000000 ) ) ;
#2548=VECTOR ( 'NONE', #15134, 1000.000000000000000 ) ;
#2549=FACE_BOUND ( 'NONE', #1042, .T. ) ;
#2551=FACE_OUTER_BOUND ( 'NONE', #3271, .T. ) ;
#2552=CARTESIAN_POINT ( 'NONE',  ( -13.57909544900000043, -18.87168146910000033, 20.35758746379999806 ) ) ;
#2555=FACE_OUTER_BOUND ( 'NONE', #3581, .T. ) ;
#2556=AXIS2_PLACEMENT_3D ( 'NONE', #19032, #25321, #16843 ) ;
#2558=DIRECTION ( 'NONE',  ( 1.000000000000000000, 0.000000000000000000, 9.436895709310000674E-16 ) ) ;
#2559=ORIENTED_EDGE ( 'NONE', *, *, #23576, .T. ) ;
#2562=CIRCLE ( 'NONE', #18847, 3.750000000000000000 ) ;
#2564=ORIENTED_EDGE ( 'NONE', *, *, #12606, .T. ) ;
#2566=CARTESIAN_POINT ( 'NONE',  ( -11.20999108620000051, -59.03959220630000004, 20.55796391140000168 ) ) ;
#2567=CARTESIAN_POINT ( 'NONE',  ( -10.37698671729999766, -80.00000000000000000, 42.77322331710000469 ) ) ;
#2569=CARTESIAN_POINT ( 'NONE',  ( -40.00000000000000000, -84.50000000000000000, 6.883382752679998869E-16 ) ) ;
#2570=CARTESIAN_POINT ( 'NONE',  ( 20.68428921539999976, -36.00000000000000000, -9.307966650710000067 ) ) ;
#2571=CARTESIAN_POINT ( 'NONE',  ( -6.306066779869998999E-15, -74.00000000000000000, -2.597921877619999821E-15 ) ) ;
#2572=CYLINDRICAL_SURFACE ( 'NONE', #22474, 1.000000000000000888 ) ;
#2574=CARTESIAN_POINT ( 'NONE',  ( -7.215414233289999757, -74.50000000000000000, -40.70731707320000226 ) ) ;
#2581=ADVANCED_FACE ( 'NONE', ( #14932 ), #27566, .T. ) ;
#2584=CARTESIAN_POINT ( 'NONE',  ( -11.77695074595358804, -64.47177034477923030, -23.22164032104561571 ) ) ;
#2587=CARTESIAN_POINT ( 'NONE',  ( 19.76788193120000159, -18.85499412049999890, 9.715484483839999186 ) ) ;
#2588=CARTESIAN_POINT ( 'NONE',  ( 7.727575544279999598, -65.07443709589999514, -23.93310889699999677 ) ) ;
#2591=CARTESIAN_POINT ( 'NONE',  ( -11.88137749259999865, -72.18745160699998564, -26.31958153910000320 ) ) ;
#2595=CARTESIAN_POINT ( 'NONE',  ( 7.120909764619999412E-15, -74.00000000000000000, 40.00000000000000000 ) ) ;
#2598=LINE ( 'NONE', #20061, #20520 ) ;
#2600=CARTESIAN_POINT ( 'NONE',  ( 20.63161943080000071, -19.46510050319999863, -7.734358783100000245 ) ) ;
#2608=CARTESIAN_POINT ( 'NONE',  ( 47.19280742699999820, -74.66666680390001432, -1.149945984370000174 ) ) ;
#2611=CARTESIAN_POINT ( 'NONE',  ( -21.60034897659999942, -79.81702851609999527, -32.77174746360000057 ) ) ;
#2612=CARTESIAN_POINT ( 'NONE',  ( -13.24831469989999988, -74.00000000000000000, 34.75169505839999573 ) ) ;
#2613=EDGE_CURVE ( 'NONE', #2654, #21728, #2421, .T. ) ;
#2617=EDGE_CURVE ( 'NONE', #24085, #5350, #6294, .T. ) ;
#2618=CARTESIAN_POINT ( 'NONE',  ( 36.22844186549999534, -74.00000000000000000, -13.75000000000000000 ) ) ;
#2621=CARTESIAN_POINT ( 'NONE',  ( -38.70548889989999708, -73.81415926540000783, 7.196178079599999222 ) ) ;
#2622=CARTESIAN_POINT ( 'NONE',  ( -21.99725903910000113, -74.00000000020000357, -32.02260505910000177 ) ) ;
#2624=LINE ( 'NONE', #25351, #26929 ) ;
#2626=CARTESIAN_POINT ( 'NONE',  ( -7.383625343918562400, -73.99964414703678983, 39.24706873604019819 ) ) ;
#2627=CARTESIAN_POINT ( 'NONE',  ( 5.789150354839999823E-15, -69.50000000000000000, 32.75000000000000000 ) ) ;
#2630=DIRECTION ( 'NONE',  ( 0.000000000000000000, 1.000000000000000000, 0.000000000000000000 ) ) ;
#2631=CARTESIAN_POINT ( 'NONE',  ( 21.03973548180000108, -61.88564085890000399, 11.46780196789999984 ) ) ;
#2632=CARTESIAN_POINT ( 'NONE',  ( 1.421085471519999843E-14, -69.00000000000000000, 33.25000000000000000 ) ) ;
#2634=CARTESIAN_POINT ( 'NONE',  ( -40.70731707320000226, -77.00000000000000000, -7.215414233289999757 ) ) ;
#2636=FACE_OUTER_BOUND ( 'NONE', #22744, .T. ) ;
#2638=CARTESIAN_POINT ( 'NONE',  ( -11.97719338340000128, -64.78279197330000727, -22.48401985850000173 ) ) ;
#2641=VERTEX_POINT ( 'NONE', #3462 ) ;
#2642=CARTESIAN_POINT ( 'NONE',  ( -32.20769385759999892, -80.50000045429999318, -22.43272066369999962 ) ) ;
#2645=CARTESIAN_POINT ( 'NONE',  ( -14.40572000550000098, -18.50000000000000000, 20.06574520719999910 ) ) ;
#2647=EDGE_LOOP ( 'NONE', ( #5849, #24143, #22261, #1283 ) ) ;
#2652=CARTESIAN_POINT ( 'NONE',  ( -10.84063885470000166, -18.87168159810000034, -21.93863571940000057 ) ) ;
#2654=VERTEX_POINT ( 'NONE', #21236 ) ;
#2657=DIRECTION ( 'NONE',  ( 1.000000000000000000, 0.000000000000000000, 0.000000000000000000 ) ) ;
#2658=CARTESIAN_POINT ( 'NONE',  ( 39.90536558136047773, -73.91587151461750693, 7.249694362032179207 ) ) ;
#2663=EDGE_LOOP ( 'NONE', ( #28748, #23889, #24650, #12109, #9724 ) ) ;
#2665=CARTESIAN_POINT ( 'NONE',  ( 36.87753886209557663, -80.23900670806611402, -13.59568402046754976 ) ) ;
#2666=CARTESIAN_POINT ( 'NONE',  ( -19.81272040990000249, -52.63293862049999916, 12.05498172269999912 ) ) ;
#2667=DIRECTION ( 'NONE',  ( 1.000000000000000000, 0.000000000000000000, 0.000000000000000000 ) ) ;
#2668=CARTESIAN_POINT ( 'NONE',  ( 32.04416956680000084, -73.81489368219999392, -20.33277479140000210 ) ) ;
#2675=FACE_OUTER_BOUND ( 'NONE', #1727, .T. ) ;
#2677=B_SPLINE_SURFACE_WITH_KNOTS ( 'NONE', 5, 5, ( 
 ( #2173, #2618, #19781, #28802, #28662, #8695 ),
 ( #17611, #24312, #4351, #13224, #27088, #14114 ),
 ( #883, #27677, #442, #23289, #7130, #7577 ),
 ( #13963, #743, #27379, #9588, #15996, #11468 ),
 ( #18194, #18638, #25474, #2908, #11616, #9292 ),
 ( #24902, #25344, #4932, #18488, #16138, #18785 ) ),
 .UNSPECIFIED., .F., .F., .F.,
 ( 6, 6 ),
 ( 6, 6 ),
 ( 0.000000000000000000, 1.940837277319999998 ),
 ( 0.000000000000000000, 0.5000000000000000000 ),
 .UNSPECIFIED. ) ;
#2678=CARTESIAN_POINT ( 'NONE',  ( 24.39713799250000292, -19.50000027030000282, 1.459766484860000046 ) ) ;
#2679=CARTESIAN_POINT ( 'NONE',  ( 26.82296289428647285, -72.69303614417458448, -10.31361415116993641 ) ) ;
#2681=CARTESIAN_POINT ( 'NONE',  ( 9.320854954070000531, -36.00000000000000000, -20.33059790500000119 ) ) ;
#2682=CARTESIAN_POINT ( 'NONE',  ( 8.935678578700709807, -19.49096733334448928, -19.40207715605563266 ) ) ;
#2685=EDGE_CURVE ( 'NONE', #23505, #18491, #15682, .T. ) ;
#2686=VECTOR ( 'NONE', #6161, 1000.000000000000000 ) ;
#2690=CARTESIAN_POINT ( 'NONE',  ( -14.65665286289999969, -74.43375220249998847, 36.94583910070000599 ) ) ;
#2692=CARTESIAN_POINT ( 'NONE',  ( -1.179190554560000104, -39.36414254499999288, -22.77357817330000245 ) ) ;
#2698=DIRECTION ( 'NONE',  ( 0.000000000000000000, 1.000000000000000000, 0.000000000000000000 ) ) ;
#2700=ORIENTED_EDGE ( 'NONE', *, *, #28663, .F. ) ;
#2701=CARTESIAN_POINT ( 'NONE',  ( 36.24656976640000039, -75.00000018780001199, -15.05817680799999891 ) ) ;
#2702=CARTESIAN_POINT ( 'NONE',  ( -22.22906643760000023, -79.50000000000000000, -32.83566815539999340 ) ) ;
#2704=CIRCLE ( 'NONE', #25495, 3.499999999999999556 ) ;
#2705=CARTESIAN_POINT ( 'NONE',  ( -13.80673513500000027, -68.20222042139999985, 22.71145972000000057 ) ) ;
#2707=CARTESIAN_POINT ( 'NONE',  ( -13.26199019340000085, -58.91587053549999808, 20.59544867430000181 ) ) ;
#2710=CARTESIAN_POINT ( 'NONE',  ( 20.06309461859999743, -36.00000000000000000, -9.476129726630000860 ) ) ;
#2713=CARTESIAN_POINT ( 'NONE',  ( -11.23228026081345199, -39.24428776201335722, -22.24512021485102053 ) ) ;
#2715=CARTESIAN_POINT ( 'NONE',  ( 28.41585885021854097, -74.42752580149716835, -27.07206850168904566 ) ) ;
#2720=ORIENTED_EDGE ( 'NONE', *, *, #8478, .T. ) ;
#2724=CARTESIAN_POINT ( 'NONE',  ( -12.43380386931423232, -65.01950801014830006, -21.83872194420420598 ) ) ;
#2725=CARTESIAN_POINT ( 'NONE',  ( 40.00000000000000000, -74.00000000000000000, 2.009834509230000106E-15 ) ) ;
#2727=CARTESIAN_POINT ( 'NONE',  ( -21.40239531899999648, -66.04426305559999832, 14.04033265860000057 ) ) ;
#2731=CARTESIAN_POINT ( 'NONE',  ( -11.98650081279999924, -70.39409877170000129, -25.90118300180000332 ) ) ;
#2732=DIRECTION ( 'NONE',  ( 0.000000000000000000, -1.000000000000000000, 0.000000000000000000 ) ) ;
#2735=CARTESIAN_POINT ( 'NONE',  ( -39.03038279190000281, -74.00032110560000831, -7.562806955070000114 ) ) ;
#2745=TOROIDAL_SURFACE ( 'NONE', #23653, 13.00000000000000000, 2.000000000000000000 ) ;
#2747=DIRECTION ( 'NONE',  ( 1.000000000000000000, 0.000000000000000000, 0.000000000000000000 ) ) ;
#2749=CARTESIAN_POINT ( 'NONE',  ( 9.988478739970000575, -36.00000000000000000, -20.41376899180000137 ) ) ;
#2751=CARTESIAN_POINT ( 'NONE',  ( 7.225850277544148881, -73.65029154561577229, -39.40310785672224370 ) ) ;
#2754=CARTESIAN_POINT ( 'NONE',  ( -4.085206522429999154, -70.99734270939998737, -28.45162464230000054 ) ) ;
#2755=CARTESIAN_POINT ( 'NONE',  ( 22.26662627820000040, -57.47855601759999900, -7.066909182079999852 ) ) ;
#2756=CARTESIAN_POINT ( 'NONE',  ( -22.11864956829469619, -74.07080536734231657, -32.38124336146950810 ) ) ;
#2758=CARTESIAN_POINT ( 'NONE',  ( -14.78710422270000002, -79.49999982573447710, 36.35833235879999847 ) ) ;
#2759=CARTESIAN_POINT ( 'NONE',  ( -2.694596519430000559, -63.24129318349999807, -26.04567641519999910 ) ) ;
#2760=CARTESIAN_POINT ( 'NONE',  ( -22.10393671050000108, -74.26505820949999759, -32.64452500950000058 ) ) ;
#2761=ORIENTED_EDGE ( 'NONE', *, *, #3818, .F. ) ;
#2762=AXIS2_PLACEMENT_3D ( 'NONE', #3121, #7492, #11972 ) ;
#2764=CARTESIAN_POINT ( 'NONE',  ( -2.619606055569999814, -19.50000000000000000, -24.29997775220000023 ) ) ;
#2765=FACE_OUTER_BOUND ( 'NONE', #13647, .T. ) ;
#2766=ORIENTED_EDGE ( 'NONE', *, *, #12031, .T. ) ;
#2767=AXIS2_PLACEMENT_3D ( 'NONE', #16696, #12175, #1554 ) ;
#2771=CARTESIAN_POINT ( 'NONE',  ( 21.85294459619999685, -62.89113864609998927, 10.91972205250000094 ) ) ;
#2772=CARTESIAN_POINT ( 'NONE',  ( 8.988163966810001071, -35.02801756110000042, -19.45347226109999994 ) ) ;
#2776=CARTESIAN_POINT ( 'NONE',  ( 47.25000000000000000, -79.00000000000000000, -7.709388683000000122E-13 ) ) ;
#2777=CARTESIAN_POINT ( 'NONE',  ( -11.24280342539999822, -58.88258727490000410, -22.09277839770000185 ) ) ;
#2778=CARTESIAN_POINT ( 'NONE',  ( 36.90870977912933881, -79.74033897581968233, -14.42227066965258686 ) ) ;
#2779=CARTESIAN_POINT ( 'NONE',  ( 23.93312032140000056, -65.07443051799999978, -7.727578354849999442 ) ) ;
#2782=ORIENTED_EDGE ( 'NONE', *, *, #7608, .F. ) ;
#2785=AXIS2_PLACEMENT_3D ( 'NONE', #26617, #12312, #27917 ) ;
#2786=VERTEX_POINT ( 'NONE', #28768 ) ;
#2787=CARTESIAN_POINT ( 'NONE',  ( -13.53260628059999959, -42.21390124650000075, 20.62898559450000135 ) ) ;
#2790=VERTEX_POINT ( 'NONE', #26461 ) ;
#2792=ADVANCED_FACE ( 'NONE', ( #8662 ), #22448, .T. ) ;
#2795=CARTESIAN_POINT ( 'NONE',  ( -11.02010494672524388, -19.46474609920444365, -19.15837582207361933 ) ) ;
#2798=CARTESIAN_POINT ( 'NONE',  ( 21.79230230059999940, -37.95144147500000287, -8.472395268590000583 ) ) ;
#2800=CARTESIAN_POINT ( 'NONE',  ( -32.66023292159999869, -79.72849242800000980, -21.85457041760000152 ) ) ;
#2805=CARTESIAN_POINT ( 'NONE',  ( 7.120909764619999412E-15, -69.50000000000000000, 40.00000000000000000 ) ) ;
#2807=DIRECTION ( 'NONE',  ( 0.000000000000000000, -1.000000000000000000, 0.000000000000000000 ) ) ;
#2808=ORIENTED_EDGE ( 'NONE', *, *, #5850, .F. ) ;
#2810=CARTESIAN_POINT ( 'NONE',  ( -19.49041480450000208, -52.62618816490000029, 12.93508487010000074 ) ) ;
#2811=LINE ( 'NONE', #27586, #27757 ) ;
#2812=CARTESIAN_POINT ( 'NONE',  ( -20.30440251868529700, -57.41946960321629234, 14.68517168904920567 ) ) ;
#2815=CARTESIAN_POINT ( 'NONE',  ( 25.27264777759999959, -64.89165752090001149, 0.6762964727910000251 ) ) ;
#2818=CARTESIAN_POINT ( 'NONE',  ( 40.00000000000000000, -69.50000000000000000, 5.786765616290000531E-15 ) ) ;
#2821=CARTESIAN_POINT ( 'NONE',  ( 7.627568735119999666, -74.00000000000000000, 38.62788659690000515 ) ) ;
#2823=ADVANCED_FACE ( 'NONE', ( #10686 ), #10972, .T. ) ;
#2827=CARTESIAN_POINT ( 'NONE',  ( 9.165577939120000295, -36.05978003129999365, -20.59810505469999953 ) ) ;
#2830=ORIENTED_EDGE ( 'NONE', *, *, #21482, .F. ) ;
#2831=CARTESIAN_POINT ( 'NONE',  ( -40.12703402703129285, -74.06318173156705598, 7.249276399910129953 ) ) ;
#2832=AXIS2_PLACEMENT_3D ( 'NONE', #21321, #8470, #14880 ) ;
#2836=CARTESIAN_POINT ( 'NONE',  ( -1.464217970924556633, -19.46608320369988121, -22.20330980833862355 ) ) ;
#2837=B_SPLINE_CURVE_WITH_KNOTS ( 'NONE', 5,
 ( #18047, #25044, #22427, #22868, #11469, #15698, #24604, #2759, #27236, #22271, #9142, #18195 ),
 .UNSPECIFIED., .F., .F.,
 ( 6, 3, 3, 6 ),
 ( 112.4516934179999907, 115.4092999559999981, 122.7593676420000008, 122.9563471680000077 ),
 .UNSPECIFIED. ) ;
#2839=CARTESIAN_POINT ( 'NONE',  ( -1.456904695350000001, -52.62618816490000029, -23.34673678599999747 ) ) ;
#2841=FACE_OUTER_BOUND ( 'NONE', #1817, .T. ) ;
#2842=CARTESIAN_POINT ( 'NONE',  ( 22.12830645909999916, -53.29680639610000270, -7.019998623859999398 ) ) ;
#2843=CARTESIAN_POINT ( 'NONE',  ( 8.986258419809999509, -35.50000000000000000, -19.49544308430000328 ) ) ;
#2846=CARTESIAN_POINT ( 'NONE',  ( 36.59060393619999729, -74.92841728889999331, -14.75000109939999859 ) ) ;
#2847=FACE_OUTER_BOUND ( 'NONE', #15652, .T. ) ;
#2848=CARTESIAN_POINT ( 'NONE',  ( -22.65559868730312942, -80.00000000000000000, -32.64705978834439293 ) ) ;
#2849=EDGE_CURVE ( 'NONE', #2022, #9163, #13594, .T. ) ;
#2850=AXIS2_PLACEMENT_3D ( 'NONE', #18388, #25384, #12095 ) ;
#2851=CIRCLE ( 'NONE', #25193, 7.249999999999999112 ) ;
#2853=AXIS2_PLACEMENT_3D ( 'NONE', #7526, #6256, #12936 ) ;
#2855=CARTESIAN_POINT ( 'NONE',  ( 20.91697839109999890, -35.19239095940000084, -8.427788642599999491 ) ) ;
#2857=FACE_OUTER_BOUND ( 'NONE', #24929, .T. ) ;
#2860=EDGE_CURVE ( 'NONE', #9320, #26317, #4770, .T. ) ;
#2866=ORIENTED_EDGE ( 'NONE', *, *, #14425, .T. ) ;
#2868=VERTEX_POINT ( 'NONE', #27195 ) ;
#2871=LINE ( 'NONE', #16250, #15503 ) ;
#2872=AXIS2_PLACEMENT_3D ( 'NONE', #1782, #4683, #6875 ) ;
#2873=B_SPLINE_CURVE_WITH_KNOTS ( 'NONE', 5,
 ( #2166, #8990, #17897, #4190, #17460, #19915 ),
 .UNSPECIFIED., .F., .F.,
 ( 6, 6 ),
 ( 0.000000000000000000, 1.000000000000000000 ),
 .UNSPECIFIED. ) ;
#2874=CARTESIAN_POINT ( 'NONE',  ( -7.230541818644482532, -73.67850591084784639, -39.46631086812988087 ) ) ;
#2876=AXIS2_PLACEMENT_3D ( 'NONE', #24730, #9264, #2732 ) ;
#2877=CARTESIAN_POINT ( 'NONE',  ( -14.90631076309999870, -74.36723410090000641, 36.29697133340000192 ) ) ;
#2878=CARTESIAN_POINT ( 'NONE',  ( -21.78892497420000041, -67.75971617740000852, 15.66234658180000139 ) ) ;
#2881=CARTESIAN_POINT ( 'NONE',  ( -12.01481558839999941, -71.12613788880000243, -25.81978417510000057 ) ) ;
#2883=DIRECTION ( 'NONE',  ( -0.6710129359900831592, 0.000000000000000000, 0.7414456417930908039 ) ) ;
#2886=ORIENTED_EDGE ( 'NONE', *, *, #16918, .F. ) ;
#2888=EDGE_CURVE ( 'NONE', #8967, #13063, #20564, .T. ) ;
#2889=CARTESIAN_POINT ( 'NONE',  ( -2.584575094209999868, -57.80430419099999995, -25.24242492149999961 ) ) ;
#2890=B_SPLINE_CURVE_WITH_KNOTS ( 'NONE', 3,
 ( #16132, #7709, #16576, #25470, #437, #16431, #12048, #13956, #18629, #9285, #20814, #5067, #733, #9582, #2902, #586, #25033, #11760, #15989, #5223, #18483, #9431, #11608, #7414, #18186, #23283, #5501, #11908, #16277 ),
 .UNSPECIFIED., .F., .F.,
 ( 4, 2, 2, 2, 1, 1, 1, 1, 2, 2, 2, 2, 1, 1, 1, 2, 2, 4 ),
 ( 0.000000000000000000, 0.2500000000000724976, 0.3750000000001087463, 0.4375000000001268985, 0.4687500000001376677, 0.4843750000001449396, 0.4921875000001469935, 0.4960937500001482703, 0.4980468750001488254, 0.5000000000001494360, 0.6250000000001784128, 0.6875000000001919576, 0.7187500000001986189, 0.7343750000002017275, 0.7421875000002008393, 0.7460937500002003953, 0.7500000000001999512, 1.000000000000000000 ),
 .UNSPECIFIED. ) ;
#2892=EDGE_CURVE ( 'NONE', #24483, #24085, #19173, .T. ) ;
#2895=CIRCLE ( 'NONE', #14053, 7.249999999999999112 ) ;
#2898=CARTESIAN_POINT ( 'NONE',  ( 20.87140401170000104, -36.00000000000000000, -10.07774184699999864 ) ) ;
#2899=CARTESIAN_POINT ( 'NONE',  ( 47.18156435510000080, -74.63486761890000309, -1.134764142530000131 ) ) ;
#2901=CARTESIAN_POINT ( 'NONE',  ( 7.213678002751584550, -73.60295742109886419, -39.27497438193323376 ) ) ;
#2902=CARTESIAN_POINT ( 'NONE',  ( -11.45632417142031301, -61.34567075806889846, 20.94901889759627522 ) ) ;
#2903=ORIENTED_EDGE ( 'NONE', *, *, #24675, .T. ) ;
#2905=CARTESIAN_POINT ( 'NONE',  ( -3.852920966090000121, -71.18862645909999287, -28.24098550969999977 ) ) ;
#2908=CARTESIAN_POINT ( 'NONE',  ( 36.47365836190000010, -74.39700102820000893, -14.67944147449999903 ) ) ;
#2910=CARTESIAN_POINT ( 'NONE',  ( 25.80868167070000396, -64.58097566740001128, 1.225860731590000086 ) ) ;
#2911=CARTESIAN_POINT ( 'NONE',  ( -22.03141727930000116, -74.00000000000000000, -32.02573219850000186 ) ) ;
#2913=ORIENTED_EDGE ( 'NONE', *, *, #11565, .F. ) ;
#2915=CARTESIAN_POINT ( 'NONE',  ( -7.366413754511537348, -73.99967301548019805, 39.30374743330985154 ) ) ;
#2916=CARTESIAN_POINT ( 'NONE',  ( 36.75354318842512669, -74.46086523469682561, -14.59276404010832628 ) ) ;
#2918=CYLINDRICAL_SURFACE ( 'NONE', #12769, 32.39999999999999858 ) ;
#2919=DIRECTION ( 'NONE',  ( 0.9408310772095872521, 0.000000000000000000, 0.3388759126238510833 ) ) ;
#2920=CARTESIAN_POINT ( 'NONE',  ( 8.988706506799999829, -34.85239680849999644, -19.44233762329999848 ) ) ;
#2924=CARTESIAN_POINT ( 'NONE',  ( 20.69873715099999956, -52.63055504180000099, 10.61298605969999898 ) ) ;
#2925=B_SPLINE_SURFACE_WITH_KNOTS ( 'NONE', 5, 5, ( 
 ( #12330, #21238, #12191, #21107, #879, #12459 ),
 ( #10131, #21372, #10275, #8109, #28074, #9720 ),
 ( #14253, #18630, #27528, #18778, #5504, #16434 ),
 ( #23144, #12049, #20965, #1024, #26176, #6050 ),
 ( #4017, #23836, #28631, #22094, #4158, #12603 ),
 ( #1847, #23697, #3739, #14796, #17571, #13031 ) ),
 .UNSPECIFIED., .F., .F., .F.,
 ( 6, 6 ),
 ( 6, 6 ),
 ( 2.618707526800000185, 4.366203223410000334 ),
 ( 0.000000000000000000, 0.5000000000000000000 ),
 .UNSPECIFIED. ) ;
#2927=CARTESIAN_POINT ( 'NONE',  ( -11.52017008789999863, -59.01533270489999694, -20.60511547919999842 ) ) ;
#2928=CARTESIAN_POINT ( 'NONE',  ( 37.14627454077874802, -79.96476207452478491, -14.01644017333399006 ) ) ;
#2929=FACE_OUTER_BOUND ( 'NONE', #6715, .T. ) ;
#2932=AXIS2_PLACEMENT_3D ( 'NONE', #23977, #8805, #22225 ) ;
#2933=CARTESIAN_POINT ( 'NONE',  ( 47.01173857123500710, -74.16368351650025659, -1.843492029084275785 ) ) ;
#2934=ORIENTED_EDGE ( 'NONE', *, *, #25396, .T. ) ;
#2935=CARTESIAN_POINT ( 'NONE',  ( -13.01278816429999985, -34.63361166290000170, 19.94379924919999780 ) ) ;
#2936=CARTESIAN_POINT ( 'NONE',  ( 9.024081099289999131, -19.49999992740000110, -18.94592230980000380 ) ) ;
#2937=ORIENTED_EDGE ( 'NONE', *, *, #4873, .T. ) ;
#2940=EDGE_LOOP ( 'NONE', ( #3507, #27405, #10044, #887 ) ) ;
#2941=CARTESIAN_POINT ( 'NONE',  ( -0.5413028987460000163, -57.47855601759999900, -23.35488904649999853 ) ) ;
#2942=CARTESIAN_POINT ( 'NONE',  ( -10.48084080227152626, -19.47282323712138208, -20.22219529147017880 ) ) ;
#2943=DIRECTION ( 'NONE',  ( 0.000000000000000000, -1.000000000000000000, 0.000000000000000000 ) ) ;
#2944=CARTESIAN_POINT ( 'NONE',  ( -9.684721259419999839, -18.50000000000000000, -20.79699324019999906 ) ) ;
#2945=CARTESIAN_POINT ( 'NONE',  ( 9.743056916871200457, -61.47481733543323656, -24.01218373186148369 ) ) ;
#2946=ORIENTED_EDGE ( 'NONE', *, *, #22702, .F. ) ;
#2947=CARTESIAN_POINT ( 'NONE',  ( -32.77174707999999725, -79.81706294759999309, -21.60034937969999902 ) ) ;
#2949=EDGE_CURVE ( 'NONE', #2641, #5527, #4546, .T. ) ;
#2951=VERTEX_POINT ( 'NONE', #2429 ) ;
#2954=DIRECTION ( 'NONE',  ( 0.2414462220490750377, 0.000000000000000000, 0.9704142011833034598 ) ) ;
#2961=B_SPLINE_CURVE_WITH_KNOTS ( 'NONE', 5,
 ( #3420, #9956, #3143, #18728, #14479, #11999 ),
 .UNSPECIFIED., .F., .F.,
 ( 6, 6 ),
 ( 0.000000000000000000, 1.000000000000000000 ),
 .UNSPECIFIED. ) ;
#2963=EDGE_CURVE ( 'NONE', #7997, #2790, #14065, .T. ) ;
#2964=CARTESIAN_POINT ( 'NONE',  ( 22.17287391929999885, -57.47832537019999677, -7.362282751269999537 ) ) ;
#2965=AXIS2_PLACEMENT_3D ( 'NONE', #21975, #15239, #6531 ) ;
#2967=CARTESIAN_POINT ( 'NONE',  ( 26.91262686989999864, -67.03347986180000362, 1.647007874590000087 ) ) ;
#2968=CARTESIAN_POINT ( 'NONE',  ( -10.54576762539999990, -18.85523517670000260, 19.18725863699999934 ) ) ;
#2970=FACE_OUTER_BOUND ( 'NONE', #7600, .T. ) ;
#2971=CARTESIAN_POINT ( 'NONE',  ( 21.70215820849999844, -37.32353051909999664, -8.471236736359999853 ) ) ;
#2973=ORIENTED_EDGE ( 'NONE', *, *, #20675, .T. ) ;
#2974=DIRECTION ( 'NONE',  ( 1.000000000000000000, 0.000000000000000000, 0.000000000000000000 ) ) ;
#2978=CARTESIAN_POINT ( 'NONE',  ( 26.90812271843742565, -72.79933240784657755, -9.897999932954709479 ) ) ;
#2983=CARTESIAN_POINT ( 'NONE',  ( -40.61475266853483390, -74.42768721757238382, 7.224488193796126723 ) ) ;
#2984=CARTESIAN_POINT ( 'NONE',  ( 38.08875739639999836, -84.00000000000000000, -9.476764215410000247 ) ) ;
#2987=CARTESIAN_POINT ( 'NONE',  ( -2.579071154395890630, -19.48685756504436384, -23.54263317592151594 ) ) ;
#2988=EDGE_CURVE ( 'NONE', #20659, #23734, #8921, .T. ) ;
#2990=CARTESIAN_POINT ( 'NONE',  ( -0.5335602090290000321, -52.63293862049999916, -23.18581005440000098 ) ) ;
#2993=CIRCLE ( 'NONE', #11392, 3.500000000000003109 ) ;
#2996=LINE ( 'NONE', #972, #19416 ) ;
#2997=CARTESIAN_POINT ( 'NONE',  ( 21.98941332889999956, -49.11505549560000361, -6.974892859150000568 ) ) ;
#2998=EDGE_CURVE ( 'NONE', #24745, #10596, #5470, .T. ) ;
#2999=DIRECTION ( 'NONE',  ( 0.000000000000000000, -1.000000000000000000, 0.000000000000000000 ) ) ;
#3000=DIRECTION ( 'NONE',  ( 1.000000000000000000, 0.000000000000000000, 0.000000000000000000 ) ) ;
#3002=EDGE_CURVE ( 'NONE', #4093, #8967, #20188, .T. ) ;
#3006=CARTESIAN_POINT ( 'NONE',  ( -14.08127054510000065, -65.97310055630001102, 21.99106896830000224 ) ) ;
#3007=CARTESIAN_POINT ( 'NONE',  ( 8.961089119540002201, -35.57149483869999784, -20.08449242119999667 ) ) ;
#3009=FACE_OUTER_BOUND ( 'NONE', #25888, .T. ) ;
#3010=CARTESIAN_POINT ( 'NONE',  ( 20.73064457619999956, -36.00000000000000000, -9.377114307539999416 ) ) ;
#3012=CIRCLE ( 'NONE', #6709, 0.5000000000000004441 ) ;
#3014=DIRECTION ( 'NONE',  ( 0.9212380119587632032, 0.000000000000000000, -0.3889993898738990930 ) ) ;
#3017=CARTESIAN_POINT ( 'NONE',  ( -32.70203577369999692, -80.13412001289999864, -21.70611439569999845 ) ) ;
#3030=EDGE_CURVE ( 'NONE', #7301, #26062, #17089, .T. ) ;
#3031=DIRECTION ( 'NONE',  ( 0.8086044598489942059, 0.000000000000000000, -0.5883526387399961033 ) ) ;
#3036=CARTESIAN_POINT ( 'NONE',  ( 8.508195433830001875, -34.61672952569999495, -20.76917450910000085 ) ) ;
#3038=LINE ( 'NONE', #3447, #27692 ) ;
#3041=EDGE_CURVE ( 'NONE', #22316, #26221, #12952, .T. ) ;
#3043=ORIENTED_EDGE ( 'NONE', *, *, #7541, .T. ) ;
#3044=FACE_OUTER_BOUND ( 'NONE', #17610, .T. ) ;
#3046=CARTESIAN_POINT ( 'NONE',  ( -11.35954001540000036, -74.50000000000000000, 45.25000000000000000 ) ) ;
#3048=VERTEX_POINT ( 'NONE', #3297 ) ;
#3049=CIRCLE ( 'NONE', #15089, 3.500000000000003109 ) ;
#3051=LINE ( 'NONE', #16128, #16794 ) ;
#3054=CARTESIAN_POINT ( 'NONE',  ( 7.233314584209180609, -74.35734738468387661, -40.52471375186235036 ) ) ;
#3056=VERTEX_POINT ( 'NONE', #12158 ) ;
#3059=CARTESIAN_POINT ( 'NONE',  ( -2.790529132629999687, -64.24504218810000111, -26.36014162090000212 ) ) ;
#3060=CARTESIAN_POINT ( 'NONE',  ( -16.10242507159999903, -71.49765472880000061, 23.35251611179999998 ) ) ;
#3061=ORIENTED_EDGE ( 'NONE', *, *, #3383, .T. ) ;
#3063=ADVANCED_FACE ( 'NONE', ( #7681 ), #1980, .T. ) ;
#3065=CARTESIAN_POINT ( 'NONE',  ( 23.60463849679999626, -59.01533270489999694, 0.3257977875450000504 ) ) ;
#3066=CARTESIAN_POINT ( 'NONE',  ( -21.01599529309999781, -64.93834962409999889, 13.98666844150000088 ) ) ;
#3067=EDGE_LOOP ( 'NONE', ( #22611, #6190, #7662, #12901 ) ) ;
#3068=CARTESIAN_POINT ( 'NONE',  ( -18.99800347089999875, -26.09861276229999660, 11.61132478269999879 ) ) ;
#3069=CARTESIAN_POINT ( 'NONE',  ( -0.9991794988550000145, -19.46390881170000142, -22.01488094909999660 ) ) ;
#3073=CARTESIAN_POINT ( 'NONE',  ( -11.74977568899999980, -18.50000000000000000, 18.05674360140000445 ) ) ;
#3074=TOROIDAL_SURFACE ( 'NONE', #19326, 30.50381168839999901, 2.000000000000000000 ) ;
#3075=CARTESIAN_POINT ( 'NONE',  ( 23.41692821889999720, -63.52052399810000338, 10.59810502480000061 ) ) ;
#3081=CARTESIAN_POINT ( 'NONE',  ( -11.18016241690000001, -57.44036991850000362, -21.74842387279999656 ) ) ;
#3084=ORIENTED_EDGE ( 'NONE', *, *, #4007, .F. ) ;
#3085=EDGE_CURVE ( 'NONE', #21366, #10298, #9835, .T. ) ;
#3088=CARTESIAN_POINT ( 'NONE',  ( -11.42167949289999918, -34.66886610320000273, 19.55066939339999976 ) ) ;
#3090=ORIENTED_EDGE ( 'NONE', *, *, #19002, .T. ) ;
#3091=CARTESIAN_POINT ( 'NONE',  ( 39.04162410880000067, -73.95638562439998509, 7.432628554209999905 ) ) ;
#3092=CARTESIAN_POINT ( 'NONE',  ( -10.71547162644561624, -19.46656777169255292, -19.55512608735946500 ) ) ;
#3093=CARTESIAN_POINT ( 'NONE',  ( 7.120909764619999412E-15, -74.50000000000000000, 40.00000000000000000 ) ) ;
#3094=CARTESIAN_POINT ( 'NONE',  ( -9.797255285709999484, -18.50000000000000000, -21.36865465820000054 ) ) ;
#3095=CARTESIAN_POINT ( 'NONE',  ( -10.20110288159999890, -84.50000000000000000, -41.00000000000000000 ) ) ;
#3096=ORIENTED_EDGE ( 'NONE', *, *, #19405, .F. ) ;
#3098=ADVANCED_FACE ( 'NONE', ( #27640 ), #5878, .T. ) ;
#3103=AXIS2_PLACEMENT_3D ( 'NONE', #23067, #23199, #2667 ) ;
#3105=CARTESIAN_POINT ( 'NONE',  ( 7.708049625630000179, -24.50935433020000076, -20.82960214859999937 ) ) ;
#3109=CARTESIAN_POINT ( 'NONE',  ( -19.45061163789999981, -45.99930305819999887, 12.20452280910000020 ) ) ;
#3110=CARTESIAN_POINT ( 'NONE',  ( 30.63102016379999881, -73.01580299129999219, -23.62320562749999908 ) ) ;
#3111=CARTESIAN_POINT ( 'NONE',  ( 22.38434844160000026, -60.58720252940000250, -7.752233810359999922 ) ) ;
#3112=CARTESIAN_POINT ( 'NONE',  ( 25.57917931149999902, -64.69849622489999774, 1.120748734570000016 ) ) ;
#3113=CARTESIAN_POINT ( 'NONE',  ( -10.60770804610000084, -19.15810967940000253, 19.29995473580000009 ) ) ;
#3114=EDGE_LOOP ( 'NONE', ( #25608, #26871, #2766, #14276 ) ) ;
#3116=CARTESIAN_POINT ( 'NONE',  ( -39.48689401896172768, -73.68677077079325954, -7.232334316218844705 ) ) ;
#3118=CARTESIAN_POINT ( 'NONE',  ( 21.72885701919999946, -37.62355108940000292, -8.376330313129999539 ) ) ;
#3120=VERTEX_POINT ( 'NONE', #21940 ) ;
#3121=CARTESIAN_POINT ( 'NONE',  ( 25.26718046270000073, -45.73899999920000425, 6.129403842640000377 ) ) ;
#3122=CARTESIAN_POINT ( 'NONE',  ( -10.89815191770000169, -18.50000000000000000, -17.99090140869999743 ) ) ;
#3124=CARTESIAN_POINT ( 'NONE',  ( 46.25000000000000000, -79.00000000000000000, -14.75000000000000000 ) ) ;
#3127=VERTEX_POINT ( 'NONE', #8374 ) ;
#3133=DIRECTION ( 'NONE',  ( 0.000000000000000000, -1.000000000000000000, 0.000000000000000000 ) ) ;
#3135=CARTESIAN_POINT ( 'NONE',  ( -0.5372044051000000042, -32.73130089789999886, -22.49056468509999718 ) ) ;
#3139=FACE_OUTER_BOUND ( 'NONE', #7188, .T. ) ;
#3141=VERTEX_POINT ( 'NONE', #22090 ) ;
#3143=CARTESIAN_POINT ( 'NONE',  ( -21.85457041760000152, -74.50000000000000000, -32.66023292159999869 ) ) ;
#3145=CARTESIAN_POINT ( 'NONE',  ( 8.744948820599999451, -35.57625659020000342, -20.62426134429999891 ) ) ;
#3146=DIRECTION ( 'NONE',  ( 1.000000000000000000, 0.000000000000000000, 0.000000000000000000 ) ) ;
#3148=CARTESIAN_POINT ( 'NONE',  ( 46.25000000000000000, -77.00000000000000000, -13.75000000000000000 ) ) ;
#3151=EDGE_CURVE ( 'NONE', #3865, #27292, #6633, .T. ) ;
#3153=ORIENTED_EDGE ( 'NONE', *, *, #15812, .T. ) ;
#3154=CARTESIAN_POINT ( 'NONE',  ( 32.73121282881579219, -74.00000011846343284, -20.86988175080205465 ) ) ;
#3156=ORIENTED_EDGE ( 'NONE', *, *, #5885, .F. ) ;
#3159=CARTESIAN_POINT ( 'NONE',  ( -10.20110288159999890, -74.00000000000000000, 41.00000000000000000 ) ) ;
#3161=ORIENTED_EDGE ( 'NONE', *, *, #15006, .F. ) ;
#3164=PLANE ( 'NONE',  #18309 ) ;
#3165=CARTESIAN_POINT ( 'NONE',  ( 21.89559254579999958, -72.72322124080000094, -31.02685804430000260 ) ) ;
#3166=FACE_OUTER_BOUND ( 'NONE', #20183, .T. ) ;
#3168=B_SPLINE_SURFACE_WITH_KNOTS ( 'NONE', 5, 5, ( 
 ( #4001, #21779, #1832, #10673, #8513, #20312 ),
 ( #5017, #24840, #26744, #13904, #383, #8937 ),
 ( #89, #18286, #27032, #9227, #13460, #534 ),
 ( #4879, #681, #9384, #7075, #18135, #4582 ),
 ( #6923, #2846, #11709, #22661, #15935, #20623 ),
 ( #22808, #17847, #16083, #6779, #15640, #2701 ) ),
 .UNSPECIFIED., .F., .F., .F.,
 ( 6, 6 ),
 ( 6, 6 ),
 ( 6.713731535029999975, 7.329014384030000606 ),
 ( 0.000000000000000000, 0.5000000000000000000 ),
 .UNSPECIFIED. ) ;
#3169=CARTESIAN_POINT ( 'NONE',  ( -12.09704001540000107, -80.00000000000000000, 47.10905722069999513 ) ) ;
#3170=CARTESIAN_POINT ( 'NONE',  ( 8.509522500270000123, -31.58327295760000197, -20.65664638119999807 ) ) ;
#3171=CARTESIAN_POINT ( 'NONE',  ( 23.14416696340000001, -57.40875702419999982, 10.37855830930000067 ) ) ;
#3173=EDGE_LOOP ( 'NONE', ( #4142, #13134, #23756, #10527 ) ) ;
#3174=AXIS2_PLACEMENT_3D ( 'NONE', #20082, #26799, #13669 ) ;
#3177=CARTESIAN_POINT ( 'NONE',  ( -2.488381974000000163, -57.43018231299999599, -24.62424122550000050 ) ) ;
#3180=EDGE_LOOP ( 'NONE', ( #12404, #27489, #3986, #18825 ) ) ;
#3182=CARTESIAN_POINT ( 'NONE',  ( -7.627568735119999666, -74.00000000000000000, 38.62788659690000515 ) ) ;
#3188=EDGE_CURVE ( 'NONE', #7412, #13154, #5090, .T. ) ;
#3192=CIRCLE ( 'NONE', #19444, 0.5000000000000013323 ) ;
#3193=CARTESIAN_POINT ( 'NONE',  ( -3.058911596290000201, -72.82938648530000592, -28.52031795890000154 ) ) ;
#3194=CARTESIAN_POINT ( 'NONE',  ( -16.01432518160000029, -72.70510571239999820, 23.73092384619999962 ) ) ;
#3198=CARTESIAN_POINT ( 'NONE',  ( -20.15147649909999927, -62.06884231739999791, 13.30139272559999952 ) ) ;
#3201=CARTESIAN_POINT ( 'NONE',  ( -0.5567007213574344249, -26.09861274200153147, -22.25841601198301944 ) ) ;
#3202=CARTESIAN_POINT ( 'NONE',  ( -2.650567523169999884, -19.17792668139999890, -23.73795088580000012 ) ) ;
#3204=ORIENTED_EDGE ( 'NONE', *, *, #6439, .F. ) ;
#3205=CYLINDRICAL_SURFACE ( 'NONE', #16537, 10.00000000000000000 ) ;
#3206=B_SPLINE_CURVE_WITH_KNOTS ( 'NONE', 3,
 ( #15249, #11473, #22725, #11775 ),
 .UNSPECIFIED., .F., .F.,
 ( 4, 4 ),
 ( 0.000000000000000000, 1.000000000000000000 ),
 .UNSPECIFIED. ) ;
#3209=CARTESIAN_POINT ( 'NONE',  ( -4.234949299205656992, -72.18744871743631109, -28.56489076017935957 ) ) ;
#3210=VERTEX_POINT ( 'NONE', #14069 ) ;
#3213=CARTESIAN_POINT ( 'NONE',  ( 26.16632615330000178, -71.08692331999999681, -10.19695628250000041 ) ) ;
#3214=FACE_OUTER_BOUND ( 'NONE', #27610, .T. ) ;
#3215=ORIENTED_EDGE ( 'NONE', *, *, #2210, .T. ) ;
#3216=EDGE_CURVE ( 'NONE', #26221, #16034, #5553, .T. ) ;
#3218=CARTESIAN_POINT ( 'NONE',  ( 47.16974535660000356, -74.50000000000000000, -1.075756255579999987 ) ) ;
#3219=ORIENTED_EDGE ( 'NONE', *, *, #6343, .T. ) ;
#3220=FACE_OUTER_BOUND ( 'NONE', #17799, .T. ) ;
#3224=CARTESIAN_POINT ( 'NONE',  ( 46.12332288628675769, -80.00000000113583098, -4.489694476353789376 ) ) ;
#3225=LINE ( 'NONE', #9472, #4301 ) ;
#3229=CARTESIAN_POINT ( 'NONE',  ( -10.51533464487888736, -19.47102514969543208, -20.05824860045767721 ) ) ;
#3230=DIRECTION ( 'NONE',  ( 1.000000000000000000, 0.000000000000000000, 0.000000000000000000 ) ) ;
#3231=CARTESIAN_POINT ( 'NONE',  ( 9.476764215410000247, -82.25000000000000000, 38.08875739639999836 ) ) ;
#3232=LINE ( 'NONE', #12091, #14814 ) ;
#3233=VERTEX_POINT ( 'NONE', #7804 ) ;
#3235=AXIS2_PLACEMENT_3D ( 'NONE', #3169, #9697, #15967 ) ;
#3236=CARTESIAN_POINT ( 'NONE',  ( -32.66023292159999869, -79.50000000000000000, -21.85457041760000152 ) ) ;
#3238=FACE_OUTER_BOUND ( 'NONE', #3114, .T. ) ;
#3239=ORIENTED_EDGE ( 'NONE', *, *, #14018, .F. ) ;
#3241=CARTESIAN_POINT ( 'NONE',  ( -14.87113501819999861, -65.53648121479999133, 22.45123099050000093 ) ) ;
#3242=ORIENTED_EDGE ( 'NONE', *, *, #10014, .T. ) ;
#3245=CARTESIAN_POINT ( 'NONE',  ( -19.89280855559999850, -39.30675845289999870, 14.46928939670000069 ) ) ;
#3247=CARTESIAN_POINT ( 'NONE',  ( 28.93927510940000047, -73.97465399030001265, -26.57194658529999742 ) ) ;
#3248=DIRECTION ( 'NONE',  ( 0.000000000000000000, -1.000000000000000000, 0.000000000000000000 ) ) ;
#3249=CARTESIAN_POINT ( 'NONE',  ( 25.82503148889999878, -66.16381828919999464, 0.7716244649270000977 ) ) ;
#3255=EDGE_CURVE ( 'NONE', #14724, #23155, #12041, .T. ) ;
#3257=B_SPLINE_CURVE_WITH_KNOTS ( 'NONE', 5,
 ( #24158, #22264, #8838, #17755, #26637, #4486, #13359, #27370, #20517 ),
 .UNSPECIFIED., .F., .F.,
 ( 6, 3, 6 ),
 ( 0.000000000000000000, 0.5000000000000000000, 1.000000000000000000 ),
 .UNSPECIFIED. ) ;
#3258=CARTESIAN_POINT ( 'NONE',  ( 21.61390653610000001, -37.84383064499999705, -8.096276181549999507 ) ) ;
#3260=ORIENTED_EDGE ( 'NONE', *, *, #25866, .F. ) ;
#3261=CARTESIAN_POINT ( 'NONE',  ( 7.973708284010000646, -18.50000000000000000, -19.11504000820000115 ) ) ;
#3264=B_SPLINE_CURVE_WITH_KNOTS ( 'NONE', 3,
 ( #13402, #32, #631, #18384, #17793, #4387, #13256, #22307, #22163, #26683, #2353, #5408, #11808, #14560, #23466, #14291, #21144, #27574, #25650, #27833, #14001, #9763, #23187, #1200, #7613, #16755, #10035, #16477, #1066, #18949, #18525, #7873, #25238, #25084, #20720, #5680, #779, #7467 ),
 .UNSPECIFIED., .F., .F.,
 ( 4, 2, 2, 1, 1, 1, 1, 2, 2, 2, 2, 1, 1, 1, 2, 2, 2, 2, 1, 1, 1, 2, 2, 4 ),
 ( 0.000000000000000000, 0.1250000000001522948, 0.1875000000002285672, 0.2187500000002666756, 0.2343750000002870482, 0.2421875000002955969, 0.2460937500003001766, 0.2480468750003007039, 0.2500000000003012590, 0.3750000000002757794, 0.4375000000002619571, 0.4687500000002539080, 0.4843750000002494671, 0.4921875000002482459, 0.4960937500002480793, 0.5000000000002479128, 0.6250000000002012834, 0.6875000000001786349, 0.7187500000001665335, 0.7343750000001604272, 0.7421875000001573186, 0.7460937500001556533, 0.7500000000001538769, 1.000000000000000000 ),
 .UNSPECIFIED. ) ;
#3265=CARTESIAN_POINT ( 'NONE',  ( 7.517162733169999278, -40.74985578699999422, -21.57753409760000096 ) ) ;
#3267=VERTEX_POINT ( 'NONE', #27767 ) ;
#3271=EDGE_LOOP ( 'NONE', ( #871, #11955, #12087, #3204 ) ) ;
#3272=CARTESIAN_POINT ( 'NONE',  ( -14.43678919070000077, -74.15747494800001505, 36.75078895099999698 ) ) ;
#3274=CARTESIAN_POINT ( 'NONE',  ( -2.483423092989999859, -26.06274386000000121, -23.44595030099999988 ) ) ;
#3277=DIRECTION ( 'NONE',  ( 1.000000000000000000, 0.000000000000000000, 0.000000000000000000 ) ) ;
#3280=CARTESIAN_POINT ( 'NONE',  ( 23.40924512820000203, -53.22700740269999642, -9.524618309619999224 ) ) ;
#3287=LINE ( 'NONE', #3422, #12145 ) ;
#3288=CARTESIAN_POINT ( 'NONE',  ( 7.310010114310000695, -36.32767552400000710, -21.47202530089999684 ) ) ;
#3290=CARTESIAN_POINT ( 'NONE',  ( -32.39999999999999858, -86.00000000000000000, 0.000000000000000000 ) ) ;
#3294=CARTESIAN_POINT ( 'NONE',  ( -2.555686511607881517, -71.82672801145491803, -28.11473483637883675 ) ) ;
#3295=DIRECTION ( 'NONE',  ( -0.7071067811865470176, 0.000000000000000000, -0.7071067811865480168 ) ) ;
#3297=CARTESIAN_POINT ( 'NONE',  ( -32.83566817450000030, -79.50000000000000000, -22.22906645670000003 ) ) ;
#3298=EDGE_LOOP ( 'NONE', ( #21641, #21966, #19805, #15161, #11151 ) ) ;
#3299=DIRECTION ( 'NONE',  ( 0.000000000000000000, 1.000000000000000000, 0.000000000000000000 ) ) ;
#3300=FACE_OUTER_BOUND ( 'NONE', #22997, .T. ) ;
#3303=CARTESIAN_POINT ( 'NONE',  ( 22.05228288849999885, -72.00360875399999827, -30.91980140109999553 ) ) ;
#3306=CARTESIAN_POINT ( 'NONE',  ( 8.804564246469999134, -31.59895619559999957, -20.26062780839999888 ) ) ;
#3307=CARTESIAN_POINT ( 'NONE',  ( -26.69328098980000163, -74.00000000000000000, -37.29988270759999835 ) ) ;
#3308=CARTESIAN_POINT ( 'NONE',  ( 4.882943008269999509E-15, -69.50000000000000000, -40.00000000000000000 ) ) ;
#3312=EDGE_CURVE ( 'NONE', #13063, #4330, #11124, .T. ) ;
#3315=ORIENTED_EDGE ( 'NONE', *, *, #11420, .F. ) ;
#3316=ADVANCED_FACE ( 'NONE', ( #1261 ), #10097, .T. ) ;
#3323=CARTESIAN_POINT ( 'NONE',  ( -7.561758309997661520, -74.02518802157268851, -38.96765197712468165 ) ) ;
#3324=ORIENTED_EDGE ( 'NONE', *, *, #7736, .T. ) ;
#3325=DIRECTION ( 'NONE',  ( -0.2414462220490755373, 0.000000000000000000, -0.9704142011833032377 ) ) ;
#3326=CARTESIAN_POINT ( 'NONE',  ( -17.94180966909999597, -19.50000000000000000, 18.81731824139999887 ) ) ;
#3334=CARTESIAN_POINT ( 'NONE',  ( 24.49010419710000264, -63.63799337820000090, -0.5178770050080000464 ) ) ;
#3335=CARTESIAN_POINT ( 'NONE',  ( 19.44161842069999935, -34.82993252660000394, -8.988741827920000205 ) ) ;
#3338=CARTESIAN_POINT ( 'NONE',  ( -2.326474588770000018, -19.16559685929999901, -22.80254021129999842 ) ) ;
#3340=ORIENTED_EDGE ( 'NONE', *, *, #25811, .T. ) ;
#3343=CARTESIAN_POINT ( 'NONE',  ( -31.89935321680000158, -74.00000000000000000, -21.99985828019999801 ) ) ;
#3344=CARTESIAN_POINT ( 'NONE',  ( -11.35954001540000036, -79.50000000000000000, 45.25000000000000000 ) ) ;
#3345=CARTESIAN_POINT ( 'NONE',  ( -1.776356839399999804E-15, -89.00000000000000000, 0.000000000000000000 ) ) ;
#3347=EDGE_CURVE ( 'NONE', #5424, #7860, #11069, .T. ) ;
#3348=AXIS2_PLACEMENT_3D ( 'NONE', #28430, #5992, #14872 ) ;
#3353=CARTESIAN_POINT ( 'NONE',  ( -1.767871301636886550, -80.14255480913817564, 47.03116330652069621 ) ) ;
#3356=EDGE_LOOP ( 'NONE', ( #12342, #23781 ) ) ;
#3357=DIRECTION ( 'NONE',  ( -0.5301416321220548955, 0.000000000000000000, -0.8479091047340887588 ) ) ;
#3359=ORIENTED_EDGE ( 'NONE', *, *, #8938, .F. ) ;
#3360=CARTESIAN_POINT ( 'NONE',  ( -21.35786096709999882, -65.07443093669999712, 13.27975207949999970 ) ) ;
#3364=CARTESIAN_POINT ( 'NONE',  ( 25.61850624154103073, -69.24211324756858232, -8.680134436598166303 ) ) ;
#3366=AXIS2_PLACEMENT_3D ( 'NONE', #11334, #20533, #26505 ) ;
#3367=CARTESIAN_POINT ( 'NONE',  ( 9.755293273557064992, -61.61770146517354618, -24.04309117867698475 ) ) ;
#3369=CARTESIAN_POINT ( 'NONE',  ( -32.80949674840000085, -79.81706281630000888, -22.29175087539999822 ) ) ;
#3372=CARTESIAN_POINT ( 'NONE',  ( 9.334872109610000362E-16, -74.00000000000000000, -2.419703924680000090E-15 ) ) ;
#3376=LINE ( 'NONE', #789, #7991 ) ;
#3377=ORIENTED_EDGE ( 'NONE', *, *, #20265, .T. ) ;
#3379=CARTESIAN_POINT ( 'NONE',  ( 0.000000000000000000, -56.78056608349999834, 0.000000000000000000 ) ) ;
#3380=CARTESIAN_POINT ( 'NONE',  ( 47.25000000000000000, -74.00000000000000000, 8.881784196999999612E-15 ) ) ;
#3382=CARTESIAN_POINT ( 'NONE',  ( 30.75969929770000277, -73.34323049660000038, -23.57645225990000171 ) ) ;
#3383=EDGE_CURVE ( 'NONE', #5488, #8306, #10177, .T. ) ;
#3384=CARTESIAN_POINT ( 'NONE',  ( -14.46557528003321025, -70.49261988755607433, 23.52773505033430723 ) ) ;
#3389=CARTESIAN_POINT ( 'NONE',  ( 21.19011208810000113, -36.03998686679999963, -8.396978594420000164 ) ) ;
#3390=CARTESIAN_POINT ( 'NONE',  ( 20.49735013020000096, -36.03245755269999506, -9.139729082780000624 ) ) ;
#3394=B_SPLINE_SURFACE_WITH_KNOTS ( 'NONE', 5, 5, ( 
 ( #23536, #16403, #12163, #21076, #5888, #28046 ),
 ( #16974, #12016, #14767, #23668, #11879, #20793 ),
 ( #845, #9690, #9974, #27642, #16682, #16549 ),
 ( #18605, #12303, #25445, #27771, #27493, #25311 ),
 ( #7808, #5339, #994, #21213, #9837, #18747 ),
 ( #8215, #28604, #17541, #17399, #3713, #19717 ) ),
 .UNSPECIFIED., .F., .F., .F.,
 ( 6, 6 ),
 ( 6, 6 ),
 ( 1.309430326270000000, 3.318582255669999981 ),
 ( 0.000000000000000000, 0.5000000000000000000 ),
 .UNSPECIFIED. ) ;
#3395=FACE_OUTER_BOUND ( 'NONE', #1279, .T. ) ;
#3396=DIRECTION ( 'NONE',  ( 0.000000000000000000, -1.000000000000000000, 0.000000000000000000 ) ) ;
#3397=CARTESIAN_POINT ( 'NONE',  ( 8.465915579399998947, -40.73328259390000028, -21.79505839740000184 ) ) ;
#3399=EDGE_LOOP ( 'NONE', ( #11630, #2471, #11380, #9755 ) ) ;
#3401=DIRECTION ( 'NONE',  ( 0.9952295494196657932, 0.000000000000000000, -0.09756097560976527416 ) ) ;
#3403=ORIENTED_EDGE ( 'NONE', *, *, #11049, .T. ) ;
#3404=AXIS2_PLACEMENT_3D ( 'NONE', #16967, #27485, #21337 ) ;
#3405=CARTESIAN_POINT ( 'NONE',  ( 20.10370293170000267, -18.85979313690000225, -8.426925535960000602 ) ) ;
#3409=CARTESIAN_POINT ( 'NONE',  ( -14.66608903329999869, -74.50000000000000000, 36.47374631129999756 ) ) ;
#3410=DIRECTION ( 'NONE',  ( 0.000000000000000000, -1.000000000000000000, 0.000000000000000000 ) ) ;
#3412=EDGE_CURVE ( 'NONE', #2130, #13695, #27423, .T. ) ;
#3415=DIRECTION ( 'NONE',  ( 0.000000000000000000, 1.000000000000000000, 0.000000000000000000 ) ) ;
#3416=CARTESIAN_POINT ( 'NONE',  ( -32.83566817730000054, -74.50000000000000000, -22.22906645950000026 ) ) ;
#3417=FACE_OUTER_BOUND ( 'NONE', #17356, .T. ) ;
#3418=ORIENTED_EDGE ( 'NONE', *, *, #26655, .T. ) ;
#3419=CARTESIAN_POINT ( 'NONE',  ( -32.77174709959999888, -74.43710720380001078, -21.60034937849999892 ) ) ;
#3420=CARTESIAN_POINT ( 'NONE',  ( -21.60034937969999902, -74.50000000000000000, -32.77174707999999725 ) ) ;
#3421=AXIS2_PLACEMENT_3D ( 'NONE', #20098, #24470, #12932 ) ;
#3422=CARTESIAN_POINT ( 'NONE',  ( 7.564829567879999012E-15, -73.00000000000000000, 32.75000000000000000 ) ) ;
#3423=CARTESIAN_POINT ( 'NONE',  ( 19.90557433739999738, -34.65022632540000558, -8.965966767359999423 ) ) ;
#3424=CARTESIAN_POINT ( 'NONE',  ( 7.250038883935697065, -73.95086734785802207, 39.95935625373193290 ) ) ;
#3425=CARTESIAN_POINT ( 'NONE',  ( -13.96596450430000047, -64.58097845250000546, 21.73803617189999926 ) ) ;
#3427=CARTESIAN_POINT ( 'NONE',  ( -38.79568063749716345, -74.00014642295835188, 7.600472224630967055 ) ) ;
#3428=EDGE_CURVE ( 'NONE', #5725, #6342, #7682, .T. ) ;
#3431=CARTESIAN_POINT ( 'NONE',  ( 31.68381302702793434, -74.06963932891925140, -22.77788534991574210 ) ) ;
#3437=PLANE ( 'NONE',  #1876 ) ;
#3438=AXIS2_PLACEMENT_3D ( 'NONE', #5161, #668, #24973 ) ;
#3440=CARTESIAN_POINT ( 'NONE',  ( 20.33277134760000138, -73.81489374239998824, -32.04417015119999945 ) ) ;
#3441=ADVANCED_FACE ( 'NONE', ( #15767 ), #24673, .T. ) ;
#3443=DIRECTION ( 'NONE',  ( 0.000000000000000000, 1.000000000000000000, 0.000000000000000000 ) ) ;
#3444=DIRECTION ( 'NONE',  ( 0.000000000000000000, -1.000000000000000000, 0.000000000000000000 ) ) ;
#3445=DIRECTION ( 'NONE',  ( 1.000000000000000000, 0.000000000000000000, 0.000000000000000000 ) ) ;
#3447=CARTESIAN_POINT ( 'NONE',  ( -31.64302845809999809, -74.00000000000000000, -31.64302845809999809 ) ) ;
#3449=ORIENTED_EDGE ( 'NONE', *, *, #18469, .T. ) ;
#3451=CARTESIAN_POINT ( 'NONE',  ( -14.01337423622812928, -80.36910030610464162, 36.66316738247557083 ) ) ;
#3453=CARTESIAN_POINT ( 'NONE',  ( 9.828880478180000324, -36.53914149509999731, -22.51363315740000104 ) ) ;
#3454=DIRECTION ( 'NONE',  ( 0.000000000000000000, 1.000000000000000000, 0.000000000000000000 ) ) ;
#3455=FACE_OUTER_BOUND ( 'NONE', #3067, .T. ) ;
#3457=CARTESIAN_POINT ( 'NONE',  ( 19.83285472758843682, -19.48229551556754657, -8.720275436146035730 ) ) ;
#3461=CIRCLE ( 'NONE', #28561, 7.250000000000000000 ) ;
#3462=CARTESIAN_POINT ( 'NONE',  ( 23.03829042120000281, -52.56313962710000709, 10.32398954119999956 ) ) ;
#3463=CARTESIAN_POINT ( 'NONE',  ( 9.032270281389999766, -35.86447823839999671, -20.16936839779999957 ) ) ;
#3464=FACE_OUTER_BOUND ( 'NONE', #19566, .T. ) ;
#3467=CARTESIAN_POINT ( 'NONE',  ( -17.65314336990000399, -18.50000000000000000, 13.58065803889999934 ) ) ;
#3471=CARTESIAN_POINT ( 'NONE',  ( -32.77954208402166358, -74.32766453548276786, -22.21551416184748717 ) ) ;
#3472=B_SPLINE_CURVE_WITH_KNOTS ( 'NONE', 5,
 ( #4311, #110, #6346, #28772, #10837, #19746, #4602, #15210, #24125, #8959, #4160, #13033, #13186, #17867, #22095, #10974, #18606, #20935 ),
 .UNSPECIFIED., .F., .F.,
 ( 6, 3, 3, 3, 3, 6 ),
 ( 0.000000000000000000, 1.123597682139999998, 2.251105814059999766, 3.378920982569999953, 4.507089344490000649, 5.576980695549999645 ),
 .UNSPECIFIED. ) ;
#3473=CARTESIAN_POINT ( 'NONE',  ( -19.85441137420000146, -60.55428303689999581, 13.13179032179999872 ) ) ;
#3474=ORIENTED_EDGE ( 'NONE', *, *, #20906, .F. ) ;
#3476=CARTESIAN_POINT ( 'NONE',  ( 46.25000000000000000, -79.00000000000000000, -7.375000000000000000 ) ) ;
#3477=CARTESIAN_POINT ( 'NONE',  ( -3.299060175100000158, -18.50000000000000000, -24.39335979490000028 ) ) ;
#3478=CARTESIAN_POINT ( 'NONE',  ( 36.49396608176380852, -74.06970218573687248, -14.11767483867770601 ) ) ;
#3482=DIRECTION ( 'NONE',  ( 0.000000000000000000, -1.000000000000000000, 0.000000000000000000 ) ) ;
#3483=DIRECTION ( 'NONE',  ( 1.000000000000000000, 0.000000000000000000, 0.000000000000000000 ) ) ;
#3487=CARTESIAN_POINT ( 'NONE',  ( 36.77570183985819341, -79.45385781081505172, -14.64121397519159196 ) ) ;
#3489=CARTESIAN_POINT ( 'NONE',  ( -2.450393045606315656, -80.33972342794427846, 46.82405269585417074 ) ) ;
#3491=CARTESIAN_POINT ( 'NONE',  ( -14.60877014137605379, -74.50000000000000000, 36.82513846446037320 ) ) ;
#3492=CARTESIAN_POINT ( 'NONE',  ( 47.25000000000000000, -75.00000000000000000, -1.242228542250000064E-12 ) ) ;
#3493=VERTEX_POINT ( 'NONE', #11688 ) ;
#3497=ORIENTED_EDGE ( 'NONE', *, *, #10431, .F. ) ;
#3499=CARTESIAN_POINT ( 'NONE',  ( 22.51853742079654808, -36.00000000000000000, -11.01541626719902922 ) ) ;
#3502=CARTESIAN_POINT ( 'NONE',  ( 39.59129699470000219, -73.90055525949999549, 7.279149876810000031 ) ) ;
#3504=EDGE_CURVE ( 'NONE', #13461, #15756, #28771, .T. ) ;
#3505=LINE ( 'NONE', #3231, #27438 ) ;
#3507=ORIENTED_EDGE ( 'NONE', *, *, #8637, .F. ) ;
#3512=CARTESIAN_POINT ( 'NONE',  ( 40.00000000000000000, -77.00000000000000000, 0.000000000000000000 ) ) ;
#3514=CARTESIAN_POINT ( 'NONE',  ( -2.238370485110000363, -80.04479719919999070, 47.01479521750000146 ) ) ;
#3515=CARTESIAN_POINT ( 'NONE',  ( 24.22382764319999993, -64.24504439390000243, 10.76339940740000145 ) ) ;
#3518=CARTESIAN_POINT ( 'NONE',  ( 4.037078284719999375E-15, -74.00000000000000000, -40.00000000000000000 ) ) ;
#3519=CARTESIAN_POINT ( 'NONE',  ( -14.40572000550000098, -18.50000000000000000, 20.06574520719999910 ) ) ;
#3520=CARTESIAN_POINT ( 'NONE',  ( 27.75394116159999669, -74.50000000000000000, -27.75394116159999669 ) ) ;
#3522=DIRECTION ( 'NONE',  ( 1.000000000000000000, 0.000000000000000000, 0.000000000000000000 ) ) ;
#3523=ORIENTED_EDGE ( 'NONE', *, *, #24757, .F. ) ;
#3524=CARTESIAN_POINT ( 'NONE',  ( 9.332951828819998852, -36.18018306619999436, -21.06416784469999826 ) ) ;
#3525=CARTESIAN_POINT ( 'NONE',  ( 20.66368818489999981, -35.66750349659999841, -8.753531078070000859 ) ) ;
#3527=CARTESIAN_POINT ( 'NONE',  ( 20.03541958720000338, -35.94892542979999916, -9.230207021330000927 ) ) ;
#3538=ORIENTED_EDGE ( 'NONE', *, *, #5536, .F. ) ;
#3539=ADVANCED_FACE ( 'NONE', ( #24789 ), #480, .F. ) ;
#3541=DIRECTION ( 'NONE',  ( -2.220446049250000002E-16, 0.000000000000000000, 1.000000000000000000 ) ) ;
#3544=CARTESIAN_POINT ( 'NONE',  ( -14.60455326470000159, -74.31496036839999419, 36.89972645289999775 ) ) ;
#3546=CARTESIAN_POINT ( 'NONE',  ( -14.51929513910000047, -74.27627443250000283, 36.71621193889999546 ) ) ;
#3549=ORIENTED_EDGE ( 'NONE', *, *, #13069, .T. ) ;
#3551=DIRECTION ( 'NONE',  ( -0.09756097560976655092, 0.000000000000000000, -0.9952295494196655712 ) ) ;
#3552=CARTESIAN_POINT ( 'NONE',  ( 23.52622212079999997, -57.40875702419999982, -9.564509902250000195 ) ) ;
#3553=DIRECTION ( 'NONE',  ( 0.000000000000000000, 1.000000000000000000, 0.000000000000000000 ) ) ;
#3554=CARTESIAN_POINT ( 'NONE',  ( 22.62017292919999889, -58.65571127909999660, 10.18887697589999952 ) ) ;
#3560=CARTESIAN_POINT ( 'NONE',  ( 7.299999026299999194, -35.81311514570000298, -21.43074813960000213 ) ) ;
#3561=CARTESIAN_POINT ( 'NONE',  ( 23.73650098047212254, -62.45651223016474773, 10.62604559626449685 ) ) ;
#3566=ORIENTED_EDGE ( 'NONE', *, *, #22511, .F. ) ;
#3567=CARTESIAN_POINT ( 'NONE',  ( 7.508026895748405316, -35.02998825093359869, -21.30133317590891906 ) ) ;
#3572=EDGE_CURVE ( 'NONE', #24310, #11938, #14618, .T. ) ;
#3576=CARTESIAN_POINT ( 'NONE',  ( 25.19069697129999952, -73.33154443940000533, -29.87473424289999713 ) ) ;
#3577=CARTESIAN_POINT ( 'NONE',  ( -22.44049059359999987, -70.63300521989999936, 17.23241241100000209 ) ) ;
#3579=CARTESIAN_POINT ( 'NONE',  ( -19.04077152199090150, -19.48549492421237517, 13.94607375679098205 ) ) ;
#3580=CARTESIAN_POINT ( 'NONE',  ( 7.135467526410000261, -73.50000000000000000, 38.71641004229999794 ) ) ;
#3581=EDGE_LOOP ( 'NONE', ( #16468, #10485, #26309, #23412, #24380 ) ) ;
#3583=ORIENTED_EDGE ( 'NONE', *, *, #11371, .F. ) ;
#3585=CARTESIAN_POINT ( 'NONE',  ( -1.158751914399999805, -60.33243244399999128, -23.66032903080000338 ) ) ;
#3587=CARTESIAN_POINT ( 'NONE',  ( 47.25000000000000000, -79.00000000000000000, -7.709388683000000122E-13 ) ) ;
#3589=EDGE_CURVE ( 'NONE', #15352, #22592, #5238, .T. ) ;
#3590=EDGE_LOOP ( 'NONE', ( #7556, #20449, #10072, #24931 ) ) ;
#3594=CARTESIAN_POINT ( 'NONE',  ( 7.619628858569999608, -36.43422328860000192, -21.46039065680000135 ) ) ;
#3596=CARTESIAN_POINT ( 'NONE',  ( 22.12830645909999916, -53.29680639610000270, -7.019998623859999398 ) ) ;
#3597=CARTESIAN_POINT ( 'NONE',  ( -16.95867319479999935, -74.00000000000000000, 44.10460184009999551 ) ) ;
#3600=DIRECTION ( 'NONE',  ( 0.000000000000000000, -1.000000000000000000, 0.000000000000000000 ) ) ;
#3601=CIRCLE ( 'NONE', #27799, 0.5000000000000004441 ) ;
#3604=CARTESIAN_POINT ( 'NONE',  ( -20.08490270809999956, -60.38591348639999268, 14.30072212849999858 ) ) ;
#3606=DIRECTION ( 'NONE',  ( 1.000000000000000000, 0.000000000000000000, 0.000000000000000000 ) ) ;
#3608=AXIS2_PLACEMENT_3D ( 'NONE', #21845, #28673, #19649 ) ;
#3609=CARTESIAN_POINT ( 'NONE',  ( -3.610293792020000225, -18.50000000000000000, -24.43613468120000221 ) ) ;
#3611=VERTEX_POINT ( 'NONE', #23318 ) ;
#3615=AXIS2_PLACEMENT_3D ( 'NONE', #8320, #28433, #6140 ) ;
#3616=CARTESIAN_POINT ( 'NONE',  ( -31.89935321680000158, -74.00000000000000000, -21.99985828019999801 ) ) ;
#3617=CARTESIAN_POINT ( 'NONE',  ( 36.47640386220000153, -80.06330722010001466, -14.49564800679999976 ) ) ;
#3621=CARTESIAN_POINT ( 'NONE',  ( 36.70830968600000688, -79.13352040803519571, -14.75000000000000000 ) ) ;
#3623=DIRECTION ( 'NONE',  ( 1.000000000000000000, 0.000000000000000000, 0.000000000000000000 ) ) ;
#3624=ORIENTED_EDGE ( 'NONE', *, *, #700, .T. ) ;
#3625=AXIS2_PLACEMENT_3D ( 'NONE', #20030, #22084, #2129 ) ;
#3626=CARTESIAN_POINT ( 'NONE',  ( 47.25000000000000000, -75.00000000000000000, -1.242228542250000064E-12 ) ) ;
#3629=CARTESIAN_POINT ( 'NONE',  ( 21.92880676370000259, -37.95796630400000282, -8.677144394200000832 ) ) ;
#3634=AXIS2_PLACEMENT_3D ( 'NONE', #754, #18498, #312 ) ;
#3635=CARTESIAN_POINT ( 'NONE',  ( 9.307965732619999599, -36.00000000019999646, -20.68428864319999860 ) ) ;
#3637=CARTESIAN_POINT ( 'NONE',  ( -3.463923112789999870, -18.50000000000000000, -22.98618337390000121 ) ) ;
#3638=ORIENTED_EDGE ( 'NONE', *, *, #10717, .T. ) ;
#3644=CARTESIAN_POINT ( 'NONE',  ( -3.592524694620000236, -80.18584070859999713, 46.36824188119999945 ) ) ;
#3645=CARTESIAN_POINT ( 'NONE',  ( -12.17277550232225991, -67.87585717449533718, -23.96830675610268102 ) ) ;
#3646=ORIENTED_EDGE ( 'NONE', *, *, #6640, .F. ) ;
#3650=CARTESIAN_POINT ( 'NONE',  ( 30.97095772320000151, -72.00000182920000213, -20.30102774879999927 ) ) ;
#3655=ADVANCED_FACE ( 'NONE', ( #775 ), #1257, .T. ) ;
#3657=B_SPLINE_CURVE_WITH_KNOTS ( 'NONE', 5,
 ( #25517, #7622, #23475, #14162, #12371, #23062 ),
 .UNSPECIFIED., .F., .F.,
 ( 6, 6 ),
 ( 0.000000000000000000, 1.000000000000000000 ),
 .UNSPECIFIED. ) ;
#3658=FACE_OUTER_BOUND ( 'NONE', #2496, .T. ) ;
#3659=CARTESIAN_POINT ( 'NONE',  ( 20.44148170879999782, -35.89950312469999716, -8.903712398839999764 ) ) ;
#3660=LINE ( 'NONE', #10332, #26999 ) ;
#3666=AXIS2_PLACEMENT_3D ( 'NONE', #957, #1227, #16789 ) ;
#3668=CARTESIAN_POINT ( 'NONE',  ( -1.776356839399999804E-15, -80.00000000000000000, 3.552713678799999214E-14 ) ) ;
#3675=FACE_OUTER_BOUND ( 'NONE', #4516, .T. ) ;
#3676=CARTESIAN_POINT ( 'NONE',  ( -14.39310877959999857, -74.06193868690000670, 36.25276817999999679 ) ) ;
#3678=FACE_OUTER_BOUND ( 'NONE', #18113, .T. ) ;
#3681=AXIS2_PLACEMENT_3D ( 'NONE', #12739, #5638, #1702 ) ;
#3683=CARTESIAN_POINT ( 'NONE',  ( 7.752235230210000161, -60.58770331659999897, -22.38439241200000396 ) ) ;
#3688=VECTOR ( 'NONE', #27782, 1000.000000000000000 ) ;
#3690=AXIS2_PLACEMENT_3D ( 'NONE', #24349, #4675, #24203 ) ;
#3694=AXIS2_PLACEMENT_3D ( 'NONE', #15595, #24494, #6870 ) ;
#3697=LINE ( 'NONE', #6152, #1184 ) ;
#3699=CARTESIAN_POINT ( 'NONE',  ( -8.022711211519999219E-16, -84.50000000000000000, 40.00000000000000000 ) ) ;
#3702=CARTESIAN_POINT ( 'NONE',  ( 20.36793921130000129, -34.63244748730000566, -8.805019764629998136 ) ) ;
#3705=ORIENTED_EDGE ( 'NONE', *, *, #865, .F. ) ;
#3708=EDGE_LOOP ( 'NONE', ( #20867, #9417, #11317, #1461 ) ) ;
#3709=ORIENTED_EDGE ( 'NONE', *, *, #9383, .F. ) ;
#3710=CIRCLE ( 'NONE', #8800, 2.000000000000000000 ) ;
#3711=AXIS2_PLACEMENT_3D ( 'NONE', #20008, #20159, #20303 ) ;
#3713=CARTESIAN_POINT ( 'NONE',  ( -7.472969336320000266, -74.00000023179998720, 38.65569830309999588 ) ) ;
#3715=CARTESIAN_POINT ( 'NONE',  ( 23.57312445299999837, -73.96004965659999186, -31.14713777060000055 ) ) ;
#3717=B_SPLINE_CURVE_WITH_KNOTS ( 'NONE', 5,
 ( #12270, #11985, #7913, #9941, #16798, #18855 ),
 .UNSPECIFIED., .F., .F.,
 ( 6, 6 ),
 ( -66.18347591719999912, -38.72099907209999969 ),
 .UNSPECIFIED. ) ;
#3718=LINE ( 'NONE', #19306, #12948 ) ;
#3719=CARTESIAN_POINT ( 'NONE',  ( -12.00784032640000021, -65.53745956570000430, -24.10472249089999863 ) ) ;
#3720=CARTESIAN_POINT ( 'NONE',  ( 7.023816214479999154, -35.71220903070000219, -21.48235969790000155 ) ) ;
#3722=ORIENTED_EDGE ( 'NONE', *, *, #9583, .T. ) ;
#3724=ORIENTED_EDGE ( 'NONE', *, *, #27470, .F. ) ;
#3725=CIRCLE ( 'NONE', #8819, 0.5000000000000027756 ) ;
#3726=CIRCLE ( 'NONE', #10656, 2.000000035460000269 ) ;
#3727=EDGE_CURVE ( 'NONE', #24375, #11422, #26058, .T. ) ;
#3728=CIRCLE ( 'NONE', #26518, 25.14975229270000057 ) ;
#3729=VERTEX_POINT ( 'NONE', #17462 ) ;
#3730=CARTESIAN_POINT ( 'NONE',  ( -2.567392390289999771, -60.04642514249999863, -25.10623713540000068 ) ) ;
#3739=CARTESIAN_POINT ( 'NONE',  ( -14.03539743980000054, -80.18584161550000999, 36.72078694980000080 ) ) ;
#3740=CIRCLE ( 'NONE', #20020, 2.000000000000001776 ) ;
#3741=CARTESIAN_POINT ( 'NONE',  ( -18.79730758629999698, -18.50000000000000000, 15.05721160110000056 ) ) ;
#3744=DIRECTION ( 'NONE',  ( 1.000000000000000000, 0.000000000000000000, 0.000000000000000000 ) ) ;
#3750=CARTESIAN_POINT ( 'NONE',  ( 36.70830968599999977, -79.00000000000000000, -14.75000000000000000 ) ) ;
#3753=EDGE_CURVE ( 'NONE', #26201, #5317, #553, .T. ) ;
#3755=DIRECTION ( 'NONE',  ( -0.7071067811865475727, 0.000000000000000000, -0.7071067811865475727 ) ) ;
#3756=CARTESIAN_POINT ( 'NONE',  ( 37.22080120100000045, -79.99999987929999179, -13.88618458220000029 ) ) ;
#3758=EDGE_CURVE ( 'NONE', #23734, #25273, #21229, .T. ) ;
#3759=DIRECTION ( 'NONE',  ( -0.9295286103719511139, 0.000000000000000000, -0.3687499999999862554 ) ) ;
#3760=AXIS2_PLACEMENT_3D ( 'NONE', #3372, #25090, #21150 ) ;
#3762=VECTOR ( 'NONE', #4180, 1000.000000000000000 ) ;
#3763=ORIENTED_EDGE ( 'NONE', *, *, #18503, .F. ) ;
#3765=CARTESIAN_POINT ( 'NONE',  ( 46.66508878058498766, -73.77886964734264552, -2.857274044103978561 ) ) ;
#3766=ORIENTED_EDGE ( 'NONE', *, *, #16561, .T. ) ;
#3767=CARTESIAN_POINT ( 'NONE',  ( 22.19837534649999711, -55.01779585689999408, 10.09345264070000070 ) ) ;
#3769=CARTESIAN_POINT ( 'NONE',  ( -7.440556932039999793, -74.12472287219999600, -39.45553247920000217 ) ) ;
#3770=ORIENTED_EDGE ( 'NONE', *, *, #2617, .T. ) ;
#3772=DIRECTION ( 'NONE',  ( 1.000000000000000000, 0.000000000000000000, 0.000000000000000000 ) ) ;
#3773=ADVANCED_FACE ( 'NONE', ( #23221 ), #10980, .T. ) ;
#3775=CARTESIAN_POINT ( 'NONE',  ( 21.92880676370000259, -37.95796630400000282, -8.677144394200000832 ) ) ;
#3777=CARTESIAN_POINT ( 'NONE',  ( -3.188346920221404535, -79.97866323289575519, 46.91088456186137989 ) ) ;
#3783=EDGE_LOOP ( 'NONE', ( #20641, #8551, #19137, #10968 ) ) ;
#3792=EDGE_CURVE ( 'NONE', #24445, #9130, #13260, .T. ) ;
#3797=CARTESIAN_POINT ( 'NONE',  ( -14.16469261447947403, -74.02381607010246967, 36.23209851156404682 ) ) ;
#3798=ORIENTED_EDGE ( 'NONE', *, *, #25582, .T. ) ;
#3799=CARTESIAN_POINT ( 'NONE',  ( -40.52471375025919542, -74.35734738351742124, -7.233314584366330457 ) ) ;
#3802=CARTESIAN_POINT ( 'NONE',  ( 0.000000000000000000, -18.50000000000000000, 0.000000000000000000 ) ) ;
#3803=ORIENTED_EDGE ( 'NONE', *, *, #20019, .F. ) ;
#3809=CARTESIAN_POINT ( 'NONE',  ( 7.592835430060000057, -49.11291935200000580, -21.85814127600000134 ) ) ;
#3811=EDGE_LOOP ( 'NONE', ( #5199, #10682, #12686, #15097 ) ) ;
#3812=EDGE_CURVE ( 'NONE', #28156, #18665, #11446, .T. ) ;
#3814=CARTESIAN_POINT ( 'NONE',  ( 22.56612536419999770, -34.67035637040000040, -0.2125348757979999836 ) ) ;
#3817=CARTESIAN_POINT ( 'NONE',  ( 19.39105705749999942, -19.17889725919999933, -8.979483757040000569 ) ) ;
#3818=EDGE_CURVE ( 'NONE', #26140, #7412, #16249, .T. ) ;
#3819=CARTESIAN_POINT ( 'NONE',  ( -14.59815767989999991, -74.46648494389999939, 36.63377406709999917 ) ) ;
#3822=VERTEX_POINT ( 'NONE', #27131 ) ;
#3823=DIRECTION ( 'NONE',  ( 0.7071067811865475727, 0.000000000000000000, -0.7071067811865475727 ) ) ;
#3825=CARTESIAN_POINT ( 'NONE',  ( 8.166636963089999313, -62.08211516050000256, -22.74134383390000025 ) ) ;
#3827=CARTESIAN_POINT ( 'NONE',  ( 23.19089252530000422, -58.59418302210000462, 10.40173300340000040 ) ) ;
#3828=CARTESIAN_POINT ( 'NONE',  ( -10.84908614390000103, -27.06313850649999964, -19.75281354290000024 ) ) ;
#3829=CIRCLE ( 'NONE', #27591, 23.36116116979999902 ) ;
#3834=CARTESIAN_POINT ( 'NONE',  ( -32.68025371723170025, -74.50000000070002670, -21.81265875462274195 ) ) ;
#3835=CARTESIAN_POINT ( 'NONE',  ( 21.21591776440000388, -18.50000000000000000, 0.5881982815080000204 ) ) ;
#3836=LINE ( 'NONE', #21616, #12085 ) ;
#3837=VERTEX_POINT ( 'NONE', #783 ) ;
#3846=ORIENTED_EDGE ( 'NONE', *, *, #3030, .F. ) ;
#3848=AXIS2_PLACEMENT_3D ( 'NONE', #11497, #7742, #16608 ) ;
#3850=B_SPLINE_CURVE_WITH_KNOTS ( 'NONE', 5,
 ( #26775, #26469, #24571, #6806, #6504, #4320 ),
 .UNSPECIFIED., .F., .F.,
 ( 6, 6 ),
 ( 0.000000000000000000, 1.000000000000000000 ),
 .UNSPECIFIED. ) ;
#3854=ADVANCED_FACE ( 'NONE', ( #21005 ), #14838, .T. ) ;
#3855=CARTESIAN_POINT ( 'NONE',  ( 19.62372718079999956, -18.50000000000000000, -7.547414732120000913 ) ) ;
#3856=EDGE_CURVE ( 'NONE', #26695, #16270, #19897, .T. ) ;
#3860=CARTESIAN_POINT ( 'NONE',  ( 38.57396449699999863, -80.00000000000000000, -9.597487326430000465 ) ) ;
#3861=CARTESIAN_POINT ( 'NONE',  ( -18.53437987951083343, -19.46453794990133446, 12.04470810626642496 ) ) ;
#3863=VERTEX_POINT ( 'NONE', #11953 ) ;
#3864=CARTESIAN_POINT ( 'NONE',  ( 8.616470839319999797, -18.62200669790000163, -19.27348050239999822 ) ) ;
#3865=VERTEX_POINT ( 'NONE', #14564 ) ;
#3866=DIRECTION ( 'NONE',  ( 0.2414462220490750377, 0.000000000000000000, 0.9704142011833034598 ) ) ;
#3867=AXIS2_PLACEMENT_3D ( 'NONE', #25612, #24378, #6452 ) ;
#3868=CARTESIAN_POINT ( 'NONE',  ( 7.049162187834887128, -36.56981903923507815, -21.51316594787862968 ) ) ;
#3870=DIRECTION ( 'NONE',  ( 0.000000000000000000, -1.000000000000000000, 0.000000000000000000 ) ) ;
#3872=CIRCLE ( 'NONE', #8523, 0.5000000000000027756 ) ;
#3873=CARTESIAN_POINT ( 'NONE',  ( 21.48176983620000158, -36.17740064299999858, -7.146355372150000385 ) ) ;
#3879=AXIS2_PLACEMENT_3D ( 'NONE', #18190, #19921, #24599 ) ;
#3880=CARTESIAN_POINT ( 'NONE',  ( 38.62788938250000115, -74.00000000000000000, 7.627566167509999495 ) ) ;
#3883=CARTESIAN_POINT ( 'NONE',  ( -32.19064304186151304, -74.02457476353460208, -22.07217569486996211 ) ) ;
#3885=EDGE_LOOP ( 'NONE', ( #20754, #16012, #24364, #7146, #24038 ) ) ;
#3893=CARTESIAN_POINT ( 'NONE',  ( 8.611776762660001694, -37.95567967650000440, -21.87916666729999804 ) ) ;
#3894=CARTESIAN_POINT ( 'NONE',  ( -32.08437107960000390, -74.00884812510000188, -21.94309233420000282 ) ) ;
#3895=CARTESIAN_POINT ( 'NONE',  ( 36.73391533630000083, -79.36276986969998859, -14.70890631340000176 ) ) ;
#3896=VERTEX_POINT ( 'NONE', #21836 ) ;
#3898=B_SPLINE_CURVE_WITH_KNOTS ( 'NONE', 3,
 ( #1164, #7838, #16720, #25616, #5646, #2756, #21795, #1574, #7975, #10691, #19609, #10414, #8378, #23698, #1852, #23984, #10134, #8530, #1431, #17433, #5914, #12879, #17285, #12605 ),
 .UNSPECIFIED., .F., .F.,
 ( 4, 2, 2, 1, 1, 1, 2, 2, 2, 1, 1, 1, 2, 2, 4 ),
 ( 0.000000000000000000, 0.2500000000000677236, 0.3750000000000931477, 0.4375000000000944800, 0.4687500000000965339, 0.4843750000000887068, 0.4921875000000847655, 0.5000000000000808242, 0.6249999999998875344, 0.6874999999997915001, 0.7187499999997323252, 0.7343749999997239986, 0.7421874999997207789, 0.7499999999997175593, 1.000000000000000000 ),
 .UNSPECIFIED. ) ;
#3900=CARTESIAN_POINT ( 'NONE',  ( -0.7685659013399879225, -79.79239604273577413, 47.20921231312638611 ) ) ;
#3901=ORIENTED_EDGE ( 'NONE', *, *, #18873, .T. ) ;
#3902=CARTESIAN_POINT ( 'NONE',  ( 47.25008975959999447, -74.83017303949999643, -0.5756401097749999085 ) ) ;
#3905=FACE_OUTER_BOUND ( 'NONE', #16674, .T. ) ;
#3906=CARTESIAN_POINT ( 'NONE',  ( -7.562763921490000207, -74.00035141509999903, -39.03055149349999908 ) ) ;
#3909=CARTESIAN_POINT ( 'NONE',  ( 22.68565687649710227, -36.18510625669999570, -10.42651188819920094 ) ) ;
#3910=EDGE_CURVE ( 'NONE', #23740, #14954, #7369, .T. ) ;
#3912=CIRCLE ( 'NONE', #28129, 0.5000000000000012212 ) ;
#3913=CARTESIAN_POINT ( 'NONE',  ( -36.23922253580000330, -74.50000000000000000, -26.33972759919999973 ) ) ;
#3915=LINE ( 'NONE', #19088, #26957 ) ;
#3916=VERTEX_POINT ( 'NONE', #1890 ) ;
#3919=CARTESIAN_POINT ( 'NONE',  ( 7.418111264149999342E-16, -69.50000000000000000, -33.25000000000000000 ) ) ;
#3922=AXIS2_PLACEMENT_3D ( 'NONE', #27351, #5349, #20802 ) ;
#3926=CARTESIAN_POINT ( 'NONE',  ( 21.79230230059999940, -37.95144147500000287, -8.472395268590000583 ) ) ;
#3929=CARTESIAN_POINT ( 'NONE',  ( 22.96745989159999723, -18.50000000000000000, 9.091461454319999191 ) ) ;
#3931=DIRECTION ( 'NONE',  ( 0.000000000000000000, 1.000000000000000000, 0.000000000000000000 ) ) ;
#3932=EDGE_CURVE ( 'NONE', #8854, #9278, #13385, .T. ) ;
#3934=AXIS2_PLACEMENT_3D ( 'NONE', #18719, #7656, #20306 ) ;
#3936=CARTESIAN_POINT ( 'NONE',  ( 19.53732555980000285, -35.60472305269999538, -8.991793591719998702 ) ) ;
#3938=CARTESIAN_POINT ( 'NONE',  ( 19.93895660729999975, -35.91131188369999450, -9.181219786679999828 ) ) ;
#3939=DIRECTION ( 'NONE',  ( 0.09756097560976770278, 0.000000000000000000, 0.9952295494196654602 ) ) ;
#3945=AXIS2_PLACEMENT_3D ( 'NONE', #16672, #10093, #19012 ) ;
#3947=CARTESIAN_POINT ( 'NONE',  ( 19.90557383419769266, -34.65022531193147159, -8.965967189900016621 ) ) ;
#3948=FACE_OUTER_BOUND ( 'NONE', #26376, .T. ) ;
#3950=ORIENTED_EDGE ( 'NONE', *, *, #14642, .T. ) ;
#3952=CARTESIAN_POINT ( 'NONE',  ( 22.95539802729999579, -27.05112424559999695, 1.027418781419999982 ) ) ;
#3953=CARTESIAN_POINT ( 'NONE',  ( 25.28698659450000363, -67.37930764479999368, 10.90088209369999994 ) ) ;
#3955=ORIENTED_EDGE ( 'NONE', *, *, #9552, .F. ) ;
#3959=CARTESIAN_POINT ( 'NONE',  ( -38.71641004229999794, -73.50000000000000000, 7.135467526410000261 ) ) ;
#3963=CARTESIAN_POINT ( 'NONE',  ( 28.27563371580000151, -71.49912264920001803, 2.269389644629999925 ) ) ;
#3965=CARTESIAN_POINT ( 'NONE',  ( 9.020398574519999713, -35.69157542760000013, -19.55164510480000217 ) ) ;
#3966=CARTESIAN_POINT ( 'NONE',  ( 9.629159357529998076, -60.22022526889999483, -23.71524624790000146 ) ) ;
#3967=CARTESIAN_POINT ( 'NONE',  ( -12.07720592679999960, -68.19952391640001110, -25.04943555990000448 ) ) ;
#3968=CARTESIAN_POINT ( 'NONE',  ( 22.89499695709999827, -58.22369335140000146, 10.25598920059999841 ) ) ;
#3969=FACE_OUTER_BOUND ( 'NONE', #27510, .T. ) ;
#3970=ORIENTED_EDGE ( 'NONE', *, *, #23115, .T. ) ;
#3971=EDGE_CURVE ( 'NONE', #9596, #6780, #3192, .T. ) ;
#3975=CARTESIAN_POINT ( 'NONE',  ( -40.00000000000000000, -84.00000000000000000, -8.881784197000000993E-16 ) ) ;
#3976=DIRECTION ( 'NONE',  ( 0.000000000000000000, 1.000000000000000000, 0.000000000000000000 ) ) ;
#3977=EDGE_CURVE ( 'NONE', #21398, #24310, #21890, .T. ) ;
#3978=DIRECTION ( 'NONE',  ( 0.7506477800816132584, 0.000000000000000000, -0.6607025883546591150 ) ) ;
#3983=ORIENTED_EDGE ( 'NONE', *, *, #25055, .T. ) ;
#3984=CARTESIAN_POINT ( 'NONE',  ( -14.65665286289999969, -79.25000000000000000, 36.94583910070000599 ) ) ;
#3985=DIRECTION ( 'NONE',  ( -0.7071067811865470176, 0.000000000000000000, 0.7071067811865480168 ) ) ;
#3986=ORIENTED_EDGE ( 'NONE', *, *, #14508, .F. ) ;
#3988=EDGE_LOOP ( 'NONE', ( #1397, #1967, #22313, #27858 ) ) ;
#3990=CARTESIAN_POINT ( 'NONE',  ( 21.65058109989999835, -18.61782386119999799, -0.1214948449970000149 ) ) ;
#3991=DIRECTION ( 'NONE',  ( 1.000000000000000000, 0.000000000000000000, 0.000000000000000000 ) ) ;
#3996=CARTESIAN_POINT ( 'NONE',  ( -18.71988641671584119, -19.47731532785768849, 13.50356754889457100 ) ) ;
#3997=CARTESIAN_POINT ( 'NONE',  ( 7.100559683520000220, -35.25283571269999783, -21.44183144160000154 ) ) ;
#3998=AXIS2_PLACEMENT_3D ( 'NONE', #5896, #21352, #4139 ) ;
#4001=CARTESIAN_POINT ( 'NONE',  ( 36.74383114260000127, -74.66666666670001007, -14.69280904159999857 ) ) ;
#4005=CARTESIAN_POINT ( 'NONE',  ( -1.348885035479999939, -65.00127796780000722, -25.13407207219999862 ) ) ;
#4006=B_SPLINE_CURVE_WITH_KNOTS ( 'NONE', 5,
 ( #14237, #14085, #25319, #9699, #18613, #20942, #7554, #10111, #19031 ),
 .UNSPECIFIED., .F., .F.,
 ( 6, 3, 6 ),
 ( 0.000000000000000000, 0.5000000000000000000, 1.000000000000000000 ),
 .UNSPECIFIED. ) ;
#4007=EDGE_CURVE ( 'NONE', #17905, #20759, #10567, .T. ) ;
#4009=CARTESIAN_POINT ( 'NONE',  ( -19.56318090859999970, -55.04870336940000186, 12.97254176369999890 ) ) ;
#4011=DIRECTION ( 'NONE',  ( 0.000000000000000000, 1.000000000000000000, 0.000000000000000000 ) ) ;
#4015=EDGE_LOOP ( 'NONE', ( #18351, #27042 ) ) ;
#4017=CARTESIAN_POINT ( 'NONE',  ( -14.30456952449999797, -80.50000235099999202, 36.55186667960000335 ) ) ;
#4018=CARTESIAN_POINT ( 'NONE',  ( -17.81645507309999843, -18.50000000000000000, 13.97041869859999963 ) ) ;
#4019=CARTESIAN_POINT ( 'NONE',  ( 21.88295226250000169, -19.17792668139999890, 9.573516633400002362 ) ) ;
#4020=CARTESIAN_POINT ( 'NONE',  ( -32.46498206463285641, -74.10093221338760827, -22.13944811776638133 ) ) ;
#4026=DIRECTION ( 'NONE',  ( 0.000000000000000000, 0.000000000000000000, -1.000000000000000000 ) ) ;
#4028=ORIENTED_EDGE ( 'NONE', *, *, #15849, .T. ) ;
#4032=EDGE_CURVE ( 'NONE', #20809, #24813, #4094, .T. ) ;
#4033=CARTESIAN_POINT ( 'NONE',  ( 36.79450594634548111, -79.51015800609961559, -14.61067903185865013 ) ) ;
#4035=DIRECTION ( 'NONE',  ( -0.7071067811865457964, 0.000000000000000000, -0.7071067811865492381 ) ) ;
#4036=EDGE_CURVE ( 'NONE', #6381, #26221, #13076, .T. ) ;
#4038=CARTESIAN_POINT ( 'NONE',  ( -19.90809684629999765, -55.86335041469999396, 12.11525402310000032 ) ) ;
#4041=CARTESIAN_POINT ( 'NONE',  ( 20.56950839670000164, -55.05548131559999803, 10.89901456070000130 ) ) ;
#4042=DIRECTION ( 'NONE',  ( 0.9952295494196653491, 0.000000000000000000, -0.09756097560976997873 ) ) ;
#4047=DIRECTION ( 'NONE',  ( 0.5301416321220552286, 0.000000000000000000, 0.8479091047340884257 ) ) ;
#4048=CARTESIAN_POINT ( 'NONE',  ( -11.48284226354935988, -58.59018045370876138, -22.64916359960036729 ) ) ;
#4049=CARTESIAN_POINT ( 'NONE',  ( -2.792231499789999738, -18.50000000000000000, -21.92192335580000062 ) ) ;
#4050=EDGE_LOOP ( 'NONE', ( #11231, #3153, #12446, #23594 ) ) ;
#4051=CARTESIAN_POINT ( 'NONE',  ( 25.14694229440000228, -65.07443093669999712, -0.3759436444569999591 ) ) ;
#4053=DIRECTION ( 'NONE',  ( 0.000000000000000000, -1.000000000000000000, 0.000000000000000000 ) ) ;
#4054=ORIENTED_EDGE ( 'NONE', *, *, #25632, .F. ) ;
#4057=CARTESIAN_POINT ( 'NONE',  ( -19.59431184860000030, -18.62337006899999992, 14.76282615579999913 ) ) ;
#4058=ORIENTED_EDGE ( 'NONE', *, *, #4331, .F. ) ;
#4060=B_SPLINE_CURVE_WITH_KNOTS ( 'NONE', 5,
 ( #9305, #5523, #25630, #1046, #16737, #7442 ),
 .UNSPECIFIED., .F., .F.,
 ( 6, 6 ),
 ( -7.329014384030000606, -6.713731535029999975 ),
 .UNSPECIFIED. ) ;
#4061=LINE ( 'NONE', #17773, #28738 ) ;
#4062=FACE_OUTER_BOUND ( 'NONE', #10262, .T. ) ;
#4063=CARTESIAN_POINT ( 'NONE',  ( 7.879643458700000380, -36.30219044630000269, -21.38844997820000060 ) ) ;
#4067=CARTESIAN_POINT ( 'NONE',  ( -11.91266501540000000, -79.50000000000000000, 46.64429291560000479 ) ) ;
#4069=EDGE_CURVE ( 'NONE', #4763, #22615, #13226, .T. ) ;
#4072=CARTESIAN_POINT ( 'NONE',  ( 24.41687773985064780, -18.97801304285953350, 1.565715090140727517 ) ) ;
#4073=ORIENTED_EDGE ( 'NONE', *, *, #13996, .F. ) ;
#4075=CARTESIAN_POINT ( 'NONE',  ( 20.95125717089999995, -36.09768395309999534, -8.611231333170000113 ) ) ;
#4077=ORIENTED_EDGE ( 'NONE', *, *, #22960, .F. ) ;
#4080=CARTESIAN_POINT ( 'NONE',  ( -3.356616257537091474, -68.05312507927790477, -27.55666181306940032 ) ) ;
#4081=CARTESIAN_POINT ( 'NONE',  ( -0.5590517731190000061, -18.50000000000000000, -21.02688049580000040 ) ) ;
#4084=DIRECTION ( 'NONE',  ( -0.9952295494196657932, 0.000000000000000000, 0.09756097560976527416 ) ) ;
#4085=CARTESIAN_POINT ( 'NONE',  ( -10.44618222529999940, -18.50000000000000000, -18.70089465730000100 ) ) ;
#4087=ORIENTED_EDGE ( 'NONE', *, *, #24723, .F. ) ;
#4088=AXIS2_PLACEMENT_3D ( 'NONE', #2177, #4497, #11015 ) ;
#4089=DIRECTION ( 'NONE',  ( 1.000000000000000000, 0.000000000000000000, 0.000000000000000000 ) ) ;
#4090=CARTESIAN_POINT ( 'NONE',  ( 22.02876637549999828, -19.46348310600000175, -0.4636467615609999871 ) ) ;
#4091=CARTESIAN_POINT ( 'NONE',  ( 23.20278881559999817, -65.91612967349999508, 11.11676163019999919 ) ) ;
#4093=VERTEX_POINT ( 'NONE', #2321 ) ;
#4094=CIRCLE ( 'NONE', #18065, 28.68388914670000034 ) ;
#4095=CARTESIAN_POINT ( 'NONE',  ( 4.882943008269999509E-15, -73.00000000000000000, -40.00000000000000000 ) ) ;
#4099=CARTESIAN_POINT ( 'NONE',  ( 36.82697894980000086, -80.49999984420000487, -13.57704391360000074 ) ) ;
#4102=CARTESIAN_POINT ( 'NONE',  ( 7.268665519299999822, -62.14086513569999681, -22.85591912949999838 ) ) ;
#4104=CARTESIAN_POINT ( 'NONE',  ( 22.86993016659999967, -57.41946943429999806, 10.24154007049999926 ) ) ;
#4105=CARTESIAN_POINT ( 'NONE',  ( 24.16120406939999654, -64.60178126830000167, -9.605465959289999134 ) ) ;
#4111=CIRCLE ( 'NONE', #24122, 21.03431122519999974 ) ;
#4112=ORIENTED_EDGE ( 'NONE', *, *, #19158, .F. ) ;
#4113=CARTESIAN_POINT ( 'NONE',  ( 21.02495559440000150, -29.55373279730000391, -7.687066009020000479 ) ) ;
#4114=CARTESIAN_POINT ( 'NONE',  ( 23.90010427143523941, -63.16487826049581145, 10.68054471888447843 ) ) ;
#4115=CARTESIAN_POINT ( 'NONE',  ( 25.26718046270000073, -74.00000000000000000, 6.129403842640000377 ) ) ;
#4119=ORIENTED_EDGE ( 'NONE', *, *, #13410, .F. ) ;
#4123=CARTESIAN_POINT ( 'NONE',  ( 9.028475982079999795, -35.72979163269999958, -19.84586683699999909 ) ) ;
#4124=FACE_OUTER_BOUND ( 'NONE', #7426, .T. ) ;
#4126=ADVANCED_FACE ( 'NONE', ( #9003 ), #12840, .T. ) ;
#4127=CARTESIAN_POINT ( 'NONE',  ( 22.01810471299999961, -19.15810975349999978, -0.4634309158250000116 ) ) ;
#4130=CARTESIAN_POINT ( 'NONE',  ( 23.56559805210000036, -58.81638232979999970, -9.577937461890000392 ) ) ;
#4131=ORIENTED_EDGE ( 'NONE', *, *, #10950, .T. ) ;
#4134=AXIS2_PLACEMENT_3D ( 'NONE', #8089, #14907, #5894 ) ;
#4135=DIRECTION ( 'NONE',  ( 0.000000000000000000, 1.000000000000000000, 0.000000000000000000 ) ) ;
#4138=CARTESIAN_POINT ( 'NONE',  ( -18.48666763681400838, -19.46756325244718155, 12.61459962061059059 ) ) ;
#4139=DIRECTION ( 'NONE',  ( 1.000000000000000000, 0.000000000000000000, 0.000000000000000000 ) ) ;
#4142=ORIENTED_EDGE ( 'NONE', *, *, #3932, .T. ) ;
#4143=CARTESIAN_POINT ( 'NONE',  ( 7.593154301330000244, -18.50000000000000000, -19.61724635699999908 ) ) ;
#4144=CARTESIAN_POINT ( 'NONE',  ( 22.68565687650000129, -36.18510625669999570, -10.42651188819999852 ) ) ;
#4145=CARTESIAN_POINT ( 'NONE',  ( -0.8491947589009999353, -58.35623000289999851, -23.39045838330000038 ) ) ;
#4146=CIRCLE ( 'NONE', #24159, 34.89999999999999858 ) ;
#4147=CARTESIAN_POINT ( 'NONE',  ( 10.65875326940000001, -36.00000000000000000, -21.02691194339999825 ) ) ;
#4150=FACE_OUTER_BOUND ( 'NONE', #7759, .T. ) ;
#4151=CIRCLE ( 'NONE', #12978, 6.750000000000000000 ) ;
#4152=AXIS2_PLACEMENT_3D ( 'NONE', #21003, #5267, #9765 ) ;
#4154=CARTESIAN_POINT ( 'NONE',  ( 21.41502072009999935, -35.30712908469999434, -7.187003606720000271 ) ) ;
#4158=CARTESIAN_POINT ( 'NONE',  ( -14.28268380569999962, -79.99937754569999981, 36.92904800159999468 ) ) ;
#4159=EDGE_CURVE ( 'NONE', #11754, #26673, #7275, .T. ) ;
#4160=CARTESIAN_POINT ( 'NONE',  ( -9.435680430750000625, -18.50000000000000000, -20.63248585200000207 ) ) ;
#4163=CARTESIAN_POINT ( 'NONE',  ( -26.69328098980000163, -74.00000000000000000, -35.88566914520000495 ) ) ;
#4164=CARTESIAN_POINT ( 'NONE',  ( 10.08507888390000140, -64.24505061060000344, -24.78972398320000181 ) ) ;
#4167=CYLINDRICAL_SURFACE ( 'NONE', #7406, 3.749999999999996447 ) ;
#4169=EDGE_CURVE ( 'NONE', #26586, #28649, #17404, .T. ) ;
#4172=ORIENTED_EDGE ( 'NONE', *, *, #24675, .F. ) ;
#4174=AXIS2_PLACEMENT_3D ( 'NONE', #4222, #8719, #3939 ) ;
#4175=B_SPLINE_CURVE_WITH_KNOTS ( 'NONE', 5,
 ( #5384, #12581, #23819, #8358, #6328, #23022, #3073, #11927, #892, #18649, #21354, #1411, #7587, #16450, #14267, #15638, #24693, #26584 ),
 .UNSPECIFIED., .F., .F.,
 ( 6, 3, 3, 3, 3, 6 ),
 ( 0.000000000000000000, 1.123597580079999991, 2.251105601749999963, 3.378920662530000563, 4.507088924770000560, 5.576980223840000583 ),
 .UNSPECIFIED. ) ;
#4177=CARTESIAN_POINT ( 'NONE',  ( -32.08921965649999919, -74.00994675159999758, -21.99574735890000099 ) ) ;
#4178=ORIENTED_EDGE ( 'NONE', *, *, #12355, .T. ) ;
#4180=DIRECTION ( 'NONE',  ( -1.000000000000000000, 0.000000000000000000, 0.000000000000000000 ) ) ;
#4181=CARTESIAN_POINT ( 'NONE',  ( 24.92937355771860197, -41.21911678059012729, 1.391361396670305339 ) ) ;
#4182=CARTESIAN_POINT ( 'NONE',  ( -22.43272077086249183, -80.34292036766261447, -32.20769378288610341 ) ) ;
#4185=ORIENTED_EDGE ( 'NONE', *, *, #3910, .T. ) ;
#4187=DIRECTION ( 'NONE',  ( 0.000000000000000000, 1.000000000000000000, 0.000000000000000000 ) ) ;
#4190=CARTESIAN_POINT ( 'NONE',  ( 21.64387303326116196, -18.61794787929532546, -0.4555539749991904808 ) ) ;
#4192=CIRCLE ( 'NONE', #4685, 3.000000000000002665 ) ;
#4193=TOROIDAL_SURFACE ( 'NONE', #7504, 38.75000000000000000, 0.5000000000000000000 ) ;
#4194=CARTESIAN_POINT ( 'NONE',  ( 9.377113207090001623, -36.00000000019999646, -20.73064381829999903 ) ) ;
#4196=CARTESIAN_POINT ( 'NONE',  ( -1.156789036890000011, -18.50000000000000000, -21.06078022829999696 ) ) ;
#4197=EDGE_LOOP ( 'NONE', ( #7874, #15535, #5355, #12327 ) ) ;
#4198=EDGE_CURVE ( 'NONE', #27292, #23692, #10055, .T. ) ;
#4201=CARTESIAN_POINT ( 'NONE',  ( -2.664535259099999805E-15, -72.82938648530000592, -3.552713678799999608E-15 ) ) ;
#4203=DIRECTION ( 'NONE',  ( -1.000000000000000000, 0.000000000000000000, -3.081450948259999971E-16 ) ) ;
#4204=ADVANCED_FACE ( 'NONE', ( #25203 ), #8910, .F. ) ;
#4205=CARTESIAN_POINT ( 'NONE',  ( 10.04439987701514880, -72.76369477738892044, -26.87308552718831933 ) ) ;
#4206=LINE ( 'NONE', #21989, #8901 ) ;
#4209=FACE_OUTER_BOUND ( 'NONE', #6195, .T. ) ;
#4214=AXIS2_PLACEMENT_3D ( 'NONE', #280, #6963, #15973 ) ;
#4216=CARTESIAN_POINT ( 'NONE',  ( -10.13149966729999818, -18.50000000000000000, 18.43352823549999897 ) ) ;
#4217=ORIENTED_EDGE ( 'NONE', *, *, #4407, .T. ) ;
#4220=ORIENTED_EDGE ( 'NONE', *, *, #26245, .F. ) ;
#4221=CARTESIAN_POINT ( 'NONE',  ( 28.63360765790000073, -72.82938648530000592, 1.697648101029999967 ) ) ;
#4222=CARTESIAN_POINT ( 'NONE',  ( -41.00000000000000000, -82.25000000000000000, -10.20110288159999890 ) ) ;
#4223=ORIENTED_EDGE ( 'NONE', *, *, #626, .F. ) ;
#4229=EDGE_CURVE ( 'NONE', #16936, #26524, #5025, .T. ) ;
#4235=EDGE_LOOP ( 'NONE', ( #13213, #23112, #4649, #7 ) ) ;
#4240=CARTESIAN_POINT ( 'NONE',  ( 22.64221431050000177, -34.66889731630000426, 0.1161384314939999940 ) ) ;
#4241=CARTESIAN_POINT ( 'NONE',  ( 24.22381685739999924, -64.24504218810000111, 10.76340169160000038 ) ) ;
#4243=ORIENTED_EDGE ( 'NONE', *, *, #11672, .F. ) ;
#4244=CARTESIAN_POINT ( 'NONE',  ( -2.605870139415221942, -64.47176446041650877, -25.91539817187144834 ) ) ;
#4248=ADVANCED_FACE ( 'NONE', ( #1855 ), #24276, .T. ) ;
#4251=CARTESIAN_POINT ( 'NONE',  ( 7.675802467109999583, -57.47600031380000729, -22.13628273389999990 ) ) ;
#4253=CARTESIAN_POINT ( 'NONE',  ( 21.17771081649999942, -61.87790347820000392, 11.21104585369999995 ) ) ;
#4254=CARTESIAN_POINT ( 'NONE',  ( 22.88682908910000435, -61.98361058570000637, -8.756040560759998925 ) ) ;
#4256=FACE_OUTER_BOUND ( 'NONE', #21115, .T. ) ;
#4263=ORIENTED_EDGE ( 'NONE', *, *, #4749, .F. ) ;
#4265=CARTESIAN_POINT ( 'NONE',  ( 20.70967183530000000, -25.50459736320000204, -8.132923256100001552 ) ) ;
#4268=VERTEX_POINT ( 'NONE', #19189 ) ;
#4269=CARTESIAN_POINT ( 'NONE',  ( 47.16974535660000356, -74.50000000000000000, -1.075756255579999987 ) ) ;
#4273=DIRECTION ( 'NONE',  ( 0.000000000000000000, -1.000000000000000000, 0.000000000000000000 ) ) ;
#4277=CARTESIAN_POINT ( 'NONE',  ( 21.02965312769999784, -18.50000000000000000, -0.4426264348499999723 ) ) ;
#4280=ORIENTED_EDGE ( 'NONE', *, *, #5356, .F. ) ;
#4284=CARTESIAN_POINT ( 'NONE',  ( -13.32502991189999797, -19.49268876740000067, 20.00853956230000108 ) ) ;
#4286=CARTESIAN_POINT ( 'NONE',  ( -43.75000000000000000, -69.00000000000000000, 0.000000000000000000 ) ) ;
#4287=B_SPLINE_CURVE_WITH_KNOTS ( 'NONE', 3,
 ( #11490, #3491, #16602, #16464, #27259, #5528 ),
 .UNSPECIFIED., .F., .F.,
 ( 4, 2, 4 ),
 ( 0.000000000000000000, 0.5000000000000000000, 1.000000000000000000 ),
 .UNSPECIFIED. ) ;
#4288=FACE_OUTER_BOUND ( 'NONE', #28698, .T. ) ;
#4290=DIRECTION ( 'NONE',  ( 0.000000000000000000, -1.000000000000000000, 0.000000000000000000 ) ) ;
#4294=CARTESIAN_POINT ( 'NONE',  ( -10.93437413680000070, -19.50000027030000282, -21.85842452360000010 ) ) ;
#4295=CARTESIAN_POINT ( 'NONE',  ( 22.23224290750000165, -37.35114138160000152, -9.119208908199999186 ) ) ;
#4296=ORIENTED_EDGE ( 'NONE', *, *, #24688, .F. ) ;
#4297=ADVANCED_BREP_SHAPE_REPRESENTATION ( '', ( #15722, #26433 ), #911 ) ;
#4299=CARTESIAN_POINT ( 'NONE',  ( -11.86778496400000016, -60.57945642420000354, 20.49707039420000143 ) ) ;
#4301=VECTOR ( 'NONE', #18518, 1000.000000000000114 ) ;
#4302=CARTESIAN_POINT ( 'NONE',  ( -19.99335094079999919, -53.79621871020000157, 14.42235124120000123 ) ) ;
#4303=CARTESIAN_POINT ( 'NONE',  ( 19.95150103176392520, -19.47987602260658235, -8.638154654088172180 ) ) ;
#4306=DIRECTION ( 'NONE',  ( -0.000000000000000000, 1.000000000000000000, 0.000000000000000000 ) ) ;
#4309=DIRECTION ( 'NONE',  ( 1.000000000000000000, 0.000000000000000000, 0.000000000000000000 ) ) ;
#4311=CARTESIAN_POINT ( 'NONE',  ( -10.89815191770000169, -18.50000000000000000, -17.99090140869999743 ) ) ;
#4313=CARTESIAN_POINT ( 'NONE',  ( -13.82310862910000004, -74.00000000000000000, 36.20061004779999791 ) ) ;
#4314=CARTESIAN_POINT ( 'NONE',  ( 11.00114453930000025, -68.91000853889998723, -26.38226308069999959 ) ) ;
#4316=VERTEX_POINT ( 'NONE', #9561 ) ;
#4318=AXIS2_PLACEMENT_3D ( 'NONE', #11199, #24633, #4668 ) ;
#4320=CARTESIAN_POINT ( 'NONE',  ( -13.44405788329999929, -68.28990366489999531, 22.97003105929999833 ) ) ;
#4323=CARTESIAN_POINT ( 'NONE',  ( -22.62625778519381825, -72.15620726826487896, 17.99661011978010805 ) ) ;
#4326=B_SPLINE_CURVE_WITH_KNOTS ( 'NONE', 5,
 ( #13868, #2812, #22321, #346, #24504, #26848, #794, #4541, #496 ),
 .UNSPECIFIED., .F., .F.,
 ( 6, 3, 6 ),
 ( 0.000000000000000000, 0.5000000000000000000, 1.000000000000000000 ),
 .UNSPECIFIED. ) ;
#4328=CARTESIAN_POINT ( 'NONE',  ( -32.46073318370000038, -74.16345073059999038, -21.90351770710000068 ) ) ;
#4329=CARTESIAN_POINT ( 'NONE',  ( -22.52722182890634528, -79.95932862086812065, -32.70629964928058087 ) ) ;
#4330=VERTEX_POINT ( 'NONE', #27776 ) ;
#4331=EDGE_CURVE ( 'NONE', #25273, #15079, #22952, .T. ) ;
#4332=DIRECTION ( 'NONE',  ( 0.000000000000000000, 1.000000000000000000, 0.000000000000000000 ) ) ;
#4341=CARTESIAN_POINT ( 'NONE',  ( 46.38894337929999523, -73.82071635820000211, -3.552936482959999864 ) ) ;
#4342=EDGE_CURVE ( 'NONE', #6001, #3048, #15615, .T. ) ;
#4343=EDGE_LOOP ( 'NONE', ( #18037, #5993, #19219, #19660, #27783, #18851, #19413 ) ) ;
#4344=AXIS2_PLACEMENT_3D ( 'NONE', #8270, #21408, #17170 ) ;
#4346=CARTESIAN_POINT ( 'NONE',  ( -21.80755408569999787, -80.04548719450001215, -32.63464586140000279 ) ) ;
#4350=ORIENTED_EDGE ( 'NONE', *, *, #27903, .T. ) ;
#4351=CARTESIAN_POINT ( 'NONE',  ( 36.33976381259999755, -73.99988452930000449, -13.99159891000000044 ) ) ;
#4354=CARTESIAN_POINT ( 'NONE',  ( 25.26718046270000073, -18.50000000000000000, 6.129403842640000377 ) ) ;
#4357=CARTESIAN_POINT ( 'NONE',  ( 40.00000000000000000, -69.50000000000000000, 3.566319567039999839E-15 ) ) ;
#4359=CARTESIAN_POINT ( 'NONE',  ( -18.41637023339999857, -19.15979404320000157, 12.71575957319999972 ) ) ;
#4360=ORIENTED_EDGE ( 'NONE', *, *, #6094, .T. ) ;
#4364=CARTESIAN_POINT ( 'NONE',  ( 22.80182977730000005, -18.50000000000000000, 8.962866840220000242 ) ) ;
#4370=ORIENTED_EDGE ( 'NONE', *, *, #8559, .T. ) ;
#4375=CARTESIAN_POINT ( 'NONE',  ( 22.35420107259999867, -19.50000000000000000, 9.881343484100000296 ) ) ;
#4377=EDGE_CURVE ( 'NONE', #17392, #25360, #13515, .T. ) ;
#4380=ADVANCED_FACE ( 'NONE', ( #2675 ), #10053, .T. ) ;
#4386=CARTESIAN_POINT ( 'NONE',  ( -10.21740987579999782, -18.50000000000000000, -18.48932970370000106 ) ) ;
#4387=CARTESIAN_POINT ( 'NONE',  ( 47.20757201636944700, -79.28844410293223177, -0.9918251209386655942 ) ) ;
#4388=ORIENTED_EDGE ( 'NONE', *, *, #27194, .T. ) ;
#4395=CARTESIAN_POINT ( 'NONE',  ( -0.8216735279219999910, -65.07443093669999712, -25.13632616349999793 ) ) ;
#4397=DIRECTION ( 'NONE',  ( 0.9295286103719527793, 0.000000000000000000, 0.3687499999999814260 ) ) ;
#4398=EDGE_LOOP ( 'NONE', ( #16457, #24875, #14601 ) ) ;
#4399=FACE_OUTER_BOUND ( 'NONE', #21298, .T. ) ;
#4402=CARTESIAN_POINT ( 'NONE',  ( 24.27931843075214147, -74.17320152699277003, -30.68465547482643885 ) ) ;
#4404=CARTESIAN_POINT ( 'NONE',  ( 23.19820347179999942, -63.60137401019999714, -8.029207517830000640 ) ) ;
#4405=CARTESIAN_POINT ( 'NONE',  ( 36.22844186549999534, -74.00000000000000000, -13.75000000000000000 ) ) ;
#4407=EDGE_CURVE ( 'NONE', #15327, #12701, #9791, .T. ) ;
#4408=ORIENTED_EDGE ( 'NONE', *, *, #23513, .T. ) ;
#4410=CARTESIAN_POINT ( 'NONE',  ( 24.38417282560000032, -18.50000000000000000, 2.479391470229999950 ) ) ;
#4415=EDGE_CURVE ( 'NONE', #26598, #26756, #7392, .T. ) ;
#4418=AXIS2_PLACEMENT_3D ( 'NONE', #14842, #18959, #27842 ) ;
#4420=DIRECTION ( 'NONE',  ( 0.000000000000000000, 1.000000000000000000, 0.000000000000000000 ) ) ;
#4421=CARTESIAN_POINT ( 'NONE',  ( 9.038647844559999811, -35.72724450169999955, -19.55068585869999964 ) ) ;
#4424=DIRECTION ( 'NONE',  ( -0.2653025664749695811, -0.9430444279528923390, -0.2007031517659765008 ) ) ;
#4427=ORIENTED_EDGE ( 'NONE', *, *, #301, .T. ) ;
#4432=DIRECTION ( 'NONE',  ( 0.000000000000000000, 0.000000000000000000, 1.000000000000000000 ) ) ;
#4433=CARTESIAN_POINT ( 'NONE',  ( -12.24426935569999841, -66.16381828960000178, -22.75094555550000308 ) ) ;
#4435=DIRECTION ( 'NONE',  ( 0.000000000000000000, -1.000000000000000000, 0.000000000000000000 ) ) ;
#4437=ORIENTED_EDGE ( 'NONE', *, *, #5861, .T. ) ;
#4438=CARTESIAN_POINT ( 'NONE',  ( 7.599202688140000106, -18.61794787459999867, -20.27108524870000039 ) ) ;
#4441=EDGE_CURVE ( 'NONE', #8283, #15872, #17711, .T. ) ;
#4442=CARTESIAN_POINT ( 'NONE',  ( -11.50108207929999971, -62.13448031410000283, 21.04282218430000029 ) ) ;
#4445=CARTESIAN_POINT ( 'NONE',  ( -20.22316239190000076, -53.78538132969999452, 14.63937920919999947 ) ) ;
#4447=CARTESIAN_POINT ( 'NONE',  ( -17.42343749999999858, -79.50000000000000000, 43.92022684009999978 ) ) ;
#4451=CARTESIAN_POINT ( 'NONE',  ( 29.25372036608126081, -74.33334105576250295, -26.12545324891368992 ) ) ;
#4452=CARTESIAN_POINT ( 'NONE',  ( 7.314380512960000580, -73.97629583769999329, -39.54203581849999694 ) ) ;
#4455=ORIENTED_EDGE ( 'NONE', *, *, #9170, .T. ) ;
#4457=CARTESIAN_POINT ( 'NONE',  ( 21.00956971319999766, -32.71502530459999747, 9.728137178119999007 ) ) ;
#4461=CARTESIAN_POINT ( 'NONE',  ( 19.36781163719999910, -19.46510053389999939, 10.50580276810000058 ) ) ;
#4462=CARTESIAN_POINT ( 'NONE',  ( 11.10253387620000076, -70.67754404800000145, -26.52623155260000232 ) ) ;
#4464=EDGE_CURVE ( 'NONE', #18925, #14853, #5045, .T. ) ;
#4467=DIRECTION ( 'NONE',  ( 0.2414462220490750377, 0.000000000000000000, 0.9704142011833034598 ) ) ;
#4469=CARTESIAN_POINT ( 'NONE',  ( 21.58901261035154562, -19.48534489990760221, 9.514599319613230577 ) ) ;
#4470=CARTESIAN_POINT ( 'NONE',  ( -40.35968420210000573, -74.26794181949999540, -7.250122995599999065 ) ) ;
#4471=EDGE_LOOP ( 'NONE', ( #8423, #17164, #17093, #24858 ) ) ;
#4473=ORIENTED_EDGE ( 'NONE', *, *, #24881, .F. ) ;
#4475=EDGE_CURVE ( 'NONE', #6357, #4763, #14182, .T. ) ;
#4478=ORIENTED_EDGE ( 'NONE', *, *, #2009, .T. ) ;
#4481=DIRECTION ( 'NONE',  ( 0.000000000000000000, 1.000000000000000000, 0.000000000000000000 ) ) ;
#4486=CARTESIAN_POINT ( 'NONE',  ( 22.25602728219974935, -57.44036991818945381, 10.13208872879983424 ) ) ;
#4488=DIRECTION ( 'NONE',  ( 0.000000000000000000, 1.000000000000000000, 0.000000000000000000 ) ) ;
#4493=CARTESIAN_POINT ( 'NONE',  ( -38.62788659690000515, -74.00000000000000000, 7.627568735119999666 ) ) ;
#4494=CARTESIAN_POINT ( 'NONE',  ( -22.06287047380000033, -74.01117791779999777, -32.15233126369999894 ) ) ;
#4495=ADVANCED_FACE ( 'NONE', ( #3905 ), #18700, .F. ) ;
#4497=DIRECTION ( 'NONE',  ( 0.000000000000000000, -1.000000000000000000, 0.000000000000000000 ) ) ;
#4498=CARTESIAN_POINT ( 'NONE',  ( -7.327696733890933345, -73.99971689350539350, 39.44377223208145011 ) ) ;
#4499=CARTESIAN_POINT ( 'NONE',  ( -18.78219790299999659, -19.46510053389999939, 11.52011550950000007 ) ) ;
#4504=DIRECTION ( 'NONE',  ( 0.9952295494196657932, 0.000000000000000000, 0.09756097560976527416 ) ) ;
#4505=DIRECTION ( 'NONE',  ( -0.09756097560976760563, 0.000000000000000000, -0.9952295494196654602 ) ) ;
#4506=PRODUCT_DEFINITION_CONTEXT ( 'detailed design', #8834, 'design' ) ;
#4507=B_SPLINE_SURFACE_WITH_KNOTS ( 'NONE', 5, 5, ( 
 ( #22956, #14474, #23371, #7659, #5314, #21190, #27749, #5593, #27619 ),
 ( #12135, #18574, #14203, #11857, #7516, #677, #18722, #7787, #23097 ),
 ( #1112, #1241, #7358, #25287, #27469, #27172, #16079, #27318, #9527 ),
 ( #2997, #24979, #5012, #20617, #13900, #20767, #16525, #22804, #16375 ),
 ( #2842, #973, #20908, #18428, #25422, #5454, #14337, #23230, #3280 ),
 ( #11702, #16221, #25136, #5728, #27876, #17079, #17370, #25973, #3552 ) ),
 .UNSPECIFIED., .F., .F., .F.,
 ( 6, 6 ),
 ( 6, 3, 6 ),
 ( 36.59856967279999651, 66.18347591719999912 ),
 ( 0.000000000000000000, 1.000000000000000000, 2.000000000000000000 ),
 .UNSPECIFIED. ) ;
#4509=CYLINDRICAL_SURFACE ( 'NONE', #18633, 0.4999999999999982236 ) ;
#4511=CARTESIAN_POINT ( 'NONE',  ( -41.00000000000000000, -82.25000000000000000, 10.20110288159999890 ) ) ;
#4514=CARTESIAN_POINT ( 'NONE',  ( -11.32359561920000068, -49.87552377809999626, 20.13167398270000064 ) ) ;
#4515=DIRECTION ( 'NONE',  ( 0.5301416321220552286, 0.000000000000000000, 0.8479091047340884257 ) ) ;
#4516=EDGE_LOOP ( 'NONE', ( #16483, #13971, #7468, #3315 ) ) ;
#4521=CARTESIAN_POINT ( 'NONE',  ( 8.681080848429999719, -37.64807918700000045, -21.92361636220000065 ) ) ;
#4523=CARTESIAN_POINT ( 'NONE',  ( -10.46177781019999919, -18.61797548019999837, -19.17903742680000079 ) ) ;
#4524=CARTESIAN_POINT ( 'NONE',  ( 21.49292127480903503, -37.16720133427794082, -7.554708306457890821 ) ) ;
#4525=VERTEX_POINT ( 'NONE', #16505 ) ;
#4526=CARTESIAN_POINT ( 'NONE',  ( -17.94180966909999597, -18.50000000000000000, 18.81731824139999887 ) ) ;
#4528=CARTESIAN_POINT ( 'NONE',  ( -36.25000000000000000, -69.00000000000000000, 2.124561919619999789E-15 ) ) ;
#4530=DIRECTION ( 'NONE',  ( 0.000000000000000000, -1.000000000000000000, 0.000000000000000000 ) ) ;
#4532=CARTESIAN_POINT ( 'NONE',  ( -14.60044964929999978, -79.81260323630000642, 36.96978765280000090 ) ) ;
#4534=CIRCLE ( 'NONE', #12864, 7.250000000000000000 ) ;
#4535=ADVANCED_FACE ( 'NONE', ( #19356 ), #448, .T. ) ;
#4537=CARTESIAN_POINT ( 'NONE',  ( 27.49606721070000148, -67.46050995630001523, 1.934822350479999953 ) ) ;
#4541=CARTESIAN_POINT ( 'NONE',  ( -19.79578083032381031, -57.47815899606673895, 12.40825019997615364 ) ) ;
#4543=ADVANCED_FACE ( 'NONE', ( #22935 ), #804, .T. ) ;
#4544=DIRECTION ( 'NONE',  ( 1.000000000000000000, 0.000000000000000000, 0.000000000000000000 ) ) ;
#4546=B_SPLINE_CURVE_WITH_KNOTS ( 'NONE', 3,
 ( #14225, #13628, #22536, #4894 ),
 .UNSPECIFIED., .F., .F.,
 ( 4, 4 ),
 ( 8.029182300089999980E-15, 6.855861996790000745 ),
 .UNSPECIFIED. ) ;
#4550=VERTEX_POINT ( 'NONE', #20889 ) ;
#4551=CARTESIAN_POINT ( 'NONE',  ( 36.36887067909999871, -79.00000000000000000, -14.85406736540000061 ) ) ;
#4552=DIRECTION ( 'NONE',  ( 0.000000000000000000, 1.000000000000000000, 0.000000000000000000 ) ) ;
#4554=DIRECTION ( 'NONE',  ( 0.000000000000000000, 1.000000000000000000, 0.000000000000000000 ) ) ;
#4555=CARTESIAN_POINT ( 'NONE',  ( 23.47058412056877330, -19.48405044125010832, 1.414240622653882173 ) ) ;
#4556=ORIENTED_EDGE ( 'NONE', *, *, #19091, .T. ) ;
#4557=DIRECTION ( 'NONE',  ( 0.000000000000000000, -1.000000000000000000, 0.000000000000000000 ) ) ;
#4558=CARTESIAN_POINT ( 'NONE',  ( 8.391519205499999856, -36.85003413439999775, -21.45231170510000140 ) ) ;
#4559=CARTESIAN_POINT ( 'NONE',  ( 7.894290250409162546, -19.46654752400787203, -20.57171819332643636 ) ) ;
#4561=DIRECTION ( 'NONE',  ( 0.000000000000000000, 0.000000000000000000, -1.000000000000000000 ) ) ;
#4562=SPHERICAL_SURFACE ( 'NONE', #25663, 2.000000000000000000 ) ;
#4563=CARTESIAN_POINT ( 'NONE',  ( -12.25492964594734779, -19.47261237683157020, 19.18132429780293080 ) ) ;
#4567=ORIENTED_EDGE ( 'NONE', *, *, #6819, .T. ) ;
#4572=DIRECTION ( 'NONE',  ( 0.000000000000000000, 1.000000000000000000, 0.000000000000000000 ) ) ;
#4573=B_SPLINE_SURFACE_WITH_KNOTS ( 'NONE', 5, 5, ( 
 ( #1099, #9939, #27740, #26687, #17210, #15001, #28566, #8735, #4090 ),
 ( #10618, #13259, #8601, #6577, #3952, #17652, #23772, #12676, #1775 ),
 ( #22166, #2206, #14865, #2071, #26533, #28422, #4240, #3814, #6418 ),
 ( #15142, #24050, #17358, #23915, #21725, #15282, #26102, #17504, #12958 ),
 ( #10482, #15438, #26389, #11050, #22023, #21872, #19965, #19394, #17796 ),
 ( #12815, #24204, #13112, #19534, #21587, #6128, #8455, #6276, #10910 ) ),
 .UNSPECIFIED., .F., .F., .F.,
 ( 6, 6 ),
 ( 6, 3, 6 ),
 ( 15.94303934750000096, 69.72897805040000208 ),
 ( 0.000000000000000000, 1.000000000000000000, 2.000000000000000000 ),
 .UNSPECIFIED. ) ;
#4574=B_SPLINE_CURVE_WITH_KNOTS ( 'NONE', 5,
 ( #25923, #12780, #17172, #17465, #26061, #3637, #15243, #24162, #6089, #4049, #19363, #26351, #19637, #5819, #4196, #14829, #13071, #1606 ),
 .UNSPECIFIED., .F., .F.,
 ( 6, 3, 3, 3, 3, 6 ),
 ( 0.000000000000000000, 1.124498255630000054, 2.252774941520000240, 3.380756636290000117, 4.508382774200000220, 5.576981603780000185 ),
 .UNSPECIFIED. ) ;
#4575=DIRECTION ( 'NONE',  ( 0.000000000000000000, 1.000000000000000000, 0.000000000000000000 ) ) ;
#4576=CARTESIAN_POINT ( 'NONE',  ( -12.61432613040000028, -66.29767256870000836, -22.40516107950000091 ) ) ;
#4578=CARTESIAN_POINT ( 'NONE',  ( -10.20110288159999890, -84.00000000000000000, -41.00000000000000000 ) ) ;
#4580=ORIENTED_EDGE ( 'NONE', *, *, #19698, .F. ) ;
#4582=CARTESIAN_POINT ( 'NONE',  ( 36.25015153569999882, -74.79528478139999947, -15.04955598449999954 ) ) ;
#4583=VECTOR ( 'NONE', #17765, 1000.000000000000000 ) ;
#4584=VECTOR ( 'NONE', #952, 1000.000000000000000 ) ;
#4587=CARTESIAN_POINT ( 'NONE',  ( -14.88246912999999871, -67.03279743669999391, 22.48335306070000073 ) ) ;
#4588=DIRECTION ( 'NONE',  ( 0.000000000000000000, -1.000000000000000000, 0.000000000000000000 ) ) ;
#4589=CARTESIAN_POINT ( 'NONE',  ( 7.242418264991816734, -74.21175622417943885, 40.33192879158703192 ) ) ;
#4593=VERTEX_POINT ( 'NONE', #21971 ) ;
#4594=B_SPLINE_CURVE_WITH_KNOTS ( 'NONE', 3,
 ( #4294, #8225, #21928, #14914, #15338, #22214 ),
 .UNSPECIFIED., .F., .F.,
 ( 4, 2, 4 ),
 ( 0.000000000000000000, 0.5000000000000000000, 1.000000000000000000 ),
 .UNSPECIFIED. ) ;
#4596=CARTESIAN_POINT ( 'NONE',  ( 7.219507042790000106, -73.62951539670000045, -39.18035607859999914 ) ) ;
#4597=ORIENTED_EDGE ( 'NONE', *, *, #18469, .F. ) ;
#4602=CARTESIAN_POINT ( 'NONE',  ( -9.762708992400000341, -18.50000000000000000, -19.20397640299999864 ) ) ;
#4603=EDGE_CURVE ( 'NONE', #13115, #26201, #16701, .T. ) ;
#4605=CARTESIAN_POINT ( 'NONE',  ( -7.234868202896564071, -73.70809116070437028, -39.52985788730124739 ) ) ;
#4606=EDGE_CURVE ( 'NONE', #8919, #19884, #8319, .T. ) ;
#4607=CARTESIAN_POINT ( 'NONE',  ( 20.73142793440000275, -60.32026811789999954, 11.32541297100000044 ) ) ;
#4608=DIRECTION ( 'NONE',  ( -0.7071067811865474617, 0.000000000000000000, 0.7071067811865474617 ) ) ;
#4614=CARTESIAN_POINT ( 'NONE',  ( 20.56960363573175243, -19.47131810281557307, 9.532984917462295371 ) ) ;
#4616=ORIENTED_EDGE ( 'NONE', *, *, #1278, .T. ) ;
#4618=AXIS2_PLACEMENT_3D ( 'NONE', #21047, #16073, #11852 ) ;
#4620=ORIENTED_EDGE ( 'NONE', *, *, #15788, .F. ) ;
#4621=CIRCLE ( 'NONE', #8299, 7.249999999999999112 ) ;
#4623=TOROIDAL_SURFACE ( 'NONE', #28342, 9.000000000000000000, 2.000000000000000000 ) ;
#4625=DIRECTION ( 'NONE',  ( 1.000000000000000000, 0.000000000000000000, 0.000000000000000000 ) ) ;
#4626=CARTESIAN_POINT ( 'NONE',  ( 19.64679318960000032, -35.95469792330000303, -9.266762188240001308 ) ) ;
#4630=CARTESIAN_POINT ( 'NONE',  ( -22.90089770769782618, -70.95732848294369433, 15.81452471505874158 ) ) ;
#4632=FACE_OUTER_BOUND ( 'NONE', #8473, .T. ) ;
#4633=ORIENTED_EDGE ( 'NONE', *, *, #21807, .T. ) ;
#4634=DIRECTION ( 'NONE',  ( 0.000000000000000000, 1.000000000000000000, 0.000000000000000000 ) ) ;
#4635=CARTESIAN_POINT ( 'NONE',  ( -22.13232309480000026, -79.66742592930000910, -32.73892524850000285 ) ) ;
#4641=EDGE_CURVE ( 'NONE', #452, #11938, #24629, .T. ) ;
#4643=DIRECTION ( 'NONE',  ( 0.9704142011833034598, 0.000000000000000000, -0.2414462220490750932 ) ) ;
#4645=CARTESIAN_POINT ( 'NONE',  ( -2.565530488230000294, -57.41946977150000464, -24.92670969510000134 ) ) ;
#4648=CARTESIAN_POINT ( 'NONE',  ( -18.56585641370000062, -19.46390881170000142, 11.87275530319999817 ) ) ;
#4649=ORIENTED_EDGE ( 'NONE', *, *, #2009, .F. ) ;
#4652=FACE_OUTER_BOUND ( 'NONE', #28454, .T. ) ;
#4653=DIRECTION ( 'NONE',  ( 0.000000000000000000, -1.000000000000000000, 0.000000000000000000 ) ) ;
#4654=CARTESIAN_POINT ( 'NONE',  ( 47.11905485129999960, -79.66016163019999397, -1.826180561010000147 ) ) ;
#4656=CIRCLE ( 'NONE', #16284, 3.750000000000000000 ) ;
#4657=LINE ( 'NONE', #2492, #90 ) ;
#4658=CARTESIAN_POINT ( 'NONE',  ( -11.67870406890000012, -57.47571038070000782, -20.30949878500000239 ) ) ;
#4660=ORIENTED_EDGE ( 'NONE', *, *, #9104, .F. ) ;
#4661=ADVANCED_FACE ( 'NONE', ( #4632 ), #20430, .T. ) ;
#4662=DIRECTION ( 'NONE',  ( 0.9704142011833030157, 0.000000000000000000, -0.2414462220490760924 ) ) ;
#4664=ORIENTED_EDGE ( 'NONE', *, *, #8307, .T. ) ;
#4666=CARTESIAN_POINT ( 'NONE',  ( 8.916781105359106618, -18.97801339259782338, -18.93583224184311220 ) ) ;
#4668=DIRECTION ( 'NONE',  ( -1.000000000000000000, 0.000000000000000000, 1.286327366459999920E-15 ) ) ;
#4670=CARTESIAN_POINT ( 'NONE',  ( 8.721287999440001215, -37.33944922460000271, -21.87060590859999820 ) ) ;
#4673=CARTESIAN_POINT ( 'NONE',  ( 21.47791241899999903, -36.56811125080000835, -7.356933755090000027 ) ) ;
#4675=DIRECTION ( 'NONE',  ( -0.8775825618903722036, 0.000000000000000000, 0.4794255386042041156 ) ) ;
#4677=CARTESIAN_POINT ( 'NONE',  ( -20.41203979210912678, -61.51300819583687485, 12.46450689150019286 ) ) ;
#4678=CARTESIAN_POINT ( 'NONE',  ( -32.77174709959999888, -74.43710720380001078, -21.60034937849999892 ) ) ;
#4679=ORIENTED_EDGE ( 'NONE', *, *, #3792, .T. ) ;
#4683=DIRECTION ( 'NONE',  ( 0.000000000000000000, 1.000000000000000000, 0.000000000000000000 ) ) ;
#4685=AXIS2_PLACEMENT_3D ( 'NONE', #16923, #8169, #26522 ) ;
#4687=AXIS2_PLACEMENT_3D ( 'NONE', #27950, #7725, #18650 ) ;
#4689=CARTESIAN_POINT ( 'NONE',  ( 9.099148368519999863, -57.44066836780000074, -22.71963871379999844 ) ) ;
#4691=DIRECTION ( 'NONE',  ( 1.000000000000000000, 0.000000000000000000, 5.551115123129980921E-17 ) ) ;
#4692=CARTESIAN_POINT ( 'NONE',  ( -11.74918180529999923, -34.66943697800000734, -19.26448814340000126 ) ) ;
#4694=DIRECTION ( 'NONE',  ( 1.000000000000000000, 0.000000000000000000, 0.000000000000000000 ) ) ;
#4695=EDGE_LOOP ( 'NONE', ( #10714, #5228, #22393, #28228 ) ) ;
#4696=EDGE_CURVE ( 'NONE', #26457, #9687, #17458, .T. ) ;
#4698=CARTESIAN_POINT ( 'NONE',  ( 24.58030493329999899, -18.50000000000000000, 2.442848308399999890 ) ) ;
#4701=CARTESIAN_POINT ( 'NONE',  ( 7.279135155890000597, -73.90050421709999284, 39.59102417159999021 ) ) ;
#4703=VECTOR ( 'NONE', #9577, 1000.000000000000000 ) ;
#4704=AXIS2_PLACEMENT_3D ( 'NONE', #1903, #25432, #5460 ) ;
#4710=CARTESIAN_POINT ( 'NONE',  ( 8.704479342339999093, -36.45005858900000106, -21.20784114439999968 ) ) ;
#4712=CARTESIAN_POINT ( 'NONE',  ( 0.000000000000000000, -57.47855601759999900, 0.000000000000000000 ) ) ;
#4715=FACE_OUTER_BOUND ( 'NONE', #9301, .T. ) ;
#4716=CARTESIAN_POINT ( 'NONE',  ( -2.585842044862892042, -19.48733830549529600, -23.57049848989026231 ) ) ;
#4719=CARTESIAN_POINT ( 'NONE',  ( -13.37241048499999962, -18.62107966670000181, 19.38866880850000030 ) ) ;
#4722=DIRECTION ( 'NONE',  ( 1.000000000000000000, 0.000000000000000000, 0.000000000000000000 ) ) ;
#4724=CARTESIAN_POINT ( 'NONE',  ( 9.356041104380000917, -74.50000000000000000, -37.60355029590000697 ) ) ;
#4725=CYLINDRICAL_SURFACE ( 'NONE', #23103, 11.00000000000000000 ) ;
#4730=VECTOR ( 'NONE', #19381, 1000.000000000000000 ) ;
#4735=CARTESIAN_POINT ( 'NONE',  ( -12.24787727680000060, -65.07443125830000952, 21.96585809910000009 ) ) ;
#4736=CARTESIAN_POINT ( 'NONE',  ( -13.48313256510000002, -64.78279493179998383, 21.61455522920000050 ) ) ;
#4738=CARTESIAN_POINT ( 'NONE',  ( -2.495716009669999735, -52.58489974409944523, -24.49317771889998241 ) ) ;
#4739=ADVANCED_FACE ( 'NONE', ( #26343 ), #13089, .T. ) ;
#4740=CARTESIAN_POINT ( 'NONE',  ( 22.17953377930000158, -65.07443093669999712, 11.85657293289999892 ) ) ;
#4745=CARTESIAN_POINT ( 'NONE',  ( -7.255215663259999559, -74.34471143260000758, -40.30304758909999663 ) ) ;
#4749=EDGE_CURVE ( 'NONE', #14143, #16936, #12472, .T. ) ;
#4751=CARTESIAN_POINT ( 'NONE',  ( -13.13725193384587264, -67.22652123493047327, -22.58921519140665168 ) ) ;
#4754=B_SPLINE_CURVE_WITH_KNOTS ( 'NONE', 3,
 ( #1814, #13003, #21627, #1963, #15475, #23810 ),
 .UNSPECIFIED., .F., .F.,
 ( 4, 2, 4 ),
 ( 0.000000000000000000, 0.5000000000000000000, 1.000000000000000000 ),
 .UNSPECIFIED. ) ;
#4755=DIRECTION ( 'NONE',  ( 0.000000000000000000, -1.000000000000000000, 0.000000000000000000 ) ) ;
#4756=DIRECTION ( 'NONE',  ( 1.000000000000000000, 0.000000000000000000, 0.000000000000000000 ) ) ;
#4758=CARTESIAN_POINT ( 'NONE',  ( -7.218875474177550267, -73.62261561668539400, -39.32889484839753180 ) ) ;
#4759=CARTESIAN_POINT ( 'NONE',  ( 20.91100902960000241, -19.47458110719999880, 9.394602247639998183 ) ) ;
#4763=VERTEX_POINT ( 'NONE', #7568 ) ;
#4764=CARTESIAN_POINT ( 'NONE',  ( -12.22902281400000035, -69.69726684059999400, -24.77074626769999810 ) ) ;
#4767=CARTESIAN_POINT ( 'NONE',  ( 20.23144668435722338, -19.46809228182657492, 9.669420246545856301 ) ) ;
#4770=CIRCLE ( 'NONE', #21066, 32.39999999999999858 ) ;
#4779=ADVANCED_FACE ( 'NONE', ( #16428 ), #9716, .T. ) ;
#4780=ORIENTED_EDGE ( 'NONE', *, *, #10822, .F. ) ;
#4783=CARTESIAN_POINT ( 'NONE',  ( 46.85366533689999358, -73.91963657849998981, -2.428543975460000226 ) ) ;
#4786=CARTESIAN_POINT ( 'NONE',  ( -22.07482501520000184, -79.88234130290000223, -32.63328169969999948 ) ) ;
#4787=ADVANCED_FACE ( 'NONE', ( #21103 ), #14390, .F. ) ;
#4788=CIRCLE ( 'NONE', #16892, 3.750000000000000000 ) ;
#4794=FACE_OUTER_BOUND ( 'NONE', #22376, .T. ) ;
#4796=CARTESIAN_POINT ( 'NONE',  ( -39.59102417159999021, -73.90050421709999284, 7.279135155890000597 ) ) ;
#4797=CARTESIAN_POINT ( 'NONE',  ( -22.00249031559999935, -74.50000000000000000, -32.67527180329999936 ) ) ;
#4800=CARTESIAN_POINT ( 'NONE',  ( -7.485155838150649110, -73.99989100306002854, 38.96201482635396474 ) ) ;
#4802=ORIENTED_EDGE ( 'NONE', *, *, #22374, .F. ) ;
#4803=DIRECTION ( 'NONE',  ( 0.000000000000000000, -1.000000000000000000, 0.000000000000000000 ) ) ;
#4805=CARTESIAN_POINT ( 'NONE',  ( 22.87354612120000041, -62.62089253239999920, 10.49332266949999948 ) ) ;
#4806=FACE_OUTER_BOUND ( 'NONE', #13223, .T. ) ;
#4809=ORIENTED_EDGE ( 'NONE', *, *, #27665, .T. ) ;
#4810=CARTESIAN_POINT ( 'NONE',  ( 47.25120111029999492, -79.32896547530000930, -0.9107464912380001110 ) ) ;
#4812=CARTESIAN_POINT ( 'NONE',  ( -11.84069971089999918, -64.35840483370000698, -23.45279569499999894 ) ) ;
#4814=DIRECTION ( 'NONE',  ( -0.7071067811865475727, 0.000000000000000000, -0.7071067811865475727 ) ) ;
#4815=DIRECTION ( 'NONE',  ( 0.000000000000000000, -1.000000000000000000, 0.000000000000000000 ) ) ;
#4818=CARTESIAN_POINT ( 'NONE',  ( 40.00000000000000000, -84.00000000000000000, 0.000000000000000000 ) ) ;
#4819=CARTESIAN_POINT ( 'NONE',  ( 46.80987811986599212, -73.90819598650089972, -2.489252664572485951 ) ) ;
#4821=CARTESIAN_POINT ( 'NONE',  ( 27.75394116159999669, -74.50000000000000000, -27.75394116159999669 ) ) ;
#4822=CARTESIAN_POINT ( 'NONE',  ( -17.94180966909999597, -19.50000000000000000, 18.81731824139999887 ) ) ;
#4825=EDGE_CURVE ( 'NONE', #3611, #9035, #5423, .T. ) ;
#4828=CARTESIAN_POINT ( 'NONE',  ( 9.014522480169999241, -36.52810941340000284, -21.48399575520000226 ) ) ;
#4830=CARTESIAN_POINT ( 'NONE',  ( -9.489637567029999943, -18.50000000000000000, -21.46212729140000164 ) ) ;
#4831=CARTESIAN_POINT ( 'NONE',  ( 21.53322619567358487, -37.52465077453045694, -7.784903219023103560 ) ) ;
#4836=ORIENTED_EDGE ( 'NONE', *, *, #17334, .T. ) ;
#4838=CARTESIAN_POINT ( 'NONE',  ( -7.215414233289999757, -80.50000000000000000, 40.70731707320000226 ) ) ;
#4839=CARTESIAN_POINT ( 'NONE',  ( -21.66710847110000060, -65.28157844300000079, 15.85023555240000093 ) ) ;
#4842=EDGE_CURVE ( 'NONE', #18987, #25992, #27791, .T. ) ;
#4843=CARTESIAN_POINT ( 'NONE',  ( -19.61616312839999665, -45.99906616869999709, 11.93235103359999982 ) ) ;
#4844=CARTESIAN_POINT ( 'NONE',  ( 26.07817510496859725, -74.32881829746334290, -29.29368945734479013 ) ) ;
#4845=CARTESIAN_POINT ( 'NONE',  ( -12.47290128200000048, -69.87861801290000585, -24.46965308400000083 ) ) ;
#4846=CARTESIAN_POINT ( 'NONE',  ( -14.77602055539237647, -74.24330531883769879, 36.28595032296689027 ) ) ;
#4847=CIRCLE ( 'NONE', #14145, 1.499999999999999556 ) ;
#4848=DIRECTION ( 'NONE',  ( 0.7071067811865492381, 0.000000000000000000, -0.7071067811865457964 ) ) ;
#4849=AXIS2_PLACEMENT_3D ( 'NONE', #409, #6952, #15213 ) ;
#4850=EDGE_LOOP ( 'NONE', ( #24237, #333, #25194, #7191 ) ) ;
#4853=CARTESIAN_POINT ( 'NONE',  ( 24.18500510740000209, -18.50000000000000000, 2.499651262099999993 ) ) ;
#4855=ORIENTED_EDGE ( 'NONE', *, *, #19435, .F. ) ;
#4857=CARTESIAN_POINT ( 'NONE',  ( 7.305170733980000719, -74.19145785139998850, 39.89387480210000092 ) ) ;
#4859=EDGE_CURVE ( 'NONE', #7605, #3896, #21509, .T. ) ;
#4860=CARTESIAN_POINT ( 'NONE',  ( 22.36835622256649714, -19.46749651865001596, 0.6186015604048864525 ) ) ;
#4861=CARTESIAN_POINT ( 'NONE',  ( 8.971088436049999615, -36.01992746820000235, -20.53904558130000169 ) ) ;
#4862=CARTESIAN_POINT ( 'NONE',  ( 8.542193844259857727, -19.47739189591211328, -20.07101182275077633 ) ) ;
#4863=ORIENTED_EDGE ( 'NONE', *, *, #21508, .F. ) ;
#4865=CARTESIAN_POINT ( 'NONE',  ( 23.56381625550000081, -19.17416318749999959, 1.511209194469999906 ) ) ;
#4867=VECTOR ( 'NONE', #13927, 1000.000000000000000 ) ;
#4868=CARTESIAN_POINT ( 'NONE',  ( -1.557368374968634228, -19.46665351424891455, -22.24853037986929394 ) ) ;
#4869=FACE_OUTER_BOUND ( 'NONE', #2326, .T. ) ;
#4870=CARTESIAN_POINT ( 'NONE',  ( -13.09065259650000002, -19.17416291640000026, 19.65126003909999852 ) ) ;
#4871=CARTESIAN_POINT ( 'NONE',  ( -41.00000000000000000, -84.00000000000000000, 10.20110288159999890 ) ) ;
#4873=EDGE_CURVE ( 'NONE', #15079, #7833, #28657, .T. ) ;
#4875=CIRCLE ( 'NONE', #25361, 3.000000000000000000 ) ;
#4879=CARTESIAN_POINT ( 'NONE',  ( 36.71193690820000199, -74.86352340930001503, -14.74418008200000152 ) ) ;
#4882=EDGE_CURVE ( 'NONE', #8136, #6525, #19944, .T. ) ;
#4883=CARTESIAN_POINT ( 'NONE',  ( -12.07243358760000085, -67.46050599719998786, -24.77970463289999969 ) ) ;
#4886=CARTESIAN_POINT ( 'NONE',  ( 20.85226889450000343, -36.17942473059999742, -9.018047964759999147 ) ) ;
#4887=CARTESIAN_POINT ( 'NONE',  ( -1.456904695350001111, -52.62618816489944606, -23.34673678599997970 ) ) ;
#4888=CARTESIAN_POINT ( 'NONE',  ( 20.77909565649999735, -36.00000000010000178, -9.444780804769999705 ) ) ;
#4890=VERTEX_POINT ( 'NONE', #19983 ) ;
#4891=CARTESIAN_POINT ( 'NONE',  ( 21.49478534619999692, -36.56947956670000366, -7.151043357429999858 ) ) ;
#4894=CARTESIAN_POINT ( 'NONE',  ( 23.14416696340000001, -57.40875702419999982, 10.37855830930000067 ) ) ;
#4899=CARTESIAN_POINT ( 'NONE',  ( -7.249276399919747149, -74.06318173121573523, -40.12703402648163831 ) ) ;
#4901=CARTESIAN_POINT ( 'NONE',  ( 10.64645172839999887, -72.61900946069999918, -26.72437960700000303 ) ) ;
#4904=CARTESIAN_POINT ( 'NONE',  ( -12.79457676070000183, -70.02558174150000525, -24.23940011709999709 ) ) ;
#4908=CARTESIAN_POINT ( 'NONE',  ( 21.27121383927310205, -19.48034373448365741, 9.460266570831914024 ) ) ;
#4909=CARTESIAN_POINT ( 'NONE',  ( 22.54638839685503271, -60.33833132835033553, -7.163837719818888061 ) ) ;
#4913=ORIENTED_EDGE ( 'NONE', *, *, #11083, .F. ) ;
#4914=EDGE_CURVE ( 'NONE', #4550, #19124, #5995, .T. ) ;
#4917=DIRECTION ( 'NONE',  ( 1.000000000000000000, 0.000000000000000000, 0.000000000000000000 ) ) ;
#4920=ORIENTED_EDGE ( 'NONE', *, *, #8637, .T. ) ;
#4922=CARTESIAN_POINT ( 'NONE',  ( 36.24656966590000451, -75.00000018780001199, -15.05817676390000059 ) ) ;
#4924=CARTESIAN_POINT ( 'NONE',  ( 47.16888057639999943, -74.56821146769999586, -1.104573556149999858 ) ) ;
#4932=CARTESIAN_POINT ( 'NONE',  ( 36.50549978619999791, -74.62369759450000117, -14.71598446109999969 ) ) ;
#4934=CARTESIAN_POINT ( 'NONE',  ( 40.00000000000000000, -74.00000000000000000, 2.009834509230000106E-15 ) ) ;
#4935=CARTESIAN_POINT ( 'NONE',  ( -21.99985828019999801, -74.00000000000000000, -31.89935321680000158 ) ) ;
#4939=CARTESIAN_POINT ( 'NONE',  ( -7.499802406392214849, -73.99986890635469194, 38.92495601869831034 ) ) ;
#4940=CARTESIAN_POINT ( 'NONE',  ( -18.23016591169999856, -18.61940624670000233, 13.57443799729999867 ) ) ;
#4947=CARTESIAN_POINT ( 'NONE',  ( 28.63360765790000073, -72.82938648530000592, 1.697648101029999967 ) ) ;
#4948=ORIENTED_EDGE ( 'NONE', *, *, #22750, .F. ) ;
#4949=CARTESIAN_POINT ( 'NONE',  ( 47.25000000000000000, -79.00000000000000000, -7.713829575100000215E-13 ) ) ;
#4951=ADVANCED_FACE ( 'NONE', ( #24663 ), #2187, .T. ) ;
#4952=CARTESIAN_POINT ( 'NONE',  ( -12.00178822160000003, -62.10499660389999832, -20.82579118980000032 ) ) ;
#4953=CARTESIAN_POINT ( 'NONE',  ( 26.98670340789999855, -72.82938977469999031, -9.720255250700001071 ) ) ;
#4960=ORIENTED_EDGE ( 'NONE', *, *, #3856, .F. ) ;
#4961=CARTESIAN_POINT ( 'NONE',  ( -7.215414233289999757, -82.25000000000000000, -40.70731707320000226 ) ) ;
#4962=CARTESIAN_POINT ( 'NONE',  ( 19.55068592539999983, -35.72724453810000256, -9.038647860560001135 ) ) ;
#4967=CYLINDRICAL_SURFACE ( 'NONE', #7879, 2.999999999999996447 ) ;
#4968=VERTEX_POINT ( 'NONE', #232 ) ;
#4971=CARTESIAN_POINT ( 'NONE',  ( 40.08893529097915120, -74.03750509247994671, 7.249551406115140928 ) ) ;
#4976=ORIENTED_EDGE ( 'NONE', *, *, #23341, .T. ) ;
#4979=CARTESIAN_POINT ( 'NONE',  ( -18.92164427849999697, -32.73099401719999690, 12.31425843260000086 ) ) ;
#4980=DIRECTION ( 'NONE',  ( 0.000000000000000000, -1.000000000000000000, 0.000000000000000000 ) ) ;
#4981=CARTESIAN_POINT ( 'NONE',  ( 31.03260167810000070, -72.62832455090000394, -20.30285101509999990 ) ) ;
#4984=ORIENTED_EDGE ( 'NONE', *, *, #11303, .F. ) ;
#4985=CARTESIAN_POINT ( 'NONE',  ( 9.212281862759999385, -37.98196146859999800, -22.49242731490000224 ) ) ;
#4988=DIRECTION ( 'NONE',  ( 0.000000000000000000, 1.000000000000000000, 0.000000000000000000 ) ) ;
#4990=CARTESIAN_POINT ( 'NONE',  ( -34.71422205039999653, -79.50000000000000000, -24.10762033259999981 ) ) ;
#4993=CARTESIAN_POINT ( 'NONE',  ( 24.03793476618687919, -19.49371143355231339, 1.498876886815959431 ) ) ;
#4996=CARTESIAN_POINT ( 'NONE',  ( 8.441591539670000088, -37.31515243520000524, -21.68264306949999920 ) ) ;
#4997=CARTESIAN_POINT ( 'NONE',  ( 45.84677419350000349, -73.50000000000000000, -4.286925650119999709 ) ) ;
#4999=TOROIDAL_SURFACE ( 'NONE', #5915, 3.750000000000000000, 1.000000000000000000 ) ;
#5001=CARTESIAN_POINT ( 'NONE',  ( -40.70731707320000226, -82.25000000000000000, -7.215414233289999757 ) ) ;
#5002=CARTESIAN_POINT ( 'NONE',  ( -12.28242885148121566, -19.47294316487861821, 19.19149835041444874 ) ) ;
#5003=DIRECTION ( 'NONE',  ( 0.9993816408608721114, 0.000000000000000000, -0.03516156865429537204 ) ) ;
#5004=DIRECTION ( 'NONE',  ( 1.000000000000000000, 0.000000000000000000, 0.000000000000000000 ) ) ;
#5006=FACE_OUTER_BOUND ( 'NONE', #21251, .T. ) ;
#5008=EDGE_CURVE ( 'NONE', #13409, #12777, #12361, .T. ) ;
#5009=DIRECTION ( 'NONE',  ( 0.4692400087391615515, 0.000000000000000000, -0.8830706733883034731 ) ) ;
#5010=CIRCLE ( 'NONE', #21295, 0.4999999999999967804 ) ;
#5012=CARTESIAN_POINT ( 'NONE',  ( 21.85814127600000134, -49.11291935110000395, -7.592835430120000062 ) ) ;
#5014=CARTESIAN_POINT ( 'NONE',  ( 8.770435879969156190, -35.38531427029693077, -20.52569411805346178 ) ) ;
#5016=ORIENTED_EDGE ( 'NONE', *, *, #14232, .T. ) ;
#5017=CARTESIAN_POINT ( 'NONE',  ( 36.72991148340000223, -74.73026516779999895, -14.71529450729999944 ) ) ;
#5019=CARTESIAN_POINT ( 'NONE',  ( -22.33509239084705555, -79.80951032333221917, -32.79088695412508514 ) ) ;
#5020=B_SPLINE_CURVE_WITH_KNOTS ( 'NONE', 3,
 ( #28267, #17204, #6267, #15133, #2060, #10900, #24042, #19808, #4080, #12949, #28687, #21860, #1912, #20112, #22420, #11764, #1427 ),
 .UNSPECIFIED., .F., .F.,
 ( 4, 2, 2, 1, 1, 1, 1, 1, 2, 2, 4 ),
 ( 0.000000000000000000, 0.2499999999997198352, 0.3749999999995797806, 0.4374999999995097255, 0.4687499999994720890, 0.4843749999994530486, 0.4921874999994436117, 0.4960937499994417799, 0.4980468749994406141, 0.4999999999994395039, 1.000000000000000000 ),
 .UNSPECIFIED. ) ;
#5022=CARTESIAN_POINT ( 'NONE',  ( -15.22757417880000119, -66.82180077600000345, 22.72230046389999814 ) ) ;
#5023=CARTESIAN_POINT ( 'NONE',  ( 8.346327226119999665, -35.76750032119999645, -21.11704210819999972 ) ) ;
#5024=CARTESIAN_POINT ( 'NONE',  ( -2.337241308500000336, -64.69849383090000572, -25.49681307870000069 ) ) ;
#5025=CIRCLE ( 'NONE', #8711, 8.999999999999998224 ) ;
#5026=CARTESIAN_POINT ( 'NONE',  ( 26.43538883845638665, -72.55114739962129988, 11.02537517961439839 ) ) ;
#5027=CARTESIAN_POINT ( 'NONE',  ( 20.11250903250000022, -36.00000000000000000, -9.561259576869998611 ) ) ;
#5030=ORIENTED_EDGE ( 'NONE', *, *, #734, .T. ) ;
#5031=CARTESIAN_POINT ( 'NONE',  ( 21.46601194620000186, -36.21205870680000061, -7.351927201700000580 ) ) ;
#5033=VERTEX_POINT ( 'NONE', #7206 ) ;
#5035=ORIENTED_EDGE ( 'NONE', *, *, #20019, .T. ) ;
#5036=LINE ( 'NONE', #22677, #4867 ) ;
#5038=DIRECTION ( 'NONE',  ( 0.000000000000000000, 1.000000000000000000, 0.000000000000000000 ) ) ;
#5039=CARTESIAN_POINT ( 'NONE',  ( -7.247546674761930596, -74.11886065900105791, -40.20585889325029427 ) ) ;
#5041=CARTESIAN_POINT ( 'NONE',  ( -14.46844930820000030, -74.19081742459999873, 36.42578001110000230 ) ) ;
#5042=CARTESIAN_POINT ( 'NONE',  ( -22.29197733299999840, -68.17313230439998506, 14.44572620890000003 ) ) ;
#5043=CARTESIAN_POINT ( 'NONE',  ( -13.53684476099999934, -28.27010607350000271, 20.60385118230000145 ) ) ;
#5045=CIRCLE ( 'NONE', #21332, 10.50000000000000000 ) ;
#5047=CARTESIAN_POINT ( 'NONE',  ( 7.680652413499999831, -31.56454373169999883, -21.10194041029999923 ) ) ;
#5048=CARTESIAN_POINT ( 'NONE',  ( -7.443137591229999295, -74.00000000000000000, 35.37770683939999827 ) ) ;
#5055=CARTESIAN_POINT ( 'NONE',  ( -12.67352077070000149, -74.00000000000000000, 33.30278006909999533 ) ) ;
#5058=ORIENTED_EDGE ( 'NONE', *, *, #8972, .F. ) ;
#5062=CARTESIAN_POINT ( 'NONE',  ( -23.14039283085165266, -72.53276285757912945, 16.72032736073078851 ) ) ;
#5063=CARTESIAN_POINT ( 'NONE',  ( -14.29547445250000060, -80.00000000000000000, 45.69901703040000029 ) ) ;
#5064=CARTESIAN_POINT ( 'NONE',  ( 11.31764174110000098, -36.00000000000000000, -22.43277175240000076 ) ) ;
#5067=CARTESIAN_POINT ( 'NONE',  ( -11.45377175261103631, -61.32605129436165470, 20.94518220247841711 ) ) ;
#5069=VERTEX_POINT ( 'NONE', #5309 ) ;
#5070=CARTESIAN_POINT ( 'NONE',  ( 23.98990767258865375, -64.35840732026599653, 10.71073183009686858 ) ) ;
#5072=CARTESIAN_POINT ( 'NONE',  ( -2.984168974620000192, -69.33908554340000308, -27.31525404649999800 ) ) ;
#5074=CARTESIAN_POINT ( 'NONE',  ( -15.68940877609999873, -70.60291157129999817, 23.18755817509999773 ) ) ;
#5077=CARTESIAN_POINT ( 'NONE',  ( -12.09704001540000107, -79.50000000000000000, 47.10905722069999513 ) ) ;
#5078=CARTESIAN_POINT ( 'NONE',  ( 24.89712376119999959, -63.41220263479998920, 0.7891782316930000540 ) ) ;
#5079=CARTESIAN_POINT ( 'NONE',  ( -21.86233684099999763, -74.36373701399999447, -32.64238205049999664 ) ) ;
#5080=EDGE_LOOP ( 'NONE', ( #27622, #9216, #7491, #4567 ) ) ;
#5081=AXIS2_PLACEMENT_3D ( 'NONE', #2222, #2090, #4694 ) ;
#5082=DIRECTION ( 'NONE',  ( -1.000000000000000000, 0.000000000000000000, 5.075305255429999693E-16 ) ) ;
#5084=CARTESIAN_POINT ( 'NONE',  ( 36.61058569223673942, -74.16120954504201279, -14.29449953322217048 ) ) ;
#5086=CIRCLE ( 'NONE', #2298, 23.36116116979999902 ) ;
#5088=DIRECTION ( 'NONE',  ( -1.000000000000000000, 0.000000000000000000, 0.000000000000000000 ) ) ;
#5089=B_SPLINE_CURVE_WITH_KNOTS ( 'NONE', 3,
 ( #10849, #6358, #3893, #28220 ),
 .UNSPECIFIED., .F., .F.,
 ( 4, 4 ),
 ( -3.225498864409999999, -2.709627031390000163 ),
 .UNSPECIFIED. ) ;
#5090=CIRCLE ( 'NONE', #15274, 25.14975229270000057 ) ;
#5091=CARTESIAN_POINT ( 'NONE',  ( 23.15160389369999905, -62.53529079469999630, 10.48384440070000068 ) ) ;
#5092=FACE_OUTER_BOUND ( 'NONE', #20221, .T. ) ;
#5096=CARTESIAN_POINT ( 'NONE',  ( 20.94731949980000252, -52.62618816490000029, 10.41165191589999850 ) ) ;
#5098=CARTESIAN_POINT ( 'NONE',  ( -11.40956707329999809, -19.15825154520000240, 19.02831704529999968 ) ) ;
#5099=CARTESIAN_POINT ( 'NONE',  ( -11.65869911329999908, -63.24100619559999359, -22.48820904579999791 ) ) ;
#5100=SPHERICAL_SURFACE ( 'NONE', #15, 1.000000000000000000 ) ;
#5101=DIRECTION ( 'NONE',  ( -1.000000000000000000, 0.000000000000000000, 0.000000000000000000 ) ) ;
#5103=CARTESIAN_POINT ( 'NONE',  ( 10.87364956280000072, -37.98927800880000660, 19.90408201490000195 ) ) ;
#5106=EDGE_LOOP ( 'NONE', ( #4028, #17306, #4984, #20070 ) ) ;
#5107=CARTESIAN_POINT ( 'NONE',  ( 23.03829042120000281, -52.56313962730000355, 10.32398954119999956 ) ) ;
#5110=ADVANCED_FACE ( 'NONE', ( #5006 ), #23684, .T. ) ;
#5113=ADVANCED_FACE ( 'NONE', ( #20456 ), #8434, .T. ) ;
#5115=CARTESIAN_POINT ( 'NONE',  ( -0.5354892050589999952, -54.24814459719999604, -23.24218483219999953 ) ) ;
#5116=DIRECTION ( 'NONE',  ( 0.000000000000000000, 1.000000000000000000, 0.000000000000000000 ) ) ;
#5119=CARTESIAN_POINT ( 'NONE',  ( -10.25754198879999990, -18.86159979430000178, -20.74776445359999855 ) ) ;
#5120=CARTESIAN_POINT ( 'NONE',  ( 9.794085904993929503, -62.04428797445658716, -24.13968230914114343 ) ) ;
#5121=EDGE_LOOP ( 'NONE', ( #16180, #15140, #10621, #19728, #21896 ) ) ;
#5124=B_SPLINE_CURVE_WITH_KNOTS ( 'NONE', 5,
 ( #27308, #666, #13596, #20452, #7203, #8924 ),
 .UNSPECIFIED., .F., .F.,
 ( 6, 6 ),
 ( 0.000000000000000000, 1.000000000000000000 ),
 .UNSPECIFIED. ) ;
#5125=CARTESIAN_POINT ( 'NONE',  ( -20.44377240776747584, -61.67331079074745759, 12.48822562784140011 ) ) ;
#5126=CYLINDRICAL_SURFACE ( 'NONE', #10690, 0.5000000000000004441 ) ;
#5130=FACE_OUTER_BOUND ( 'NONE', #12351, .T. ) ;
#5133=FACE_OUTER_BOUND ( 'NONE', #3399, .T. ) ;
#5134=CARTESIAN_POINT ( 'NONE',  ( -12.79457955380000023, -70.02558078490001492, -24.23939601560000057 ) ) ;
#5135=CARTESIAN_POINT ( 'NONE',  ( 22.42217291749999930, -60.60023544439999910, -7.442794370989999742 ) ) ;
#5136=VECTOR ( 'NONE', #4988, 1000.000000000000000 ) ;
#5137=CARTESIAN_POINT ( 'NONE',  ( 26.22710519529999829, -65.11419048929998610, 1.448574456039999792 ) ) ;
#5140=DIRECTION ( 'NONE',  ( -0.2414462220490753985, 0.000000000000000000, 0.9704142011833032377 ) ) ;
#5141=CARTESIAN_POINT ( 'NONE',  ( 21.59295723509999831, -37.02888336210000375, -8.543455487960001093 ) ) ;
#5144=CARTESIAN_POINT ( 'NONE',  ( 7.256994698139999755, -74.37142462010000088, 40.28432270869999599 ) ) ;
#5147=CARTESIAN_POINT ( 'NONE',  ( 47.25063473080000165, -79.41040171960000293, -0.8747163666420000316 ) ) ;
#5150=DIRECTION ( 'NONE',  ( 0.2414462220490755373, 0.000000000000000000, 0.9704142011833032377 ) ) ;
#5151=CONICAL_SURFACE ( 'NONE', #24697, 21.99999999999999645, 0.03490658503990158590 ) ;
#5156=CARTESIAN_POINT ( 'NONE',  ( -39.46631086808643829, -73.67850591079914579, 7.230541818641200713 ) ) ;
#5157=AXIS2_PLACEMENT_3D ( 'NONE', #24769, #2919, #608 ) ;
#5158=CARTESIAN_POINT ( 'NONE',  ( 23.99083882220000064, -19.17999199609999650, 1.537804108040000006 ) ) ;
#5160=ORIENTED_EDGE ( 'NONE', *, *, #27869, .T. ) ;
#5161=CARTESIAN_POINT ( 'NONE',  ( -27.04683438039999999, -79.50000000000000000, -36.23922253580000330 ) ) ;
#5163=CARTESIAN_POINT ( 'NONE',  ( -2.079970928869999902, -32.71502530469999925, -23.05888968329999855 ) ) ;
#5165=DIRECTION ( 'NONE',  ( 0.8830706733883038062, 0.000000000000000000, 0.4692400087391607744 ) ) ;
#5166=DIRECTION ( 'NONE',  ( 0.000000000000000000, 1.000000000000000000, 0.000000000000000000 ) ) ;
#5168=CARTESIAN_POINT ( 'NONE',  ( -26.69328098980000163, -79.50000000000000000, -35.88566914520000495 ) ) ;
#5169=ORIENTED_EDGE ( 'NONE', *, *, #5850, .T. ) ;
#5170=CARTESIAN_POINT ( 'NONE',  ( -32.83566819349999832, -74.43710720380001078, -22.22906645439999807 ) ) ;
#5172=TOROIDAL_SURFACE ( 'NONE', #9818, 6.750000000000000000, 2.000000000000000000 ) ;
#5174=CIRCLE ( 'NONE', #19121, 0.5000000000000004441 ) ;
#5175=CARTESIAN_POINT ( 'NONE',  ( -13.09595933279999969, -66.29670474889999809, 22.12657759070000196 ) ) ;
#5176=CARTESIAN_POINT ( 'NONE',  ( 8.753525549769999969, -35.66748467180000404, -20.66368372700000222 ) ) ;
#5179=DIRECTION ( 'NONE',  ( 0.000000000000000000, -1.000000000000000000, 0.000000000000000000 ) ) ;
#5180=CARTESIAN_POINT ( 'NONE',  ( -40.70731707320000226, -74.50000000000000000, 7.215414233289999757 ) ) ;
#5181=EDGE_CURVE ( 'NONE', #3837, #20989, #21731, .T. ) ;
#5182=EDGE_CURVE ( 'NONE', #21366, #7391, #1652, .T. ) ;
#5187=DIRECTION ( 'NONE',  ( 1.000000000000000000, 0.000000000000000000, 0.000000000000000000 ) ) ;
#5188=EDGE_CURVE ( 'NONE', #15327, #20206, #12941, .T. ) ;
#5191=DIRECTION ( 'NONE',  ( 0.2414462220490755373, 0.000000000000000000, -0.9704142011833032377 ) ) ;
#5192=AXIS2_PLACEMENT_3D ( 'NONE', #15288, #24357, #26540 ) ;
#5193=CARTESIAN_POINT ( 'NONE',  ( -7.135467526410000261, -73.50000000000000000, -38.71641004229999794 ) ) ;
#5194=VECTOR ( 'NONE', #6671, 1000.000000000000000 ) ;
#5196=CARTESIAN_POINT ( 'NONE',  ( -14.51986742080000070, -74.16918790970001396, 36.33983588299999923 ) ) ;
#5197=CARTESIAN_POINT ( 'NONE',  ( -20.89470113539999829, -64.89165740699999674, 14.23290170900000007 ) ) ;
#5199=ORIENTED_EDGE ( 'NONE', *, *, #26685, .T. ) ;
#5201=CARTESIAN_POINT ( 'NONE',  ( 8.999623101399999214, -28.60070731709999947, -19.24185364099999873 ) ) ;
#5202=DIRECTION ( 'NONE',  ( 0.7414456417930908039, 0.000000000000000000, 0.6710129359900831592 ) ) ;
#5204=CARTESIAN_POINT ( 'NONE',  ( -38.71640952649999434, -73.65708014139998738, -7.135466514619999145 ) ) ;
#5205=ORIENTED_EDGE ( 'NONE', *, *, #9166, .T. ) ;
#5206=EDGE_CURVE ( 'NONE', #10474, #12521, #4146, .T. ) ;
#5207=ORIENTED_EDGE ( 'NONE', *, *, #5941, .F. ) ;
#5210=CARTESIAN_POINT ( 'NONE',  ( 0.000000000000000000, -82.50000000000000000, 0.000000000000000000 ) ) ;
#5214=EDGE_LOOP ( 'NONE', ( #20365, #13759, #26373, #1495 ) ) ;
#5218=FACE_OUTER_BOUND ( 'NONE', #2000, .T. ) ;
#5222=CARTESIAN_POINT ( 'NONE',  ( 7.244487271036906151, -74.17548517116718187, -40.28268501225647213 ) ) ;
#5223=CARTESIAN_POINT ( 'NONE',  ( -11.70222064965240172, -62.88295250684831927, 21.29956024434785533 ) ) ;
#5226=CARTESIAN_POINT ( 'NONE',  ( -1.921056761090000009, -65.40406720010000186, -25.43250850220000103 ) ) ;
#5227=CARTESIAN_POINT ( 'NONE',  ( -14.26173026869999916, -70.13572605659999226, 23.46380719780000135 ) ) ;
#5228=ORIENTED_EDGE ( 'NONE', *, *, #23622, .T. ) ;
#5231=CARTESIAN_POINT ( 'NONE',  ( 25.13837759289999951, -65.04696659260000047, -0.1122880703080000042 ) ) ;
#5232=CARTESIAN_POINT ( 'NONE',  ( 19.49031394080000013, -35.44486363859999756, -8.986483599810000555 ) ) ;
#5234=DIRECTION ( 'NONE',  ( 0.000000000000000000, -1.000000000000000000, 0.000000000000000000 ) ) ;
#5235=CIRCLE ( 'NONE', #10780, 3.000000000000000888 ) ;
#5236=CARTESIAN_POINT ( 'NONE',  ( -2.659303201050000176, -19.18187901349999791, -24.02256761569999810 ) ) ;
#5238=B_SPLINE_CURVE_WITH_KNOTS ( 'NONE', 3,
 ( #25080, #5115, #22902, #2941 ),
 .UNSPECIFIED., .F., .F.,
 ( 4, 4 ),
 ( 0.000000000000000000, 6.855861996820000748 ),
 .UNSPECIFIED. ) ;
#5239=ORIENTED_EDGE ( 'NONE', *, *, #3504, .T. ) ;
#5242=CARTESIAN_POINT ( 'NONE',  ( 22.19742911240000183, -63.93339545899999621, 11.06904267899999894 ) ) ;
#5243=CARTESIAN_POINT ( 'NONE',  ( 8.448066558069998067, -35.04931392889999842, -20.87699790789999810 ) ) ;
#5248=CARTESIAN_POINT ( 'NONE',  ( -12.30071345790000059, -60.59571585039999775, -20.16720244700000109 ) ) ;
#5251=ORIENTED_EDGE ( 'NONE', *, *, #14018, .T. ) ;
#5252=CARTESIAN_POINT ( 'NONE',  ( 46.73654926506065266, -73.84018091753036117, -2.679827245328084029 ) ) ;
#5253=ORIENTED_EDGE ( 'NONE', *, *, #21481, .F. ) ;
#5256=CARTESIAN_POINT ( 'NONE',  ( -10.80893812770000117, -34.66940579810000145, 19.80733931360000000 ) ) ;
#5258=VERTEX_POINT ( 'NONE', #16336 ) ;
#5259=CIRCLE ( 'NONE', #28501, 3.750000000000000000 ) ;
#5260=CARTESIAN_POINT ( 'NONE',  ( 45.99664576397077553, -80.06168502921590857, -4.396813276268206394 ) ) ;
#5262=CARTESIAN_POINT ( 'NONE',  ( -10.45725474138590982, -19.47453298910726716, -20.36980114618768312 ) ) ;
#5265=CARTESIAN_POINT ( 'NONE',  ( 10.08508256729999886, -64.24504434620000382, -24.78974309399999854 ) ) ;
#5267=DIRECTION ( 'NONE',  ( 0.000000000000000000, -1.000000000000000000, 0.000000000000000000 ) ) ;
#5272=CIRCLE ( 'NONE', #20645, 0.5000000000000027756 ) ;
#5273=FACE_OUTER_BOUND ( 'NONE', #563, .T. ) ;
#5275=DIRECTION ( 'NONE',  ( 0.7506477800816132584, 0.000000000000000000, -0.6607025883546591150 ) ) ;
#5279=CARTESIAN_POINT ( 'NONE',  ( -19.63703172620000004, -39.31812514049999407, 14.25736781099999995 ) ) ;
#5281=CARTESIAN_POINT ( 'NONE',  ( 27.75394116159999669, -74.50000000000000000, -27.75394116159999669 ) ) ;
#5283=CARTESIAN_POINT ( 'NONE',  ( 23.45077801099999704, -61.76643916500000131, -9.453800512080000829 ) ) ;
#5287=EDGE_CURVE ( 'NONE', #6525, #8106, #1966, .T. ) ;
#5289=CARTESIAN_POINT ( 'NONE',  ( -7.105427357599999217E-15, -84.50000000000000000, -3.552713678799999608E-15 ) ) ;
#5290=CARTESIAN_POINT ( 'NONE',  ( 1.598721155460000041E-15, -84.50000000000000000, 3.352873534370000046E-15 ) ) ;
#5291=CIRCLE ( 'NONE', #675, 3.500000000000003109 ) ;
#5292=CARTESIAN_POINT ( 'NONE',  ( 21.56903202939999886, -37.01027120230000378, -8.514697926349999335 ) ) ;
#5293=DIRECTION ( 'NONE',  ( 0.000000000000000000, -1.000000000000000000, 0.000000000000000000 ) ) ;
#5295=CARTESIAN_POINT ( 'NONE',  ( 21.32348952279355814, -36.24018116387741628, -9.136262763236869588 ) ) ;
#5299=CARTESIAN_POINT ( 'NONE',  ( 8.437044979949998691, -36.55186187079999627, -21.65894763279999680 ) ) ;
#5302=ORIENTED_EDGE ( 'NONE', *, *, #25396, .F. ) ;
#5307=CARTESIAN_POINT ( 'NONE',  ( -1.494460185578279088, -19.46625705891651847, -22.21735697087711969 ) ) ;
#5309=CARTESIAN_POINT ( 'NONE',  ( 26.46310988749999993, -64.24504445130001784, 1.532420830840000026 ) ) ;
#5312=CARTESIAN_POINT ( 'NONE',  ( -38.90587669217570976, -73.50000000000002842, 7.169550435234046226 ) ) ;
#5314=CARTESIAN_POINT ( 'NONE',  ( 21.65894763289999858, -36.55186186859999964, -8.437044980280001383 ) ) ;
#5317=VERTEX_POINT ( 'NONE', #4838 ) ;
#5319=B_SPLINE_CURVE_WITH_KNOTS ( 'NONE', 3,
 ( #1199, #9762, #10034, #8010, #18818, #27707, #5407, #7746, #16612, #16900, #1735, #13221, #4048, #21979 ),
 .UNSPECIFIED., .F., .F.,
 ( 4, 2, 2, 1, 1, 2, 2, 4 ),
 ( 0.000000000000000000, 0.2500000000000178746, 0.3750000000000266454, 0.4375000000000310307, 0.4687500000000333067, 0.4843750000000344169, 0.5000000000000355271, 1.000000000000000000 ),
 .UNSPECIFIED. ) ;
#5320=B_SPLINE_CURVE_WITH_KNOTS ( 'NONE', 3,
 ( #3218, #22895, #27404, #16465, #12079, #24780, #2933, #25225, #22743, #22599, #18512, #18070, #7005, #4819, #13697, #20552, #5252, #20707, #7999, #3765, #23864, #1315, #8135, #14418, #10025, #10157, #12484, #14818, #18806, #12626, #19077 ),
 .UNSPECIFIED., .F., .F.,
 ( 4, 2, 1, 1, 1, 2, 2, 2, 1, 1, 1, 2, 2, 2, 1, 1, 1, 2, 2, 4 ),
 ( 0.000000000000000000, 0.1250000000000331124, 0.1875000000000519307, 0.2187500000000589251, 0.2343750000000601463, 0.2421875000000630329, 0.2500000000000659472, 0.3750000000000856537, 0.4375000000000947020, 0.4687500000000999756, 0.4843750000001043055, 0.4921875000001044720, 0.5000000000001045830, 0.6250000000000885958, 0.6875000000000806022, 0.7187500000000779377, 0.7343750000000768274, 0.7421875000000747180, 0.7500000000000724976, 1.000000000000000000 ),
 .UNSPECIFIED. ) ;
#5322=CARTESIAN_POINT ( 'NONE',  ( 47.19280574540000117, -74.66665734379999719, -1.149945984370000174 ) ) ;
#5325=CARTESIAN_POINT ( 'NONE',  ( -2.664535259099999805E-15, -72.00000000000000000, -3.552713678799999608E-15 ) ) ;
#5326=FACE_OUTER_BOUND ( 'NONE', #12299, .T. ) ;
#5327=CARTESIAN_POINT ( 'NONE',  ( 10.20110288159999890, -84.00000000000000000, 41.00000000000000000 ) ) ;
#5328=DIRECTION ( 'NONE',  ( 0.000000000000000000, -1.000000000000000000, 0.000000000000000000 ) ) ;
#5330=VECTOR ( 'NONE', #23160, 1000.000000000000000 ) ;
#5332=EDGE_LOOP ( 'NONE', ( #2430, #7969, #4855, #7432 ) ) ;
#5333=AXIS2_PLACEMENT_3D ( 'NONE', #18484, #28557, #10757 ) ;
#5339=CARTESIAN_POINT ( 'NONE',  ( -7.185776204499999764, -73.64071409359999620, 38.99606912750000731 ) ) ;
#5341=CARTESIAN_POINT ( 'NONE',  ( 25.07535757159999790, -74.22136841340000046, -30.21433045149999685 ) ) ;
#5342=CARTESIAN_POINT ( 'NONE',  ( 9.226669613569999484, -71.28738307410000630, -26.41756239489999913 ) ) ;
#5343=CARTESIAN_POINT ( 'NONE',  ( -13.46604720019999846, -19.89614183979999851, 20.40796202710000173 ) ) ;
#5345=DIRECTION ( 'NONE',  ( 0.000000000000000000, -1.000000000000000000, 0.000000000000000000 ) ) ;
#5348=CARTESIAN_POINT ( 'NONE',  ( 10.33697414329999908, -72.00000000000000000, -28.69893982729999848 ) ) ;
#5349=DIRECTION ( 'NONE',  ( 0.9842024174352067556, 0.000000000000000000, -0.1770468907230369482 ) ) ;
#5350=VERTEX_POINT ( 'NONE', #9487 ) ;
#5352=DIRECTION ( 'NONE',  ( 1.000000000000000000, 0.000000000000000000, 0.000000000000000000 ) ) ;
#5355=ORIENTED_EDGE ( 'NONE', *, *, #1193, .F. ) ;
#5356=EDGE_CURVE ( 'NONE', #11676, #25229, #27895, .T. ) ;
#5357=CARTESIAN_POINT ( 'NONE',  ( -0.8483992499709999136, -57.91738531389999878, -23.36308592830000208 ) ) ;
#5363=CARTESIAN_POINT ( 'NONE',  ( 22.03428119550000019, -37.34495693419999185, -8.933655458900000568 ) ) ;
#5364=CARTESIAN_POINT ( 'NONE',  ( 46.96755458150000351, -74.27975760209999123, -2.596029696810000065 ) ) ;
#5371=CARTESIAN_POINT ( 'NONE',  ( -3.243670240720000209, -70.36214388629998950, -27.70857142859999911 ) ) ;
#5372=CARTESIAN_POINT ( 'NONE',  ( -14.93352430010000020, -69.88459027950000291, 23.05437816310000088 ) ) ;
#5373=ORIENTED_EDGE ( 'NONE', *, *, #861, .T. ) ;
#5374=CARTESIAN_POINT ( 'NONE',  ( -14.65665288169999947, -79.50000000000000000, 36.94583914790000279 ) ) ;
#5375=B_SPLINE_CURVE_WITH_KNOTS ( 'NONE', 5,
 ( #982, #22966, #18733, #19008, #16536, #16232, #5462, #7931, #27327 ),
 .UNSPECIFIED., .F., .F.,
 ( 6, 3, 6 ),
 ( 0.000000000000000000, 0.4480559759399665998, 1.000000000000000000 ),
 .UNSPECIFIED. ) ;
#5377=CARTESIAN_POINT ( 'NONE',  ( 24.46716655439999855, -58.91551295370000219, 1.187497063919999984 ) ) ;
#5378=CARTESIAN_POINT ( 'NONE',  ( 19.49373789020000203, -35.48172793740000230, -8.986332944369998188 ) ) ;
#5379=ORIENTED_EDGE ( 'NONE', *, *, #3347, .T. ) ;
#5380=DIRECTION ( 'NONE',  ( 0.000000000000000000, 1.000000000000000000, 0.000000000000000000 ) ) ;
#5381=CARTESIAN_POINT ( 'NONE',  ( -2.776065240120000333, -18.86697026210000061, -23.72009294809999957 ) ) ;
#5383=VERTEX_POINT ( 'NONE', #13860 ) ;
#5384=CARTESIAN_POINT ( 'NONE',  ( -10.13149966729999818, -18.50000000000000000, 18.43352823549999897 ) ) ;
#5387=CARTESIAN_POINT ( 'NONE',  ( 22.43277176080000146, -36.00000000000000000, -11.31764183710000005 ) ) ;
#5389=CARTESIAN_POINT ( 'NONE',  ( -3.967099564274365164, -72.37489743483658344, -28.45199697807708006 ) ) ;
#5390=VERTEX_POINT ( 'NONE', #20573 ) ;
#5392=CARTESIAN_POINT ( 'NONE',  ( -12.45432576839999861, -65.00127508749999095, -21.87307312520000124 ) ) ;
#5393=CARTESIAN_POINT ( 'NONE',  ( 24.54494471330000138, -66.27261548020000248, -9.685072589820000744 ) ) ;
#5394=DIRECTION ( 'NONE',  ( 0.000000000000000000, 1.000000000000000000, 0.000000000000000000 ) ) ;
#5396=FACE_OUTER_BOUND ( 'NONE', #16286, .T. ) ;
#5403=ORIENTED_EDGE ( 'NONE', *, *, #21864, .T. ) ;
#5407=CARTESIAN_POINT ( 'NONE',  ( -11.65705697597267942, -61.40679450237151826, -22.99730055226696734 ) ) ;
#5408=CARTESIAN_POINT ( 'NONE',  ( 47.19132921107751599, -79.33749027171297996, -1.164644976861414438 ) ) ;
#5413=VERTEX_POINT ( 'NONE', #5048 ) ;
#5417=ORIENTED_EDGE ( 'NONE', *, *, #17999, .F. ) ;
#5418=DIRECTION ( 'NONE',  ( 0.09756097560976716154, 0.000000000000000000, -0.9952295494196655712 ) ) ;
#5419=CARTESIAN_POINT ( 'NONE',  ( -19.24779671730000175, -32.69575302480000545, 13.93068917299999931 ) ) ;
#5422=CARTESIAN_POINT ( 'NONE',  ( 22.18796890659999832, -59.03423364030000187, -7.691677767369998975 ) ) ;
#5423=B_SPLINE_CURVE_WITH_KNOTS ( 'NONE', 3,
 ( #25467, #16859, #9996, #23557, #5498, #3323, #12454, #28071 ),
 .UNSPECIFIED., .F., .F.,
 ( 4, 2, 2, 4 ),
 ( 0.000000000000000000, 0.5000000000000066613, 0.7500000000000033307, 1.000000000000000000 ),
 .UNSPECIFIED. ) ;
#5424=VERTEX_POINT ( 'NONE', #24872 ) ;
#5426=CARTESIAN_POINT ( 'NONE',  ( 8.681080848429999719, -37.64807918700000045, -21.92361636220000065 ) ) ;
#5427=CARTESIAN_POINT ( 'NONE',  ( -19.73459501710000197, -19.50000000000000000, 14.41863426819999994 ) ) ;
#5428=CARTESIAN_POINT ( 'NONE',  ( 21.61801161090000178, -37.04357994280000099, -8.573564459640000024 ) ) ;
#5430=VERTEX_POINT ( 'NONE', #17877 ) ;
#5431=DIRECTION ( 'NONE',  ( 0.000000000000000000, 1.000000000000000000, 0.000000000000000000 ) ) ;
#5438=VERTEX_POINT ( 'NONE', #25013 ) ;
#5441=CARTESIAN_POINT ( 'NONE',  ( -40.65853658540000026, -84.00000000000000000, -6.717799458580000049 ) ) ;
#5442=CARTESIAN_POINT ( 'NONE',  ( -13.15600360629633236, -19.48875933375592950, 19.82831268508771316 ) ) ;
#5445=B_SPLINE_CURVE_WITH_KNOTS ( 'NONE', 3,
 ( #6102, #1895, #10455, #3926 ),
 .UNSPECIFIED., .F., .F.,
 ( 4, 4 ),
 ( -4.007730545210000273, -3.491867373409999864 ),
 .UNSPECIFIED. ) ;
#5446=CARTESIAN_POINT ( 'NONE',  ( 19.69582338720000081, -18.50000000000000000, -7.383548592259999488 ) ) ;
#5447=ADVANCED_FACE ( 'NONE', ( #28781 ), #472, .T. ) ;
#5449=CARTESIAN_POINT ( 'NONE',  ( -2.604257624009999716, -32.67314203990000010, -24.29262257289999738 ) ) ;
#5451=EDGE_CURVE ( 'NONE', #3863, #5430, #15291, .T. ) ;
#5452=CARTESIAN_POINT ( 'NONE',  ( -31.89935321680000158, -74.00000000000000000, -21.99985828019999801 ) ) ;
#5454=CARTESIAN_POINT ( 'NONE',  ( 22.59227796120000065, -53.25913232239999928, -9.063833271410000947 ) ) ;
#5456=CARTESIAN_POINT ( 'NONE',  ( 36.24656966590000451, -75.00000018780001199, -15.05817676390000059 ) ) ;
#5457=ORIENTED_EDGE ( 'NONE', *, *, #11788, .T. ) ;
#5460=DIRECTION ( 'NONE',  ( 1.000000000000000000, 0.000000000000000000, 0.000000000000000000 ) ) ;
#5461=CARTESIAN_POINT ( 'NONE',  ( 21.34788071859999903, -35.28814083279999636, -7.426814964410000108 ) ) ;
#5462=CARTESIAN_POINT ( 'NONE',  ( 36.27185351749999853, -79.54415414250000538, -14.99731109350000047 ) ) ;
#5464=DIRECTION ( 'NONE',  ( 1.000000000000000000, 0.000000000000000000, 0.000000000000000000 ) ) ;
#5465=CARTESIAN_POINT ( 'NONE',  ( -11.35954001540000036, -79.50000000000000000, 47.25000000000000000 ) ) ;
#5470=LINE ( 'NONE', #7806, #27115 ) ;
#5472=ADVANCED_FACE ( 'NONE', ( #14374 ), #5621, .F. ) ;
#5478=EDGE_CURVE ( 'NONE', #7089, #22756, #20453, .T. ) ;
#5480=CARTESIAN_POINT ( 'NONE',  ( 20.30102379280000235, -72.31415926540000783, -30.97095677779999789 ) ) ;
#5482=CARTESIAN_POINT ( 'NONE',  ( -21.23294764439999938, -65.91137168669999369, 14.52552031449999959 ) ) ;
#5487=CYLINDRICAL_SURFACE ( 'NONE', #8091, 3.749999999999996447 ) ;
#5488=VERTEX_POINT ( 'NONE', #12025 ) ;
#5490=ORIENTED_EDGE ( 'NONE', *, *, #10658, .T. ) ;
#5491=CARTESIAN_POINT ( 'NONE',  ( -14.03261327740279896, -80.23900667062660830, 36.71350245345666252 ) ) ;
#5494=DIRECTION ( 'NONE',  ( -0.2414462220490755373, 0.000000000000000000, 0.9704142011833032377 ) ) ;
#5495=ORIENTED_EDGE ( 'NONE', *, *, #8218, .T. ) ;
#5496=CARTESIAN_POINT ( 'NONE',  ( -7.370698677632464779, -73.94611354405870429, 38.67409461690933625 ) ) ;
#5497=ADVANCED_FACE ( 'NONE', ( #25169 ), #25731, .F. ) ;
#5498=CARTESIAN_POINT ( 'NONE',  ( -7.479537002312467209, -74.09468416707295546, -39.31219897218396397 ) ) ;
#5499=EDGE_LOOP ( 'NONE', ( #27834, #25020, #13822, #17521 ) ) ;
#5500=CARTESIAN_POINT ( 'NONE',  ( 7.448284947614243201, -36.87977280728636487, -21.48523428999794760 ) ) ;
#5501=CARTESIAN_POINT ( 'NONE',  ( -11.91368332737741831, -63.90944102351340916, 21.57903816910991779 ) ) ;
#5502=EDGE_CURVE ( 'NONE', #15872, #14143, #23983, .T. ) ;
#5504=CARTESIAN_POINT ( 'NONE',  ( -14.54237663339999997, -79.81382879129999708, 36.82469782859999441 ) ) ;
#5505=VECTOR ( 'NONE', #23737, 1000.000000000000114 ) ;
#5506=CARTESIAN_POINT ( 'NONE',  ( -3.778287650309999801, -69.97113394379999818, -28.14671785339999843 ) ) ;
#5507=CARTESIAN_POINT ( 'NONE',  ( -13.83569956370000043, -69.21570870340001136, 23.22967513160000053 ) ) ;
#5508=EDGE_LOOP ( 'NONE', ( #6566, #8171, #19223 ) ) ;
#5510=DIRECTION ( 'NONE',  ( 0.000000000000000000, 1.000000000000000000, 0.000000000000000000 ) ) ;
#5512=CARTESIAN_POINT ( 'NONE',  ( 26.01008226429999937, -64.47176828549999072, 1.369137345940000028 ) ) ;
#5513=CARTESIAN_POINT ( 'NONE',  ( -21.14183719079999690, -62.95300605010000083, 15.28077941859999989 ) ) ;
#5514=ORIENTED_EDGE ( 'NONE', *, *, #21807, .F. ) ;
#5516=CARTESIAN_POINT ( 'NONE',  ( -0.5268693940142937793, -39.36577620583297943, -22.72254148439001398 ) ) ;
#5517=CARTESIAN_POINT ( 'NONE',  ( -7.282285323108220965, -73.99998672515624776, 39.66612828077759900 ) ) ;
#5518=CARTESIAN_POINT ( 'NONE',  ( 36.38049338981862491, -74.01943097537444771, -13.95685178916381730 ) ) ;
#5519=ORIENTED_EDGE ( 'NONE', *, *, #21645, .F. ) ;
#5520=LINE ( 'NONE', #21254, #20990 ) ;
#5522=CARTESIAN_POINT ( 'NONE',  ( 36.43808797039999803, -79.65546220359999552, -14.69303470340000040 ) ) ;
#5523=CARTESIAN_POINT ( 'NONE',  ( 36.70830927769999619, -74.93175448689999030, -14.75000110549999910 ) ) ;
#5526=CARTESIAN_POINT ( 'NONE',  ( -40.00000000000000000, -69.00000000000000000, 3.236300116779999679E-15 ) ) ;
#5527=VERTEX_POINT ( 'NONE', #3171 ) ;
#5528=CARTESIAN_POINT ( 'NONE',  ( -14.93121066289999987, -74.50000000000000000, 36.29905574720000061 ) ) ;
#5530=ORIENTED_EDGE ( 'NONE', *, *, #6133, .T. ) ;
#5531=CARTESIAN_POINT ( 'NONE',  ( -11.00251064340000084, -27.06784995459999976, 19.39886944670000091 ) ) ;
#5534=CARTESIAN_POINT ( 'NONE',  ( -2.580132123360000307, -54.50138674060000454, -25.16134040389999882 ) ) ;
#5536=EDGE_CURVE ( 'NONE', #22592, #3729, #4006, .T. ) ;
#5539=CARTESIAN_POINT ( 'NONE',  ( 39.03038279099999386, -74.00032110540000474, 7.562806955190000124 ) ) ;
#5541=ADVANCED_FACE ( 'NONE', ( #18756 ), #21220, .F. ) ;
#5546=AXIS2_PLACEMENT_3D ( 'NONE', #10523, #12578, #21350 ) ;
#5547=CARTESIAN_POINT ( 'NONE',  ( -32.68889462130000112, -80.00000031659999422, -22.56856178450000172 ) ) ;
#5548=CARTESIAN_POINT ( 'NONE',  ( 10.08508256729999886, -64.24504434620000382, -24.78974309399999854 ) ) ;
#5549=CIRCLE ( 'NONE', #6945, 3.499999999999999556 ) ;
#5551=CARTESIAN_POINT ( 'NONE',  ( -34.11790219230000076, -79.50000000000000000, -24.21840725559999896 ) ) ;
#5552=ORIENTED_EDGE ( 'NONE', *, *, #13996, .T. ) ;
#5553=CIRCLE ( 'NONE', #7408, 0.4999999999999982236 ) ;
#5555=VERTEX_POINT ( 'NONE', #9565 ) ;
#5556=FACE_OUTER_BOUND ( 'NONE', #3180, .T. ) ;
#5561=ADVANCED_FACE ( 'NONE', ( #25455 ), #23265, .F. ) ;
#5562=DIRECTION ( 'NONE',  ( 0.000000000000000000, 0.000000000000000000, 1.000000000000000000 ) ) ;
#5563=CARTESIAN_POINT ( 'NONE',  ( -10.90352314479999940, -18.50000000000000000, 18.09320272940000152 ) ) ;
#5565=CIRCLE ( 'NONE', #9272, 6.750000000000002665 ) ;
#5568=DIRECTION ( 'NONE',  ( 1.000000000000000000, 0.000000000000000000, 0.000000000000000000 ) ) ;
#5569=CARTESIAN_POINT ( 'NONE',  ( 20.10924407270000103, -35.62996179179999245, -8.973978175680001002 ) ) ;
#5571=ORIENTED_EDGE ( 'NONE', *, *, #17538, .F. ) ;
#5574=CARTESIAN_POINT ( 'NONE',  ( -16.01759400379999931, -69.30633957129998635, 23.18138418170000037 ) ) ;
#5576=CARTESIAN_POINT ( 'NONE',  ( 40.00000000000000000, -82.25000000000000000, 0.000000000000000000 ) ) ;
#5583=ORIENTED_EDGE ( 'NONE', *, *, #19697, .T. ) ;
#5584=CARTESIAN_POINT ( 'NONE',  ( 19.82501711970000002, -19.48264111129999776, -8.815784396710000692 ) ) ;
#5588=AXIS2_PLACEMENT_3D ( 'NONE', #13392, #6714, #22452 ) ;
#5592=CARTESIAN_POINT ( 'NONE',  ( 8.985156090609999424, -35.55399656489999671, -19.52064371570000034 ) ) ;
#5593=CARTESIAN_POINT ( 'NONE',  ( 22.62696043789999933, -36.51121532250000001, -9.295214654749999639 ) ) ;
#5595=CARTESIAN_POINT ( 'NONE',  ( -10.60846119319999836, -27.03158754559999721, -21.08535220339999938 ) ) ;
#5597=EDGE_CURVE ( 'NONE', #26341, #26269, #8647, .T. ) ;
#5598=CARTESIAN_POINT ( 'NONE',  ( -32.72710940640000388, -74.40224539360001188, -22.12820698629999683 ) ) ;
#5601=CARTESIAN_POINT ( 'NONE',  ( 8.973973756419999503, -35.62994960090000518, -20.10924160899999791 ) ) ;
#5604=CARTESIAN_POINT ( 'NONE',  ( 7.105427357599999217E-15, -74.50000000000000000, 3.552713678799999608E-15 ) ) ;
#5605=TOROIDAL_SURFACE ( 'NONE', #18166, 38.75000000000000000, 0.5000000000000000000 ) ;
#5608=ORIENTED_EDGE ( 'NONE', *, *, #24373, .F. ) ;
#5610=CARTESIAN_POINT ( 'NONE',  ( -12.17175180279999935, -57.47855601759999900, -19.93971687999999887 ) ) ;
#5616=CARTESIAN_POINT ( 'NONE',  ( 25.16314806569999973, -73.44383031769999093, -29.90446131310000055 ) ) ;
#5619=DIRECTION ( 'NONE',  ( 1.000000000000000000, 0.000000000000000000, 0.000000000000000000 ) ) ;
#5620=CARTESIAN_POINT ( 'NONE',  ( 8.528659902539999393, -19.44973803559999936, -20.19953053829999945 ) ) ;
#5621=CYLINDRICAL_SURFACE ( 'NONE', #6962, 0.5000000000000025535 ) ;
#5624=ORIENTED_EDGE ( 'NONE', *, *, #15617, .T. ) ;
#5631=CARTESIAN_POINT ( 'NONE',  ( -14.19188855770000046, -80.00000000000000000, 37.13021410070000883 ) ) ;
#5632=EDGE_CURVE ( 'NONE', #28507, #24612, #6327, .T. ) ;
#5636=VERTEX_POINT ( 'NONE', #8645 ) ;
#5637=DIRECTION ( 'NONE',  ( 0.000000000000000000, -1.000000000000000000, 0.000000000000000000 ) ) ;
#5638=DIRECTION ( 'NONE',  ( 0.000000000000000000, 1.000000000000000000, 0.000000000000000000 ) ) ;
#5639=ORIENTED_EDGE ( 'NONE', *, *, #1141, .T. ) ;
#5641=CARTESIAN_POINT ( 'NONE',  ( 8.034824971200507093, -66.63181019764634527, -24.57972119927973154 ) ) ;
#5642=CARTESIAN_POINT ( 'NONE',  ( 7.461111551219999249, -36.92670964950000467, -21.48614944720000253 ) ) ;
#5644=CARTESIAN_POINT ( 'NONE',  ( 21.98941332900000134, -49.11505549560000361, -6.974892859150000568 ) ) ;
#5646=CARTESIAN_POINT ( 'NONE',  ( -22.10465418478271005, -74.05401792490640389, -32.32543926652451916 ) ) ;
#5647=ORIENTED_EDGE ( 'NONE', *, *, #21146, .F. ) ;
#5651=CARTESIAN_POINT ( 'NONE',  ( 19.49202744680000166, -35.46335013489999710, -8.986408038590001368 ) ) ;
#5655=CARTESIAN_POINT ( 'NONE',  ( -3.024786108369999837, -18.62181730670000235, -23.68429331439999785 ) ) ;
#5656=CARTESIAN_POINT ( 'NONE',  ( 36.74383121569999844, -74.66666669110000498, -14.69280905019999928 ) ) ;
#5658=CARTESIAN_POINT ( 'NONE',  ( 36.24656994149999889, -79.00000000000000000, -15.05817610060000078 ) ) ;
#5661=AXIS2_PLACEMENT_3D ( 'NONE', #12240, #21154, #9772 ) ;
#5666=CARTESIAN_POINT ( 'NONE',  ( -2.682509845957436134, -80.39326405337963877, 46.73547856321033578 ) ) ;
#5668=VERTEX_POINT ( 'NONE', #9084 ) ;
#5670=ORIENTED_EDGE ( 'NONE', *, *, #16717, .F. ) ;
#5675=CARTESIAN_POINT ( 'NONE',  ( -17.94180966909999597, -19.50000000000000000, 18.81731824139999887 ) ) ;
#5680=CARTESIAN_POINT ( 'NONE',  ( 46.55834487451462422, -79.96456861975623553, -3.902750372498239084 ) ) ;
#5681=VERTEX_POINT ( 'NONE', #13756 ) ;
#5686=CARTESIAN_POINT ( 'NONE',  ( -1.986940095230000036, -55.03616289790000593, -23.76239100950000349 ) ) ;
#5687=CARTESIAN_POINT ( 'NONE',  ( -3.562216359109999786, -80.34292033629999708, 46.31451622120000167 ) ) ;
#5689=VERTEX_POINT ( 'NONE', #19864 ) ;
#5692=CARTESIAN_POINT ( 'NONE',  ( 27.75394116159999669, -74.50000000000000000, -27.75394116159999669 ) ) ;
#5695=ADVANCED_FACE ( 'NONE', ( #15334 ), #4725, .T. ) ;
#5698=DIRECTION ( 'NONE',  ( 0.000000000000000000, -1.000000000000000000, 0.000000000000000000 ) ) ;
#5700=AXIS2_PLACEMENT_3D ( 'NONE', #948, #23344, #8232 ) ;
#5702=CARTESIAN_POINT ( 'NONE',  ( -39.97648509736585964, -73.96150430845531787, -7.250349464191292448 ) ) ;
#5704=ORIENTED_EDGE ( 'NONE', *, *, #28715, .F. ) ;
#5707=CARTESIAN_POINT ( 'NONE',  ( -16.72250540970000188, -71.11599492770000097, 23.42677820880000183 ) ) ;
#5710=CARTESIAN_POINT ( 'NONE',  ( 37.60355029590000697, -84.00000000000000000, -9.356041104380000917 ) ) ;
#5713=CARTESIAN_POINT ( 'NONE',  ( -40.29089741864007834, -74.18137224046458300, 7.244162156032251332 ) ) ;
#5714=EDGE_CURVE ( 'NONE', #4093, #20809, #17986, .T. ) ;
#5715=CARTESIAN_POINT ( 'NONE',  ( 46.75000000000000000, -69.50000000000000000, 7.285566699530000990E-15 ) ) ;
#5718=CARTESIAN_POINT ( 'NONE',  ( 20.46648349389999666, -19.16110312220000012, -8.147944065169999917 ) ) ;
#5721=CIRCLE ( 'NONE', #3848, 3.500000000000003109 ) ;
#5722=CARTESIAN_POINT ( 'NONE',  ( -14.64093407760000076, -74.15747494800001505, 36.27438844899999992 ) ) ;
#5724=CARTESIAN_POINT ( 'NONE',  ( 10.20110288159999890, -84.50000000000000000, -41.00000000000000000 ) ) ;
#5725=VERTEX_POINT ( 'NONE', #18282 ) ;
#5727=DIRECTION ( 'NONE',  ( 0.000000000000000000, 1.000000000000000000, 0.000000000000000000 ) ) ;
#5728=CARTESIAN_POINT ( 'NONE',  ( 22.16162922080000186, -57.47158989559999753, -7.992697997670000554 ) ) ;
#5730=CARTESIAN_POINT ( 'NONE',  ( 6.846103682120000755, -36.12241484350000320, -21.55427193710000111 ) ) ;
#5731=LINE ( 'NONE', #28292, #20142 ) ;
#5737=AXIS2_PLACEMENT_3D ( 'NONE', #15960, #22830, #18456 ) ;
#5740=CARTESIAN_POINT ( 'NONE',  ( 8.770435879989999961, -35.38531427019999853, -20.52569411800000054 ) ) ;
#5741=CARTESIAN_POINT ( 'NONE',  ( 7.219194746714282296, -73.62392792451103674, 39.33235237968798259 ) ) ;
#5744=AXIS2_PLACEMENT_3D ( 'NONE', #11650, #20560, #330 ) ;
#5748=ORIENTED_EDGE ( 'NONE', *, *, #19002, .F. ) ;
#5749=CARTESIAN_POINT ( 'NONE',  ( -1.314504061159999897E-13, -19.46510050329999686, -1.119104808819999722E-13 ) ) ;
#5750=ORIENTED_EDGE ( 'NONE', *, *, #12855, .T. ) ;
#5752=ADVANCED_FACE ( 'NONE', ( #14048 ), #4507, .T. ) ;
#5756=CARTESIAN_POINT ( 'NONE',  ( 40.00000000000000000, -73.00000000000000000, 2.433892081919999696E-15 ) ) ;
#5757=CARTESIAN_POINT ( 'NONE',  ( 25.11727467239999712, -73.66811105200000043, -29.97254555069999782 ) ) ;
#5758=CARTESIAN_POINT ( 'NONE',  ( -22.07768936720000141, -67.34374581909999335, 16.43776412940000142 ) ) ;
#5760=CARTESIAN_POINT ( 'NONE',  ( -18.49356544879450581, -19.46625705890763669, 12.40291896993568699 ) ) ;
#5763=DIRECTION ( 'NONE',  ( 1.836909530730000976E-16, 0.000000000000000000, -1.000000000000000000 ) ) ;
#5764=ORIENTED_EDGE ( 'NONE', *, *, #7429, .F. ) ;
#5765=CARTESIAN_POINT ( 'NONE',  ( -10.94986905363052543, -44.38603308081882659, 20.11695812405464068 ) ) ;
#5767=AXIS2_PLACEMENT_3D ( 'NONE', #28250, #15113, #19646 ) ;
#5768=CARTESIAN_POINT ( 'NONE',  ( -0.5578430832430000263, -60.34941021230000047, -23.62008496760000043 ) ) ;
#5769=CIRCLE ( 'NONE', #25328, 38.75000000000000000 ) ;
#5772=ORIENTED_EDGE ( 'NONE', *, *, #1133, .F. ) ;
#5773=CARTESIAN_POINT ( 'NONE',  ( -15.00047198269999882, -74.50000000000000000, 39.16845525979999820 ) ) ;
#5774=ORIENTED_EDGE ( 'NONE', *, *, #18225, .F. ) ;
#5777=CARTESIAN_POINT ( 'NONE',  ( 7.532037665939999904, -37.10289230739999766, -21.49296857539999905 ) ) ;
#5781=CARTESIAN_POINT ( 'NONE',  ( -17.73582829829999952, -18.50000000000000000, 11.34636642620000124 ) ) ;
#5783=EDGE_CURVE ( 'NONE', #28456, #17366, #23644, .T. ) ;
#5786=CARTESIAN_POINT ( 'NONE',  ( 23.55258138210000141, -57.47122622279999860, 0.3294346322440000474 ) ) ;
#5787=CARTESIAN_POINT ( 'NONE',  ( -20.88233480739999948, -63.63883271309998690, 12.80551527529999944 ) ) ;
#5788=ORIENTED_EDGE ( 'NONE', *, *, #12658, .T. ) ;
#5789=AXIS2_PLACEMENT_3D ( 'NONE', #15072, #8809, #21656 ) ;
#5793=CARTESIAN_POINT ( 'NONE',  ( -1.415652922210000053, -19.46458168450000059, -22.11082617310000131 ) ) ;
#5795=ORIENTED_EDGE ( 'NONE', *, *, #10051, .F. ) ;
#5796=ADVANCED_FACE ( 'NONE', ( #12827 ), #15168, .F. ) ;
#5798=CARTESIAN_POINT ( 'NONE',  ( 8.987275428499998498, -35.25070440529999871, -19.47217453680000077 ) ) ;
#5799=CARTESIAN_POINT ( 'NONE',  ( 36.36887067909999871, -79.22577739489999260, -14.85406736540000061 ) ) ;
#5800=ORIENTED_EDGE ( 'NONE', *, *, #3428, .F. ) ;
#5802=AXIS2_PLACEMENT_3D ( 'NONE', #22120, #22256, #28369 ) ;
#5806=CARTESIAN_POINT ( 'NONE',  ( -13.16183723299999997, -70.12921532840000793, -24.09258145020000086 ) ) ;
#5809=AXIS2_PLACEMENT_3D ( 'NONE', #19269, #10079, #3277 ) ;
#5811=CARTESIAN_POINT ( 'NONE',  ( 8.548167153169895727, -18.60777319252632012, -18.90116954123247339 ) ) ;
#5812=EDGE_LOOP ( 'NONE', ( #12174, #24678, #22629, #4073, #25026 ) ) ;
#5814=CARTESIAN_POINT ( 'NONE',  ( 19.49544348199999888, -35.50000000000000000, -8.986258402430001624 ) ) ;
#5815=ORIENTED_EDGE ( 'NONE', *, *, #9011, .F. ) ;
#5817=DIRECTION ( 'NONE',  ( 0.7071067811865475727, 0.000000000000000000, -0.7071067811865475727 ) ) ;
#5818=DIRECTION ( 'NONE',  ( -0.5301416321220548955, 0.000000000000000000, -0.8479091047340887588 ) ) ;
#5819=CARTESIAN_POINT ( 'NONE',  ( -1.558004792230000213, -18.50000000000000000, -21.15181860990000118 ) ) ;
#5828=CARTESIAN_POINT ( 'NONE',  ( -2.582000063019999736, -32.72519969599999712, -24.62603268980000237 ) ) ;
#5831=DIRECTION ( 'NONE',  ( 0.9952295494196653491, 0.000000000000000000, 0.09756097560976997873 ) ) ;
#5832=B_SPLINE_CURVE_WITH_KNOTS ( 'NONE', 5,
 ( #23300, #7854, #16456, #5389, #3209, #756 ),
 .UNSPECIFIED., .F., .F.,
 ( 6, 6 ),
 ( 0.000000000000000000, 1.000000000000000000 ),
 .UNSPECIFIED. ) ;
#5835=CARTESIAN_POINT ( 'NONE',  ( 28.96803677850000369, -74.08474241140000061, -26.54391550880000139 ) ) ;
#5836=CARTESIAN_POINT ( 'NONE',  ( -14.17623297788752801, -74.02548642939331103, 36.23315183394973360 ) ) ;
#5837=EDGE_LOOP ( 'NONE', ( #13485, #24196, #13283, #9790 ) ) ;
#5839=CARTESIAN_POINT ( 'NONE',  ( 20.55825494609999993, -36.03428657229999743, -8.976966250369997624 ) ) ;
#5840=CARTESIAN_POINT ( 'NONE',  ( -22.03951503178797466, -79.50000008679997165, -32.70331798545759483 ) ) ;
#5841=ORIENTED_EDGE ( 'NONE', *, *, #16811, .T. ) ;
#5846=CARTESIAN_POINT ( 'NONE',  ( 21.21808891099999883, -34.59820414320000026, -7.670974023059999425 ) ) ;
#5849=ORIENTED_EDGE ( 'NONE', *, *, #3428, .T. ) ;
#5850=EDGE_CURVE ( 'NONE', #10833, #8141, #21235, .T. ) ;
#5853=CARTESIAN_POINT ( 'NONE',  ( 27.11492820700000195, -72.00000000000000000, 10.50528228810000009 ) ) ;
#5854=CARTESIAN_POINT ( 'NONE',  ( 38.81101221950712699, -73.50000015768026174, 7.152485405691547449 ) ) ;
#5856=CARTESIAN_POINT ( 'NONE',  ( 47.20527375670212678, -74.60741763389601999, -0.8389613764862925427 ) ) ;
#5857=CARTESIAN_POINT ( 'NONE',  ( -14.86256651179999899, -74.31496036839999419, 36.29330022180000270 ) ) ;
#5858=CARTESIAN_POINT ( 'NONE',  ( -2.667359241160000227, -19.40610837490000051, -23.95394751019999902 ) ) ;
#5861=EDGE_CURVE ( 'NONE', #5636, #26524, #14685, .T. ) ;
#5862=DIRECTION ( 'NONE',  ( 1.000000000000000000, 0.000000000000000000, 0.000000000000000000 ) ) ;
#5864=CARTESIAN_POINT ( 'NONE',  ( 8.904050045449999118, -63.43030842769999111, -23.33241554479999991 ) ) ;
#5866=CARTESIAN_POINT ( 'NONE',  ( 21.09816162019999908, -57.90606206700000058, 10.50668310290000029 ) ) ;
#5868=ORIENTED_EDGE ( 'NONE', *, *, #15849, .F. ) ;
#5871=CARTESIAN_POINT ( 'NONE',  ( -32.77174708219999388, -74.50000000000000000, -21.60034937629999874 ) ) ;
#5875=CYLINDRICAL_SURFACE ( 'NONE', #22712, 32.39999999999999858 ) ;
#5877=B_SPLINE_CURVE_WITH_KNOTS ( 'NONE', 3,
 ( #24684, #11547, #9075, #6910, #27310, #4716, #2987, #524, #9371, #18273, #27166, #11849, #11399, #7351, #16369, #27459, #20760, #818, #14042, #16214, #27019, #9660, #13749, #9521, #22796, #18567, #7204, #25279, #4868, #5307, #2836, #14195, #7061, #23089 ),
 .UNSPECIFIED., .F., .F.,
 ( 4, 2, 2, 2, 1, 1, 2, 2, 2, 2, 1, 1, 2, 2, 2, 2, 2, 2, 4 ),
 ( 0.000000000000000000, 0.1250000000000807410, 0.1875000000001225964, 0.2187500000001417200, 0.2343750000001512956, 0.2421875000001560141, 0.2460937500001563749, 0.2500000000001567080, 0.3750000000001619260, 0.4375000000001644795, 0.4687500000001657008, 0.4843750000001652012, 0.4921875000001638689, 0.5000000000001625367, 0.6250000000001205702, 0.6875000000001005862, 0.7187500000000905942, 0.7500000000000804912, 1.000000000000000000 ),
 .UNSPECIFIED. ) ;
#5878=B_SPLINE_SURFACE_WITH_KNOTS ( 'NONE', 5, 5, ( 
 ( #21073, #27900, #16832, #10243, #19528, #28413 ),
 ( #26316, #1990, #10684, #13027, #6341, #15206 ),
 ( #24119, #6792, #15655, #28765, #26459, #24557 ),
 ( #8951, #19881, #6492, #4452, #10832, #15351 ),
 ( #28628, #4596, #17862, #19456, #102, #13473 ),
 ( #13322, #28488, #17566, #19740, #26759, #22378 ) ),
 .UNSPECIFIED., .F., .F., .F.,
 ( 6, 6 ),
 ( 6, 6 ),
 ( 6.164978647489999068E-14, 3.318582256960000088 ),
 ( 0.000000000000000000, 0.5000000000000000000 ),
 .UNSPECIFIED. ) ;
#5879=CARTESIAN_POINT ( 'NONE',  ( 21.68616571579999786, -36.53050720059999890, -9.276357967610000088 ) ) ;
#5882=( NAMED_UNIT ( * ) SI_UNIT ( $, .STERADIAN. ) SOLID_ANGLE_UNIT ( ) );
#5884=VERTEX_POINT ( 'NONE', #2218 ) ;
#5885=EDGE_CURVE ( 'NONE', #27953, #10144, #17589, .T. ) ;
#5888=CARTESIAN_POINT ( 'NONE',  ( -7.309593153519999831, -74.20682108740001581, 39.90427328519999861 ) ) ;
#5889=CARTESIAN_POINT ( 'NONE',  ( 36.74383121569999844, -74.66666669110000498, -14.69280905019999928 ) ) ;
#5890=CARTESIAN_POINT ( 'NONE',  ( 0.000000000000000000, -65.07443093669999712, 0.000000000000000000 ) ) ;
#5891=EDGE_CURVE ( 'NONE', #13332, #23505, #23827, .T. ) ;
#5892=CARTESIAN_POINT ( 'NONE',  ( 20.30649716989999831, -72.92631715480000310, -31.15598209699999543 ) ) ;
#5893=CARTESIAN_POINT ( 'NONE',  ( -22.62045161340000021, -72.18745079350000537, 17.95000703219999849 ) ) ;
#5894=DIRECTION ( 'NONE',  ( 1.000000000000000000, 0.000000000000000000, 0.000000000000000000 ) ) ;
#5895=CARTESIAN_POINT ( 'NONE',  ( -19.07003705186754772, -19.48618186053298729, 13.97615460328316850 ) ) ;
#5896=CARTESIAN_POINT ( 'NONE',  ( 0.000000000000000000, -77.00000000000000000, 40.00000000000000000 ) ) ;
#5897=CARTESIAN_POINT ( 'NONE',  ( 7.275524202149999731, -35.36119132620000016, -21.39448337560000013 ) ) ;
#5899=ORIENTED_EDGE ( 'NONE', *, *, #6622, .T. ) ;
#5902=ADVANCED_FACE ( 'NONE', ( #27721 ), #935, .F. ) ;
#5903=CARTESIAN_POINT ( 'NONE',  ( -0.8216735425519999803, -65.07443087359999367, -25.13632629549999820 ) ) ;
#5907=VERTEX_POINT ( 'NONE', #495 ) ;
#5908=CARTESIAN_POINT ( 'NONE',  ( 21.52374314169999892, -36.14100892300000112, -6.944365564089999943 ) ) ;
#5911=CARTESIAN_POINT ( 'NONE',  ( 7.680736482459486147, -37.36815571398255287, -21.51429411660182112 ) ) ;
#5914=CARTESIAN_POINT ( 'NONE',  ( -22.19754890820426141, -74.24418269597721576, -32.70460539598555272 ) ) ;
#5915=AXIS2_PLACEMENT_3D ( 'NONE', #9650, #14032, #14460 ) ;
#5916=CARTESIAN_POINT ( 'NONE',  ( 22.58213840700000219, -18.62337006899999992, 9.587758752840001009 ) ) ;
#5918=CARTESIAN_POINT ( 'NONE',  ( -20.69822367649999961, -60.21448500349999478, 14.94573686989999928 ) ) ;
#5919=ORIENTED_EDGE ( 'NONE', *, *, #21438, .T. ) ;
#5920=DIRECTION ( 'NONE',  ( 0.000000000000000000, 1.000000000000000000, 0.000000000000000000 ) ) ;
#5922=CARTESIAN_POINT ( 'NONE',  ( -7.242462472455940770, -73.74610187082289769, 39.62162972294830610 ) ) ;
#5927=CARTESIAN_POINT ( 'NONE',  ( 36.90882362299999642, -79.77892039240001054, -14.42426562490000030 ) ) ;
#5929=B_SPLINE_SURFACE_WITH_KNOTS ( 'NONE', 5, 5, ( 
 ( #17015, #19199, #1178, #3343, #3616, #12619 ),
 ( #18796, #25902, #10289, #27688, #7726, #21810 ),
 ( #14947, #26333, #4177, #23853, #3894, #24141 ),
 ( #13050, #13343, #127, #19760, #22110, #8823 ),
 ( #19621, #17739, #26041, #21668, #26624, #15223 ),
 ( #8675, #6663, #17587, #4328, #1718, #28505 ),
 ( #2151, #17448, #22248, #8545, #21961, #6066 ),
 ( #19472, #12757, #10558, #28361, #8392, #6359 ),
 ( #17298, #26190, #2010, #6221, #26476, #1864 ),
 ( #21057, #5598, #682, #16381, #16530, #18868 ),
 ( #5170, #1116, #23377, #22809, #827, #3419 ),
 ( #12284, #7663, #27177, #9816, #22961, #18581 ) ),
 .UNSPECIFIED., .F., .F., .F.,
 ( 6, 3, 3, 6 ),
 ( 6, 6 ),
 ( 1.571604936880000172E-14, 0.7090651247770000110, 1.217987177950000000, 1.662727347059999916 ),
 ( 0.000000000000000000, 0.5000000000000000000 ),
 .UNSPECIFIED. ) ;
#5932=CARTESIAN_POINT ( 'NONE',  ( -1.788420423618143573, -80.14911468510305781, 47.02595689713370319 ) ) ;
#5935=AXIS2_PLACEMENT_3D ( 'NONE', #7733, #11935, #4815 ) ;
#5937=EDGE_LOOP ( 'NONE', ( #28726, #20105, #21031 ) ) ;
#5939=CARTESIAN_POINT ( 'NONE',  ( 7.215414233289999757, -74.50000000000000000, 40.70731707320000226 ) ) ;
#5941=EDGE_CURVE ( 'NONE', #9669, #11676, #6799, .T. ) ;
#5944=FACE_OUTER_BOUND ( 'NONE', #14968, .T. ) ;
#5946=CARTESIAN_POINT ( 'NONE',  ( -2.664535259099999805E-15, -72.00000000000000000, -3.552713678799999608E-15 ) ) ;
#5948=ORIENTED_EDGE ( 'NONE', *, *, #7129, .T. ) ;
#5951=CARTESIAN_POINT ( 'NONE',  ( 24.49010421493784406, -63.63799308313229375, -0.5178719358674350737 ) ) ;
#5952=B_SPLINE_CURVE_WITH_KNOTS ( 'NONE', 5,
 ( #28555, #17493, #2499, #24337, #11354, #18075 ),
 .UNSPECIFIED., .F., .F.,
 ( 6, 6 ),
 ( 0.000000000000000000, 1.000000000000000000 ),
 .UNSPECIFIED. ) ;
#5954=CARTESIAN_POINT ( 'NONE',  ( -0.8452062098810000368, -52.63280639840000674, -23.17863372589999926 ) ) ;
#5955=CARTESIAN_POINT ( 'NONE',  ( -2.982732789429999976, -80.14658269599999585, 46.75678581369999876 ) ) ;
#5958=AXIS2_PLACEMENT_3D ( 'NONE', #4357, #6990, #4203 ) ;
#5962=CARTESIAN_POINT ( 'NONE',  ( 18.48933855830000184, -18.50000000000000000, 10.02928721039999971 ) ) ;
#5963=CARTESIAN_POINT ( 'NONE',  ( -14.52092404085399480, -74.11005257168056914, 36.26393844516264409 ) ) ;
#5964=( NAMED_UNIT ( * ) PLANE_ANGLE_UNIT ( ) SI_UNIT ( $, .RADIAN. ) );
#5966=EDGE_CURVE ( 'NONE', #17644, #6901, #11821, .T. ) ;
#5968=CARTESIAN_POINT ( 'NONE',  ( -39.82679900524143335, -73.86845561502485680, -7.247933038825284058 ) ) ;
#5969=EDGE_LOOP ( 'NONE', ( #11104, #6444, #18054, #28598 ) ) ;
#5970=CARTESIAN_POINT ( 'NONE',  ( 20.13916512639999823, -35.75711592529999194, -8.969779973209998758 ) ) ;
#5972=EDGE_CURVE ( 'NONE', #27517, #3056, #24000, .T. ) ;
#5976=AXIS2_PLACEMENT_3D ( 'NONE', #18926, #5920, #3606 ) ;
#5977=LINE ( 'NONE', #10606, #22843 ) ;
#5982=CARTESIAN_POINT ( 'NONE',  ( 9.030336851690002220, -49.07760086190000237, -22.46437391599999955 ) ) ;
#5987=CARTESIAN_POINT ( 'NONE',  ( 39.82679900458370525, -73.86845561458682141, 7.247933038809558859 ) ) ;
#5989=CARTESIAN_POINT ( 'NONE',  ( -13.91698628299999996, -74.00000000000000000, 36.28539016370000070 ) ) ;
#5990=CARTESIAN_POINT ( 'NONE',  ( -14.59449648670000066, -74.30694342880001102, 36.46277468150000090 ) ) ;
#5991=CARTESIAN_POINT ( 'NONE',  ( -0.9323766011660000741, -19.46563609400000061, -22.01671729150000090 ) ) ;
#5992=DIRECTION ( 'NONE',  ( 0.000000000000000000, 1.000000000000000000, 0.000000000000000000 ) ) ;
#5993=ORIENTED_EDGE ( 'NONE', *, *, #18441, .T. ) ;
#5995=CIRCLE ( 'NONE', #7427, 0.5000000000000004441 ) ;
#5996=CARTESIAN_POINT ( 'NONE',  ( 41.00000000000000000, -84.00000000000000000, 10.20110288159999890 ) ) ;
#5997=CARTESIAN_POINT ( 'NONE',  ( 9.592815379950000221, -63.15675378939999973, -23.84803803759999852 ) ) ;
#5999=CARTESIAN_POINT ( 'NONE',  ( 23.16843193700000114, -58.19955223950000089, 10.39065333399999957 ) ) ;
#6000=CARTESIAN_POINT ( 'NONE',  ( -10.66143851719999880, -19.46147658920000012, -19.56664533329999855 ) ) ;
#6001=VERTEX_POINT ( 'NONE', #11668 ) ;
#6002=AXIS2_PLACEMENT_3D ( 'NONE', #14365, #26798, #6830 ) ;
#6003=CIRCLE ( 'NONE', #14408, 3.750000000000000000 ) ;
#6009=CARTESIAN_POINT ( 'NONE',  ( 23.61771397852908905, -61.89519144020896135, 10.58390714728316517 ) ) ;
#6010=CARTESIAN_POINT ( 'NONE',  ( -12.97028186550000051, -64.93834961630000180, 21.65804104839999766 ) ) ;
#6011=ORIENTED_EDGE ( 'NONE', *, *, #20744, .F. ) ;
#6017=DIRECTION ( 'NONE',  ( 1.000000000000000000, 0.000000000000000000, 0.000000000000000000 ) ) ;
#6019=VERTEX_POINT ( 'NONE', #27141 ) ;
#6020=AXIS2_PLACEMENT_3D ( 'NONE', #24705, #5328, #27039 ) ;
#6024=DIRECTION ( 'NONE',  ( 0.000000000000000000, -1.000000000000000000, 0.000000000000000000 ) ) ;
#6025=CARTESIAN_POINT ( 'NONE',  ( 19.43005615430000077, -18.50000000000000000, -7.795798979470000667 ) ) ;
#6028=CARTESIAN_POINT ( 'NONE',  ( -19.03017963434894355, -19.48524588021119897, 13.93486461670488019 ) ) ;
#6030=ORIENTED_EDGE ( 'NONE', *, *, #10677, .F. ) ;
#6031=CARTESIAN_POINT ( 'NONE',  ( 8.242644157730001808, -18.61945111320000024, -19.92601236959999866 ) ) ;
#6032=VERTEX_POINT ( 'NONE', #7181 ) ;
#6033=CARTESIAN_POINT ( 'NONE',  ( 22.45851445570000138, -37.35781404580000498, -9.270563969170000362 ) ) ;
#6036=ADVANCED_FACE ( 'NONE', ( #25251 ), #11431, .T. ) ;
#6037=CARTESIAN_POINT ( 'NONE',  ( -1.246792988649999989, -63.98660223360000288, -24.68432187749999684 ) ) ;
#6039=EDGE_CURVE ( 'NONE', #16955, #4550, #2811, .T. ) ;
#6040=LINE ( 'NONE', #27926, #10564 ) ;
#6041=CARTESIAN_POINT ( 'NONE',  ( -10.20110288159999890, -82.25000000000000000, 41.00000000000000000 ) ) ;
#6043=DIRECTION ( 'NONE',  ( 1.000000000000000000, 0.000000000000000000, 0.000000000000000000 ) ) ;
#6045=CARTESIAN_POINT ( 'NONE',  ( 21.43032141470000340, -35.85552704899999554, -7.415723140210000786 ) ) ;
#6046=CARTESIAN_POINT ( 'NONE',  ( -13.24460949609980176, -57.44036993108258571, 20.55651328139954970 ) ) ;
#6048=DIRECTION ( 'NONE',  ( 0.000000000000000000, 1.000000000000000000, 0.000000000000000000 ) ) ;
#6049=ORIENTED_EDGE ( 'NONE', *, *, #17536, .T. ) ;
#6050=CARTESIAN_POINT ( 'NONE',  ( -14.48711453910000024, -79.93770852559998730, 37.01826959139999929 ) ) ;
#6051=AXIS2_PLACEMENT_3D ( 'NONE', #14639, #25723, #1266 ) ;
#6052=CARTESIAN_POINT ( 'NONE',  ( -18.17465718120000062, -18.50000000000000000, 14.49293709880000058 ) ) ;
#6056=CARTESIAN_POINT ( 'NONE',  ( -32.83566817743611210, -74.45672837283663625, -22.22906645946389403 ) ) ;
#6057=CARTESIAN_POINT ( 'NONE',  ( -19.94071978170000392, -58.91580639759999372, 14.22745801819999834 ) ) ;
#6059=ORIENTED_EDGE ( 'NONE', *, *, #7944, .F. ) ;
#6060=FACE_OUTER_BOUND ( 'NONE', #4398, .T. ) ;
#6062=CARTESIAN_POINT ( 'NONE',  ( -0.5819109535500001096, -18.85523519099999845, -21.88665078049999835 ) ) ;
#6064=EDGE_LOOP ( 'NONE', ( #3763, #680, #23058, #14391, #26968, #10930, #875, #19809, #25627 ) ) ;
#6066=CARTESIAN_POINT ( 'NONE',  ( -32.53182592119999583, -74.14930846740000447, -21.71085396679999846 ) ) ;
#6067=CARTESIAN_POINT ( 'NONE',  ( 36.59060436630000623, -79.00000000000000000, -14.75000000000000000 ) ) ;
#6070=CARTESIAN_POINT ( 'NONE',  ( 36.80498107454818069, -79.53797605812111726, -14.59361009559306588 ) ) ;
#6073=CARTESIAN_POINT ( 'NONE',  ( -3.562216332169999777, -80.49999996399999702, 46.31451619710000500 ) ) ;
#6077=VECTOR ( 'NONE', #2546, 1000.000000000000000 ) ;
#6078=FACE_OUTER_BOUND ( 'NONE', #24803, .T. ) ;
#6080=B_SPLINE_CURVE_WITH_KNOTS ( 'NONE', 5,
 ( #21575, #24037, #8296, #28263, #23760, #23903, #19804, #28684, #1631, #24335, #1762, #19662 ),
 .UNSPECIFIED., .F., .F.,
 ( 6, 3, 3, 6 ),
 ( 0.000000000000000000, 0.5344641413661697094, 0.6876411154090131816, 0.9548616571615552440 ),
 .UNSPECIFIED. ) ;
#6083=DIRECTION ( 'NONE',  ( 0.000000000000000000, -1.000000000000000000, 0.000000000000000000 ) ) ;
#6084=ORIENTED_EDGE ( 'NONE', *, *, #16719, .T. ) ;
#6085=DIRECTION ( 'NONE',  ( -0.8479091047340884257, 0.000000000000000000, 0.5301416321220554506 ) ) ;
#6086=CARTESIAN_POINT ( 'NONE',  ( -10.20110288159999890, -80.50000000000000000, 41.00000000000000000 ) ) ;
#6089=CARTESIAN_POINT ( 'NONE',  ( -2.934623177220000212, -18.50000000000000000, -22.07839963489999846 ) ) ;
#6094=EDGE_CURVE ( 'NONE', #5668, #3611, #18968, .T. ) ;
#6097=AXIS2_PLACEMENT_3D ( 'NONE', #9043, #2807, #7316 ) ;
#6098=CARTESIAN_POINT ( 'NONE',  ( 10.84021880913943292, -72.51523419968246742, -26.83307298900866655 ) ) ;
#6099=CARTESIAN_POINT ( 'NONE',  ( -12.41807177957389641, -68.06111460909730226, -23.59935023276523225 ) ) ;
#6100=ORIENTED_EDGE ( 'NONE', *, *, #25179, .T. ) ;
#6102=CARTESIAN_POINT ( 'NONE',  ( 21.92880676370000259, -37.95796630400000282, -8.677144394200000832 ) ) ;
#6106=CARTESIAN_POINT ( 'NONE',  ( 40.00000000000000000, -74.50000000000000000, 2.433892081919999696E-15 ) ) ;
#6108=CARTESIAN_POINT ( 'NONE',  ( -14.43041715065195163, -70.42331188428948963, 23.51227004908529139 ) ) ;
#6109=SHAPE_REPRESENTATION_RELATIONSHIP ( 'NONE' , 'NONE' ,  #10734, #4297 ) ;
#6112=CARTESIAN_POINT ( 'NONE',  ( -40.38463872098324003, -74.25043946812532170, -7.240437622411593388 ) ) ;
#6113=ORIENTED_EDGE ( 'NONE', *, *, #11570, .F. ) ;
#6114=AXIS2_PLACEMENT_3D ( 'NONE', #19425, #6159, #21755 ) ;
#6115=CARTESIAN_POINT ( 'NONE',  ( 20.91612140590000024, -35.95760432899999870, -8.563236930080000420 ) ) ;
#6117=ORIENTED_EDGE ( 'NONE', *, *, #3041, .F. ) ;
#6123=CARTESIAN_POINT ( 'NONE',  ( 7.019998623859999398, -53.29680639659999741, -22.12830645909999916 ) ) ;
#6128=CARTESIAN_POINT ( 'NONE',  ( 23.55258117300000009, -57.47122623430000488, 0.3294352490589999571 ) ) ;
#6129=CARTESIAN_POINT ( 'NONE',  ( 24.48314189319999912, -69.76823842119999597, 12.05682714019999935 ) ) ;
#6131=ORIENTED_EDGE ( 'NONE', *, *, #25001, .T. ) ;
#6132=CARTESIAN_POINT ( 'NONE',  ( -40.00100507770000036, -74.03378462380000258, 7.261004788019999268 ) ) ;
#6133=EDGE_CURVE ( 'NONE', #16270, #2022, #9168, .T. ) ;
#6137=EDGE_LOOP ( 'NONE', ( #11922, #693, #25964, #11121 ) ) ;
#6138=EDGE_CURVE ( 'NONE', #23662, #13129, #25547, .T. ) ;
#6139=CARTESIAN_POINT ( 'NONE',  ( 28.91458732679999954, -72.00000191859999177, 3.086547544710000146 ) ) ;
#6140=DIRECTION ( 'NONE',  ( -0.9952295494196655712, 0.000000000000000000, 0.09756097560976655092 ) ) ;
#6141=CARTESIAN_POINT ( 'NONE',  ( 9.320354432040000248, -58.88647179320000191, -23.00258203210000119 ) ) ;
#6142=CARTESIAN_POINT ( 'NONE',  ( -12.09194248459999876, -69.13468671140000765, -24.96157070200000305 ) ) ;
#6144=DIRECTION ( 'NONE',  ( 0.1708373792999891283, 0.000000000000000000, 0.9852992387259373874 ) ) ;
#6147=EDGE_LOOP ( 'NONE', ( #19033, #10645, #25910, #19569 ) ) ;
#6152=CARTESIAN_POINT ( 'NONE',  ( -15.39089091200000148, -74.00000000000000000, 40.15260594389999937 ) ) ;
#6154=CARTESIAN_POINT ( 'NONE',  ( -37.60355029590000697, -74.50000000000000000, 9.356041104380000917 ) ) ;
#6157=CARTESIAN_POINT ( 'NONE',  ( 19.24185463459999923, -28.60070551269999939, -8.999622039089999248 ) ) ;
#6159=DIRECTION ( 'NONE',  ( 1.665334536939999828E-16, 0.000000000000000000, 1.000000000000000000 ) ) ;
#6160=ORIENTED_EDGE ( 'NONE', *, *, #7631, .T. ) ;
#6161=DIRECTION ( 'NONE',  ( 0.000000000000000000, 1.000000000000000000, 0.000000000000000000 ) ) ;
#6163=CARTESIAN_POINT ( 'NONE',  ( 0.000000000000000000, -89.00000000000000000, 0.000000000000000000 ) ) ;
#6164=ORIENTED_EDGE ( 'NONE', *, *, #287, .T. ) ;
#6165=CIRCLE ( 'NONE', #26183, 0.5000000000000004441 ) ;
#6167=VERTEX_POINT ( 'NONE', #3519 ) ;
#6169=CARTESIAN_POINT ( 'NONE',  ( 21.64387302759999798, -18.61794787939999907, -0.4555542569220000226 ) ) ;
#6173=CARTESIAN_POINT ( 'NONE',  ( 19.11795961949999878, -18.50000000000000000, -7.980821806519998951 ) ) ;
#6175=CARTESIAN_POINT ( 'NONE',  ( -23.04876999539999716, -71.79380085219999330, 16.27051555959999973 ) ) ;
#6178=CARTESIAN_POINT ( 'NONE',  ( 9.476129726560001743, -36.00000000000000000, -20.06309461059999677 ) ) ;
#6181=CARTESIAN_POINT ( 'NONE',  ( 7.415722487370000060, -35.85552663179999655, -21.43032142309999699 ) ) ;
#6185=CARTESIAN_POINT ( 'NONE',  ( 8.147944900010001490, -19.16110315519999929, -20.46648291129999819 ) ) ;
#6188=CARTESIAN_POINT ( 'NONE',  ( 21.41593371060000095, -36.06062539690000790, -10.16216188949999832 ) ) ;
#6189=CIRCLE ( 'NONE', #27160, 3.000000000000002665 ) ;
#6190=ORIENTED_EDGE ( 'NONE', *, *, #23181, .T. ) ;
#6191=FACE_OUTER_BOUND ( 'NONE', #1096, .T. ) ;
#6193=CARTESIAN_POINT ( 'NONE',  ( -19.55068289229999934, -53.82492386869999734, 13.58563889210000042 ) ) ;
#6195=EDGE_LOOP ( 'NONE', ( #14617, #18627, #10127, #15577 ) ) ;
#6197=B_SPLINE_CURVE_WITH_KNOTS ( 'NONE', 3,
 ( #3182, #14661, #5496, #23280, #27668, #9995 ),
 .UNSPECIFIED., .F., .F.,
 ( 4, 2, 4 ),
 ( 0.000000000000000000, 0.5000000000000000000, 1.000000000000000000 ),
 .UNSPECIFIED. ) ;
#6198=DIRECTION ( 'NONE',  ( 0.3687499999999814260, 0.000000000000000000, -0.9295286103719527793 ) ) ;
#6205=CIRCLE ( 'NONE', #4344, 2.000000000000000000 ) ;
#6206=CARTESIAN_POINT ( 'NONE',  ( 40.35498444582718491, -74.39270540192882208, 7.250043397140349732 ) ) ;
#6211=ORIENTED_EDGE ( 'NONE', *, *, #5972, .F. ) ;
#6212=DIRECTION ( 'NONE',  ( 0.000000000000000000, 0.000000000000000000, -1.000000000000000000 ) ) ;
#6215=PLANE ( 'NONE',  #213 ) ;
#6218=ADVANCED_FACE ( 'NONE', ( #4652 ), #26403, .F. ) ;
#6221=CARTESIAN_POINT ( 'NONE',  ( -32.63918253220000310, -74.37556698459998472, -21.86237412950000092 ) ) ;
#6222=CARTESIAN_POINT ( 'NONE',  ( -22.32000499276877648, -79.78861691627724895, -32.79741325785565209 ) ) ;
#6223=ORIENTED_EDGE ( 'NONE', *, *, #11601, .T. ) ;
#6225=CARTESIAN_POINT ( 'NONE',  ( -22.43272078519999724, -80.50000000000000000, -32.20769377289999369 ) ) ;
#6229=CARTESIAN_POINT ( 'NONE',  ( 22.22712039270000162, -56.22908209860000284, 10.11290092780000194 ) ) ;
#6230=CARTESIAN_POINT ( 'NONE',  ( -7.215414233289999757, -82.25000000000000000, -40.70731707320000226 ) ) ;
#6232=ORIENTED_EDGE ( 'NONE', *, *, #11565, .T. ) ;
#6234=DIRECTION ( 'NONE',  ( 1.000000000000000000, 0.000000000000000000, 0.000000000000000000 ) ) ;
#6235=B_SPLINE_CURVE_WITH_KNOTS ( 'NONE', 5,
 ( #8289, #16628, #14717, #12104, #8025, #1484 ),
 .UNSPECIFIED., .F., .F.,
 ( 6, 6 ),
 ( 0.000000000000000000, 1.000000000000000000 ),
 .UNSPECIFIED. ) ;
#6237=CARTESIAN_POINT ( 'NONE',  ( 8.838003463759999789, -36.72346566359999542, -21.71672433710000050 ) ) ;
#6239=CARTESIAN_POINT ( 'NONE',  ( 25.58518446212841368, -68.16673579364382363, 10.86874726639485900 ) ) ;
#6240=ORIENTED_EDGE ( 'NONE', *, *, #12300, .T. ) ;
#6245=DIRECTION ( 'NONE',  ( 1.000000000000000000, 0.000000000000000000, 0.000000000000000000 ) ) ;
#6256=DIRECTION ( 'NONE',  ( 0.000000000000000000, -1.000000000000000000, 0.000000000000000000 ) ) ;
#6259=ADVANCED_FACE ( 'NONE', ( #4062 ), #12930, .F. ) ;
#6261=CARTESIAN_POINT ( 'NONE',  ( 24.53235143598864809, -18.49999964046002532, 2.185477904151989392 ) ) ;
#6263=CARTESIAN_POINT ( 'NONE',  ( 20.15567332630000053, -35.83134904089999395, -9.008831785180001717 ) ) ;
#6265=ORIENTED_EDGE ( 'NONE', *, *, #896, .F. ) ;
#6267=CARTESIAN_POINT ( 'NONE',  ( -2.955163290202864612, -65.70113804361405130, -26.82187320845386935 ) ) ;
#6268=TOROIDAL_SURFACE ( 'NONE', #10429, 3.500000000000000000, 0.5000000000000000000 ) ;
#6269=LINE ( 'NONE', #23495, #2548 ) ;
#6270=CARTESIAN_POINT ( 'NONE',  ( -13.16183723299999997, -70.12921532840000793, -24.09258145020000086 ) ) ;
#6271=CARTESIAN_POINT ( 'NONE',  ( 9.272014655150000451, -53.24879282989999751, -22.83553957720000227 ) ) ;
#6273=CARTESIAN_POINT ( 'NONE',  ( 27.35691629450000306, -72.00000000000000000, -11.81987123310000065 ) ) ;
#6274=ORIENTED_EDGE ( 'NONE', *, *, #25423, .T. ) ;
#6275=CARTESIAN_POINT ( 'NONE',  ( 0.000000000000000000, -84.00000000000000000, 40.00000000000000000 ) ) ;
#6276=CARTESIAN_POINT ( 'NONE',  ( 23.36166334209999818, -57.47815921199999423, -0.2645295228999999804 ) ) ;
#6277=CARTESIAN_POINT ( 'NONE',  ( 23.24950849600000069, -64.69849383090000572, 10.72429619139999879 ) ) ;
#6281=CARTESIAN_POINT ( 'NONE',  ( -1.348884344130889978, -65.00127109658718894, -25.13406902656907960 ) ) ;
#6287=CARTESIAN_POINT ( 'NONE',  ( 9.808844109879998996, -64.48635843210000473, -24.34110466499999959 ) ) ;
#6289=CARTESIAN_POINT ( 'NONE',  ( 22.91820467009999618, -58.62494694620000502, 10.26923006039999997 ) ) ;
#6290=CARTESIAN_POINT ( 'NONE',  ( -11.09892319740000133, -42.21394486799999868, -22.03407446800000002 ) ) ;
#6294=B_SPLINE_CURVE_WITH_KNOTS ( 'NONE', 5,
 ( #7971, #7708, #26027, #16861, #5641, #23559 ),
 .UNSPECIFIED., .F., .F.,
 ( 6, 6 ),
 ( 0.000000000000000000, 1.000000000000000000 ),
 .UNSPECIFIED. ) ;
#6298=CARTESIAN_POINT ( 'NONE',  ( 21.03406691489999858, -18.50000000000000000, -0.2329208952929999743 ) ) ;
#6300=VERTEX_POINT ( 'NONE', #24177 ) ;
#6303=CARTESIAN_POINT ( 'NONE',  ( 20.19953095279999999, -19.44973810689999993, -8.528659567000000052 ) ) ;
#6304=DIRECTION ( 'NONE',  ( 1.000000000000000000, 0.000000000000000000, 0.000000000000000000 ) ) ;
#6306=ORIENTED_EDGE ( 'NONE', *, *, #17528, .T. ) ;
#6307=CARTESIAN_POINT ( 'NONE',  ( -11.74920108874028202, -34.67040743928694013, -19.26451607462440663 ) ) ;
#6309=ORIENTED_EDGE ( 'NONE', *, *, #26379, .T. ) ;
#6310=CARTESIAN_POINT ( 'NONE',  ( 8.988129812000000385, -35.79614491170000434, -20.14651233290000221 ) ) ;
#6316=CARTESIAN_POINT ( 'NONE',  ( 22.71729720029999910, -18.50000000000000000, 2.301109238659999612 ) ) ;
#6317=CARTESIAN_POINT ( 'NONE',  ( 19.97576656849999921, -36.00000000000000000, -19.97576656849999921 ) ) ;
#6319=EDGE_LOOP ( 'NONE', ( #839, #8749, #13182, #14553, #17759, #858 ) ) ;
#6322=CARTESIAN_POINT ( 'NONE',  ( 6.717799458580000049, -84.00000000000000000, 40.65853658540000026 ) ) ;
#6325=CARTESIAN_POINT ( 'NONE',  ( -18.91794663875353422, -19.48260761092758386, 13.81468008931694591 ) ) ;
#6327=CIRCLE ( 'NONE', #3998, 7.250000000000000000 ) ;
#6328=CARTESIAN_POINT ( 'NONE',  ( -11.11735237159999912, -18.50000000000000000, 18.07942598360000019 ) ) ;
#6330=CARTESIAN_POINT ( 'NONE',  ( -38.71640881029999548, -73.50000064450000536, -7.135467304789999687 ) ) ;
#6332=CARTESIAN_POINT ( 'NONE',  ( -2.379621828269999906, -63.61851004920001174, -25.36216796620000125 ) ) ;
#6333=CARTESIAN_POINT ( 'NONE',  ( 9.858088328779999188, -36.06031159439999811, -21.09473900560000104 ) ) ;
#6335=CARTESIAN_POINT ( 'NONE',  ( -19.75976373869999847, -56.26681992150000156, 12.38608856119999935 ) ) ;
#6336=CARTESIAN_POINT ( 'NONE',  ( -16.49390888960000368, -74.00000000000000000, 44.28897684009999836 ) ) ;
#6337=EDGE_CURVE ( 'NONE', #24581, #11515, #25717, .T. ) ;
#6338=CARTESIAN_POINT ( 'NONE',  ( -12.07243358760000085, -67.46050599719998786, -24.77970463289999969 ) ) ;
#6340=FACE_OUTER_BOUND ( 'NONE', #23932, .T. ) ;
#6341=CARTESIAN_POINT ( 'NONE',  ( 7.255206491240000055, -74.34472676620001153, -40.30310653799999443 ) ) ;
#6342=VERTEX_POINT ( 'NONE', #19200 ) ;
#6343=EDGE_CURVE ( 'NONE', #26105, #27046, #16873, .T. ) ;
#6345=EDGE_CURVE ( 'NONE', #5383, #25644, #18587, .T. ) ;
#6346=CARTESIAN_POINT ( 'NONE',  ( -10.54884365010000025, -18.50000000000000000, -18.22394246889999891 ) ) ;
#6347=FACE_OUTER_BOUND ( 'NONE', #7109, .T. ) ;
#6348=CARTESIAN_POINT ( 'NONE',  ( 20.83731409940000034, -18.50000000000000000, 8.681372653689999552 ) ) ;
#6349=CARTESIAN_POINT ( 'NONE',  ( -32.83566817450000030, -79.50000000000000000, -22.22906645670000003 ) ) ;
#6352=ORIENTED_EDGE ( 'NONE', *, *, #19347, .T. ) ;
#6357=VERTEX_POINT ( 'NONE', #25903 ) ;
#6358=CARTESIAN_POINT ( 'NONE',  ( 8.543355817900000204, -37.95349900170000268, -21.83354978650000078 ) ) ;
#6359=CARTESIAN_POINT ( 'NONE',  ( -32.63800352850000053, -74.22019266179999875, -21.66201587429999975 ) ) ;
#6362=CARTESIAN_POINT ( 'NONE',  ( 19.72252123670000401, -35.98036830730000446, -9.327645202300001159 ) ) ;
#6365=ADVANCED_FACE ( 'NONE', ( #25488 ), #1486, .T. ) ;
#6367=VERTEX_POINT ( 'NONE', #7076 ) ;
#6369=CARTESIAN_POINT ( 'NONE',  ( 46.13218886749999825, -73.50000000000000000, -3.897659475159999776 ) ) ;
#6372=CARTESIAN_POINT ( 'NONE',  ( -21.60034899049999879, -79.50000026560000776, -32.77174743160000503 ) ) ;
#6374=ADVANCED_FACE ( 'NONE', ( #15224 ), #142, .F. ) ;
#6375=AXIS2_PLACEMENT_3D ( 'NONE', #20598, #12117, #25537 ) ;
#6377=CARTESIAN_POINT ( 'NONE',  ( -17.94180966909999597, -19.50000000000000000, 18.81731824139999887 ) ) ;
#6381=VERTEX_POINT ( 'NONE', #2702 ) ;
#6387=CARTESIAN_POINT ( 'NONE',  ( 9.901441303826389984, -72.79609598216572408, -26.91377043562950178 ) ) ;
#6388=FACE_OUTER_BOUND ( 'NONE', #5499, .T. ) ;
#6390=CARTESIAN_POINT ( 'NONE',  ( 8.873743607898822106, -64.92653621548541309, -23.73262392692488021 ) ) ;
#6391=DIRECTION ( 'NONE',  ( 1.000000000000000000, 0.000000000000000000, 0.000000000000000000 ) ) ;
#6393=CARTESIAN_POINT ( 'NONE',  ( 19.60237952920000026, -18.50000000000000000, 8.863026849229999726 ) ) ;
#6397=FACE_OUTER_BOUND ( 'NONE', #1745, .T. ) ;
#6398=VERTEX_POINT ( 'NONE', #6515 ) ;
#6399=EDGE_CURVE ( 'NONE', #6381, #8240, #27629, .T. ) ;
#6407=CARTESIAN_POINT ( 'NONE',  ( 8.036479196959999201E-15, -69.00000000000000000, -43.75000000000000000 ) ) ;
#6413=CARTESIAN_POINT ( 'NONE',  ( -10.66687304220000065, -18.85531889179999965, -19.32093941720000174 ) ) ;
#6416=TOROIDAL_SURFACE ( 'NONE', #5958, 6.750000000000000000, 0.5000000000000000000 ) ;
#6418=CARTESIAN_POINT ( 'NONE',  ( 22.55812702580000106, -34.66943697789999845, -0.5428458454240000508 ) ) ;
#6423=DIRECTION ( 'NONE',  ( -1.836909530730000236E-16, 0.000000000000000000, 1.000000000000000000 ) ) ;
#6425=CARTESIAN_POINT ( 'NONE',  ( -10.17458377400000025, -18.50000000000000000, -22.50859265919999785 ) ) ;
#6426=VERTEX_POINT ( 'NONE', #23102 ) ;
#6430=CARTESIAN_POINT ( 'NONE',  ( 24.28331883913842404, -74.17350752487904231, -30.68182624356128585 ) ) ;
#6431=CARTESIAN_POINT ( 'NONE',  ( -12.04650979770000063, -69.29982785389999833, -25.46956491610000128 ) ) ;
#6432=DIRECTION ( 'NONE',  ( 0.000000000000000000, 1.000000000000000000, 0.000000000000000000 ) ) ;
#6433=CARTESIAN_POINT ( 'NONE',  ( -11.22052832319999816, -34.66889731630000426, -19.66680200659999755 ) ) ;
#6435=DIRECTION ( 'NONE',  ( 0.000000000000000000, 1.000000000000000000, 0.000000000000000000 ) ) ;
#6437=CIRCLE ( 'NONE', #26955, 1.000000000000000888 ) ;
#6439=EDGE_CURVE ( 'NONE', #1612, #3048, #8139, .T. ) ;
#6444=ORIENTED_EDGE ( 'NONE', *, *, #9972, .T. ) ;
#6446=CARTESIAN_POINT ( 'NONE',  ( 40.00000000000000000, -69.00000000000000000, 5.456746166030000766E-15 ) ) ;
#6449=CARTESIAN_POINT ( 'NONE',  ( 27.35691629450000306, -72.00000000000000000, -11.81987123310000065 ) ) ;
#6450=DIRECTION ( 'NONE',  ( 0.7071067811865475727, 0.000000000000000000, 0.7071067811865475727 ) ) ;
#6452=DIRECTION ( 'NONE',  ( 0.000000000000000000, 0.000000000000000000, -1.000000000000000000 ) ) ;
#6453=CARTESIAN_POINT ( 'NONE',  ( 6.717799458580000049, -84.00000000000000000, -40.65853658540000026 ) ) ;
#6456=DIRECTION ( 'NONE',  ( 0.09756097560976667582, 0.000000000000000000, 0.9952295494196654602 ) ) ;
#6460=ORIENTED_EDGE ( 'NONE', *, *, #26020, .F. ) ;
#6462=CARTESIAN_POINT ( 'NONE',  ( 28.28064714961420378, -69.93672243438709302, 2.457583639001003295 ) ) ;
#6467=B_SPLINE_CURVE_WITH_KNOTS ( 'NONE', 5,
 ( #21004, #18822, #27711, #7750, #14563, #27977 ),
 .UNSPECIFIED., .F., .F.,
 ( 6, 6 ),
 ( 0.000000000000000000, 1.000000000000000000 ),
 .UNSPECIFIED. ) ;
#6468=EDGE_CURVE ( 'NONE', #21056, #27454, #2961, .T. ) ;
#6470=EDGE_CURVE ( 'NONE', #21012, #15974, #11272, .T. ) ;
#6472=CYLINDRICAL_SURFACE ( 'NONE', #11499, 2.999999999999996447 ) ;
#6477=CARTESIAN_POINT ( 'NONE',  ( 8.654032102250001302, -18.62337004359999781, -18.91112466639999923 ) ) ;
#6478=CARTESIAN_POINT ( 'NONE',  ( 22.18469061490000271, -36.06131723480000062, -10.59598294889999970 ) ) ;
#6481=CARTESIAN_POINT ( 'NONE',  ( -13.78316409329999814, -60.27285653700000267, 21.13754188760000119 ) ) ;
#6482=AXIS2_PLACEMENT_3D ( 'NONE', #1001, #7694, #1272 ) ;
#6483=CARTESIAN_POINT ( 'NONE',  ( 8.887092021739999126, -37.65454143339999860, -22.08144368150000147 ) ) ;
#6486=CARTESIAN_POINT ( 'NONE',  ( 4.534235129290000123E-15, -79.00000000000000000, -36.25000000000000000 ) ) ;
#6487=CIRCLE ( 'NONE', #18127, 0.5000000000000004441 ) ;
#6490=EDGE_LOOP ( 'NONE', ( #3090, #7374 ) ) ;
#6492=CARTESIAN_POINT ( 'NONE',  ( 7.279149876880000036, -73.90055525929999192, -39.59129699409999859 ) ) ;
#6493=ORIENTED_EDGE ( 'NONE', *, *, #15750, .T. ) ;
#6499=CARTESIAN_POINT ( 'NONE',  ( -7.851152467529999512, -74.00000000000000000, 38.40621260480000387 ) ) ;
#6501=CARTESIAN_POINT ( 'NONE',  ( 9.975420127400001391, -67.81624775490000445, -25.13735964720000027 ) ) ;
#6502=CARTESIAN_POINT ( 'NONE',  ( -19.68647263579999773, -57.47571016759999907, 12.70082573810000071 ) ) ;
#6504=CARTESIAN_POINT ( 'NONE',  ( -13.80673513442132183, -68.20222041995040740, 22.71145971957957244 ) ) ;
#6505=DIRECTION ( 'NONE',  ( -0.9704142011833034598, 0.000000000000000000, -0.2414462220490750932 ) ) ;
#6508=CARTESIAN_POINT ( 'NONE',  ( -7.227556247458971406, -73.66327267196029993, 39.42995888277184235 ) ) ;
#6509=CARTESIAN_POINT ( 'NONE',  ( -40.70731707320000226, -74.50000000000000000, -7.215414233289999757 ) ) ;
#6510=EDGE_LOOP ( 'NONE', ( #26235, #2459, #7791, #10040, #23414 ) ) ;
#6511=VECTOR ( 'NONE', #9025, 1000.000000000000000 ) ;
#6513=AXIS2_PLACEMENT_3D ( 'NONE', #5773, #6198, #17278 ) ;
#6515=CARTESIAN_POINT ( 'NONE',  ( 24.39713799250000292, -19.50000027030000282, 1.459766484860000046 ) ) ;
#6519=DIRECTION ( 'NONE',  ( 0.000000000000000000, 1.000000000000000000, 0.000000000000000000 ) ) ;
#6520=FACE_OUTER_BOUND ( 'NONE', #26283, .T. ) ;
#6522=EDGE_LOOP ( 'NONE', ( #13192, #9087, #8604, #9743, #10318, #21769 ) ) ;
#6525=VERTEX_POINT ( 'NONE', #20625 ) ;
#6527=CARTESIAN_POINT ( 'NONE',  ( -6.717799458580000049, -84.00000000000000000, 40.65853658540000026 ) ) ;
#6531=DIRECTION ( 'NONE',  ( 0.000000000000000000, 0.000000000000000000, -1.000000000000000000 ) ) ;
#6535=DIRECTION ( 'NONE',  ( 1.000000000000000000, 0.000000000000000000, 0.000000000000000000 ) ) ;
#6537=DIRECTION ( 'NONE',  ( 0.000000000000000000, 1.000000000000000000, 0.000000000000000000 ) ) ;
#6543=CARTESIAN_POINT ( 'NONE',  ( -17.64372670299999868, -18.50000000000000000, 13.83547606110000139 ) ) ;
#6549=DIRECTION ( 'NONE',  ( 0.000000000000000000, 1.000000000000000000, 0.000000000000000000 ) ) ;
#6552=LINE ( 'NONE', #18062, #15408 ) ;
#6555=AXIS2_PLACEMENT_3D ( 'NONE', #35, #19817, #10765 ) ;
#6559=EDGE_LOOP ( 'NONE', ( #14882, #16570, #23326 ) ) ;
#6561=ORIENTED_EDGE ( 'NONE', *, *, #22702, .T. ) ;
#6562=CARTESIAN_POINT ( 'NONE',  ( 28.76419640220090912, -72.15620615179069830, 2.906284881040829937 ) ) ;
#6564=ORIENTED_EDGE ( 'NONE', *, *, #19034, .T. ) ;
#6566=ORIENTED_EDGE ( 'NONE', *, *, #25804, .T. ) ;
#6568=DIRECTION ( 'NONE',  ( 0.000000000000000000, 1.000000000000000000, 0.000000000000000000 ) ) ;
#6570=CARTESIAN_POINT ( 'NONE',  ( -10.89815230080000141, -18.50000000000000000, -17.99090062400000178 ) ) ;
#6574=AXIS2_PLACEMENT_3D ( 'NONE', #11075, #4554, #25940 ) ;
#6577=CARTESIAN_POINT ( 'NONE',  ( 23.56468125250000156, -27.03158754569999900, 1.355479213289999985 ) ) ;
#6578=CARTESIAN_POINT ( 'NONE',  ( 25.14778840239999980, -69.33908554340000308, 11.07326088209999959 ) ) ;
#6579=CARTESIAN_POINT ( 'NONE',  ( 40.28633210762483685, -74.17816432815648398, 7.244343739438153129 ) ) ;
#6580=ORIENTED_EDGE ( 'NONE', *, *, #5206, .F. ) ;
#6585=ADVANCED_FACE ( 'NONE', ( #98 ), #2572, .T. ) ;
#6586=CARTESIAN_POINT ( 'NONE',  ( 0.000000000000000000, -65.07443093669999712, 0.000000000000000000 ) ) ;
#6589=CARTESIAN_POINT ( 'NONE',  ( -12.05824332719999958, -67.66818001709999919, -24.37626866669999970 ) ) ;
#6590=CARTESIAN_POINT ( 'NONE',  ( 24.34110602900000231, -64.48636181450000038, -9.808841899269999942 ) ) ;
#6591=ORIENTED_EDGE ( 'NONE', *, *, #626, .T. ) ;
#6593=DIRECTION ( 'NONE',  ( 0.000000000000000000, 1.000000000000000000, 0.000000000000000000 ) ) ;
#6594=CARTESIAN_POINT ( 'NONE',  ( -11.18243144779999909, -57.47855601759999900, 20.51090144570000007 ) ) ;
#6595=CARTESIAN_POINT ( 'NONE',  ( 37.60355029590000697, -74.00000000000000000, -9.356041104380000917 ) ) ;
#6597=AXIS2_PLACEMENT_3D ( 'NONE', #17189, #3931, #3522 ) ;
#6604=EDGE_CURVE ( 'NONE', #24784, #11872, #27311, .T. ) ;
#6605=DIRECTION ( 'NONE',  ( 1.000000000000000000, 0.000000000000000000, 0.000000000000000000 ) ) ;
#6608=CARTESIAN_POINT ( 'NONE',  ( -3.807886452449999570, -80.00000000000000000, 46.75000000000000000 ) ) ;
#6611=CARTESIAN_POINT ( 'NONE',  ( -17.94180966909999597, -19.50000000000000000, 18.81731824139999887 ) ) ;
#6612=CARTESIAN_POINT ( 'NONE',  ( 21.56931447779999900, -36.56979901409999911, -6.850353625240000355 ) ) ;
#6614=AXIS2_PLACEMENT_3D ( 'NONE', #13324, #17429, #105 ) ;
#6618=CARTESIAN_POINT ( 'NONE',  ( 0.000000000000000000, -80.50000000000000000, 0.000000000000000000 ) ) ;
#6619=CIRCLE ( 'NONE', #2450, 7.249999999999999112 ) ;
#6622=EDGE_CURVE ( 'NONE', #4330, #24784, #14090, .T. ) ;
#6623=CARTESIAN_POINT ( 'NONE',  ( -40.00000000000000000, -74.50000000000000000, 2.464695114669999848E-15 ) ) ;
#6624=LINE ( 'NONE', #19862, #15253 ) ;
#6625=CARTESIAN_POINT ( 'NONE',  ( -11.98644653210000044, -66.39602363730000434, -23.89227711550000066 ) ) ;
#6630=CARTESIAN_POINT ( 'NONE',  ( 8.028473304129999377, -18.50000000000000000, -18.85230009969999898 ) ) ;
#6633=CIRCLE ( 'NONE', #2932, 11.00000000000000000 ) ;
#6634=CARTESIAN_POINT ( 'NONE',  ( -14.19074604640000103, -64.47177095450000195, 21.84081649480000209 ) ) ;
#6635=DIRECTION ( 'NONE',  ( 1.000000000000000000, 0.000000000000000000, 0.000000000000000000 ) ) ;
#6637=AXIS2_PLACEMENT_3D ( 'NONE', #8760, #14457, #21033 ) ;
#6638=DIRECTION ( 'NONE',  ( 1.000000000000000000, 0.000000000000000000, 0.000000000000000000 ) ) ;
#6639=DIRECTION ( 'NONE',  ( 0.000000000000000000, -1.000000000000000000, 0.000000000000000000 ) ) ;
#6640=EDGE_CURVE ( 'NONE', #5430, #19506, #12222, .T. ) ;
#6644=ORIENTED_EDGE ( 'NONE', *, *, #3971, .T. ) ;
#6648=CARTESIAN_POINT ( 'NONE',  ( 20.14180068619999631, -45.99906616869999709, 11.02192007709999899 ) ) ;
#6651=CARTESIAN_POINT ( 'NONE',  ( 19.26420165869999934, -18.61776472269999871, 9.888281526900000173 ) ) ;
#6652=CARTESIAN_POINT ( 'NONE',  ( 8.558198341779998941, -66.59066310410000256, -24.38877182639999930 ) ) ;
#6654=ORIENTED_EDGE ( 'NONE', *, *, #7098, .F. ) ;
#6656=CARTESIAN_POINT ( 'NONE',  ( 27.03296752710000206, -72.21526977780000323, -11.52669541869999925 ) ) ;
#6660=FACE_OUTER_BOUND ( 'NONE', #5508, .T. ) ;
#6662=PLANE ( 'NONE',  #9341 ) ;
#6663=CARTESIAN_POINT ( 'NONE',  ( -32.48735602109999832, -74.14773635299999910, -22.07522367249999817 ) ) ;
#6665=CARTESIAN_POINT ( 'NONE',  ( -10.59381889375850960, -19.48875964712268782, -21.30758956286935302 ) ) ;
#6666=CIRCLE ( 'NONE', #3421, 3.000000000000000000 ) ;
#6667=CARTESIAN_POINT ( 'NONE',  ( 24.99717791306386161, -43.98373191176955999, 1.386805645287898292 ) ) ;
#6671=DIRECTION ( 'NONE',  ( 0.000000000000000000, 1.000000000000000000, 0.000000000000000000 ) ) ;
#6674=CARTESIAN_POINT ( 'NONE',  ( -22.92366483370072672, -71.08353289282860032, 15.88272241998541290 ) ) ;
#6675=CARTESIAN_POINT ( 'NONE',  ( -12.84659744679999882, -72.82938648530000592, -25.64625568420000334 ) ) ;
#6677=ORIENTED_EDGE ( 'NONE', *, *, #25362, .T. ) ;
#6690=AXIS2_PLACEMENT_3D ( 'NONE', #18496, #2630, #455 ) ;
#6692=CARTESIAN_POINT ( 'NONE',  ( -22.11992770129999997, -74.33689811570000927, -32.70527315500000043 ) ) ;
#6693=CARTESIAN_POINT ( 'NONE',  ( -1.156001381979999909, -57.47571038090000428, -23.39939166179999930 ) ) ;
#6697=CARTESIAN_POINT ( 'NONE',  ( 7.479534728624448903, -74.09469053464687249, -39.31221710977964534 ) ) ;
#6698=EDGE_LOOP ( 'NONE', ( #6591, #9773, #27075, #6211 ) ) ;
#6699=CARTESIAN_POINT ( 'NONE',  ( 27.11492913210000211, -72.00000000000000000, 10.50528373760000100 ) ) ;
#6700=DIRECTION ( 'NONE',  ( 0.000000000000000000, 1.000000000000000000, 0.000000000000000000 ) ) ;
#6702=PLANE ( 'NONE',  #20985 ) ;
#6706=CARTESIAN_POINT ( 'NONE',  ( 23.55258138210000141, -57.47122622279999860, 0.3294346322440000474 ) ) ;
#6707=DIRECTION ( 'NONE',  ( 0.000000000000000000, 0.000000000000000000, -1.000000000000000000 ) ) ;
#6709=AXIS2_PLACEMENT_3D ( 'NONE', #17988, #2558, #26442 ) ;
#6711=ORIENTED_EDGE ( 'NONE', *, *, #21645, .T. ) ;
#6713=CARTESIAN_POINT ( 'NONE',  ( 28.56383486739311550, -72.59720960093795838, 2.210274403918753183 ) ) ;
#6714=DIRECTION ( 'NONE',  ( 0.000000000000000000, -1.000000000000000000, 0.000000000000000000 ) ) ;
#6715=EDGE_LOOP ( 'NONE', ( #21260, #21368, #16200, #8715, #20667, #28477 ) ) ;
#6716=FACE_OUTER_BOUND ( 'NONE', #18420, .T. ) ;
#6717=EDGE_CURVE ( 'NONE', #18911, #26338, #25574, .T. ) ;
#6720=CARTESIAN_POINT ( 'NONE',  ( -35.88566914520000495, -80.00000000000000000, -26.69328098980000163 ) ) ;
#6723=DIRECTION ( 'NONE',  ( 0.7071067811865474617, 0.000000000000000000, 0.7071067811865474617 ) ) ;
#6726=EDGE_CURVE ( 'NONE', #3127, #17492, #28439, .T. ) ;
#6729=CARTESIAN_POINT ( 'NONE',  ( -14.93121078260000090, -79.49999975080000070, 36.29905569799999654 ) ) ;
#6732=AXIS2_PLACEMENT_3D ( 'NONE', #7930, #16818, #19145 ) ;
#6733=CARTESIAN_POINT ( 'NONE',  ( -20.56018235820000228, -57.40875686090000585, 14.85415984670000000 ) ) ;
#6737=CARTESIAN_POINT ( 'NONE',  ( 28.37123197869999913, -70.21789636049999217, 2.505359212729999729 ) ) ;
#6740=CARTESIAN_POINT ( 'NONE',  ( 26.04734495227661739, -74.32587665817413836, -29.31966643403540829 ) ) ;
#6741=FACE_OUTER_BOUND ( 'NONE', #15949, .T. ) ;
#6742=CARTESIAN_POINT ( 'NONE',  ( 23.88371843180000198, -64.81171329779999724, -9.133376755849999640 ) ) ;
#6743=CYLINDRICAL_SURFACE ( 'NONE', #17109, 7.250000000000004441 ) ;
#6744=ORIENTED_EDGE ( 'NONE', *, *, #17538, .T. ) ;
#6749=CARTESIAN_POINT ( 'NONE',  ( 7.215414233289999757, -74.50000000000000000, 40.70731707320000226 ) ) ;
#6750=ORIENTED_EDGE ( 'NONE', *, *, #18102, .F. ) ;
#6752=DIRECTION ( 'NONE',  ( 1.000000000000000000, 0.000000000000000000, 0.000000000000000000 ) ) ;
#6755=CARTESIAN_POINT ( 'NONE',  ( 22.73895411410159184, -19.47261671706005970, 1.022399396795566906 ) ) ;
#6756=ORIENTED_EDGE ( 'NONE', *, *, #23539, .F. ) ;
#6757=VECTOR ( 'NONE', #7646, 1000.000000000000000 ) ;
#6758=CARTESIAN_POINT ( 'NONE',  ( 26.80994437584741164, -72.64395437913957210, -10.47635535423811604 ) ) ;
#6760=CARTESIAN_POINT ( 'NONE',  ( 8.371797148759998919, -37.28113868359999827, -21.64024904569999919 ) ) ;
#6761=CARTESIAN_POINT ( 'NONE',  ( 21.44781821315665837, -35.39811109517434318, -7.092598482907919610 ) ) ;
#6762=ORIENTED_EDGE ( 'NONE', *, *, #23979, .F. ) ;
#6766=CARTESIAN_POINT ( 'NONE',  ( 40.00000000000000000, -84.00000000000000000, 0.000000000000000000 ) ) ;
#6767=CYLINDRICAL_SURFACE ( 'NONE', #17261, 4.749999999999999112 ) ;
#6774=CARTESIAN_POINT ( 'NONE',  ( -13.15060416100000040, -67.65187322490000099, -22.80468052719999861 ) ) ;
#6779=CARTESIAN_POINT ( 'NONE',  ( 36.36887047860000166, -75.00000017930000240, -14.85406792070000037 ) ) ;
#6780=VERTEX_POINT ( 'NONE', #9680 ) ;
#6781=CARTESIAN_POINT ( 'NONE',  ( -14.45912934149999884, -67.24379409739999858, 22.35770716749999920 ) ) ;
#6782=CARTESIAN_POINT ( 'NONE',  ( -12.97028186550000051, -64.93834961630000180, 21.65804104839999766 ) ) ;
#6783=DIRECTION ( 'NONE',  ( 0.9279287544047433167, 0.000000000000000000, 0.3727575978418970482 ) ) ;
#6785=CARTESIAN_POINT ( 'NONE',  ( -19.58536422119999543, -55.03616289790000593, 13.60193610299999989 ) ) ;
#6787=CARTESIAN_POINT ( 'NONE',  ( 19.92838004652724138, -19.48035124000026741, -8.655192717976913030 ) ) ;
#6788=CARTESIAN_POINT ( 'NONE',  ( -11.46863496920000003, -57.40875702469999453, -22.62382260909999943 ) ) ;
#6790=FACE_OUTER_BOUND ( 'NONE', #15460, .T. ) ;
#6791=CARTESIAN_POINT ( 'NONE',  ( 28.79684628073619024, -74.38486911952558955, -26.65149887044830734 ) ) ;
#6792=CARTESIAN_POINT ( 'NONE',  ( 7.260991986019999622, -74.03376265059999639, -40.00088823080000111 ) ) ;
#6798=CARTESIAN_POINT ( 'NONE',  ( 21.98573708710000219, -45.96202241439999625, 9.944421315929998784 ) ) ;
#6799=CIRCLE ( 'NONE', #13284, 0.5000000000000004441 ) ;
#6802=CARTESIAN_POINT ( 'NONE',  ( 19.91311854129999759, -18.50000000000000000, 8.957432309550000582 ) ) ;
#6806=CARTESIAN_POINT ( 'NONE',  ( -14.22861622156947092, -68.06112402365553748, 22.55404109828588588 ) ) ;
#6807=CARTESIAN_POINT ( 'NONE',  ( -22.22906645670000003, -74.50000000000000000, -32.83566817450000030 ) ) ;
#6809=CARTESIAN_POINT ( 'NONE',  ( -40.00088823259999771, -74.03376265130000888, -7.260991985950000505 ) ) ;
#6815=LINE ( 'NONE', #8980, #3762 ) ;
#6819=EDGE_CURVE ( 'NONE', #5488, #6001, #20089, .T. ) ;
#6827=CARTESIAN_POINT ( 'NONE',  ( -22.53893513710000107, -80.06168502749999050, -32.36019062569999249 ) ) ;
#6830=DIRECTION ( 'NONE',  ( 1.000000000000000000, 0.000000000000000000, 0.000000000000000000 ) ) ;
#6832=ORIENTED_EDGE ( 'NONE', *, *, #25921, .T. ) ;
#6833=DIRECTION ( 'NONE',  ( 1.000000000000000000, 0.000000000000000000, 0.000000000000000000 ) ) ;
#6835=CARTESIAN_POINT ( 'NONE',  ( -38.71641004229999794, -73.50000000000000000, 7.135467526410000261 ) ) ;
#6836=CARTESIAN_POINT ( 'NONE',  ( -21.88970062429999786, -74.04477437299999565, -32.25615024759999727 ) ) ;
#6837=CARTESIAN_POINT ( 'NONE',  ( -1.450349733809999986, -57.47122622300000216, -23.51019145590000292 ) ) ;
#6839=DIRECTION ( 'NONE',  ( 0.000000000000000000, -1.000000000000000000, 0.000000000000000000 ) ) ;
#6840=CARTESIAN_POINT ( 'NONE',  ( -18.58434179929999885, -19.16559685920000078, 13.41605620019999989 ) ) ;
#6841=ORIENTED_EDGE ( 'NONE', *, *, #3216, .T. ) ;
#6844=EDGE_CURVE ( 'NONE', #18811, #7089, #21485, .T. ) ;
#6845=CARTESIAN_POINT ( 'NONE',  ( 20.30848777263183536, -73.00723796075250505, -31.22327362632934822 ) ) ;
#6848=DIRECTION ( 'NONE',  ( 0.000000000000000000, 1.000000000000000000, 0.000000000000000000 ) ) ;
#6850=B_SPLINE_SURFACE_WITH_KNOTS ( 'NONE', 5, 5, ( 
 ( #13666, #10864, #6827, #15841, #26937, #20223 ),
 ( #13507, #15690, #8687, #141, #22418, #6977 ),
 ( #20367, #8991, #24300, #22126, #11320, #24751 ),
 ( #24451, #24597, #4786, #19916, #4346, #22571 ),
 ( #13065, #4635, #2465, #22263, #8558, #2611 ),
 ( #20078, #11459, #17898, #17461, #26347, #6372 ) ),
 .UNSPECIFIED., .F., .F., .F.,
 ( 6, 6 ),
 ( 6, 6 ),
 ( 2.646611395639999920, 4.419061266649999986 ),
 ( 0.000000000000000000, 0.5000000000000000000 ),
 .UNSPECIFIED. ) ;
#6853=DIRECTION ( 'NONE',  ( 0.000000000000000000, -1.000000000000000000, 0.000000000000000000 ) ) ;
#6857=ORIENTED_EDGE ( 'NONE', *, *, #2617, .F. ) ;
#6866=CARTESIAN_POINT ( 'NONE',  ( -9.771355533599999532, -18.50000000000000000, -22.03737773150000123 ) ) ;
#6870=DIRECTION ( 'NONE',  ( 1.000000000000000000, 0.000000000000000000, 0.000000000000000000 ) ) ;
#6873=CYLINDRICAL_SURFACE ( 'NONE', #25800, 0.5000000000000004441 ) ;
#6875=DIRECTION ( 'NONE',  ( 1.000000000000000000, 0.000000000000000000, 0.000000000000000000 ) ) ;
#6876=EDGE_LOOP ( 'NONE', ( #2406, #1090, #23419 ) ) ;
#6881=CARTESIAN_POINT ( 'NONE',  ( 25.44178589691103554, -74.26977420868146851, -29.81503247152727454 ) ) ;
#6884=CARTESIAN_POINT ( 'NONE',  ( 23.33413376120000038, -63.63811275439999804, -7.452427173000001126 ) ) ;
#6888=B_SPLINE_CURVE_WITH_KNOTS ( 'NONE', 5,
 ( #21757, #14761, #10511, #6307, #21904, #17101 ),
 .UNSPECIFIED., .F., .F.,
 ( 6, 6 ),
 ( 0.000000000000000000, 1.000000000000000000 ),
 .UNSPECIFIED. ) ;
#6895=CARTESIAN_POINT ( 'NONE',  ( -36.25000000000000000, -79.00000000000000000, 2.124561919619999789E-15 ) ) ;
#6897=CARTESIAN_POINT ( 'NONE',  ( 7.260205543919999727, -73.74944613220000633, 39.69269201139999836 ) ) ;
#6899=AXIS2_PLACEMENT_3D ( 'NONE', #16462, #24924, #23172 ) ;
#6900=CARTESIAN_POINT ( 'NONE',  ( 22.21661127598724761, -19.46574300968510229, 0.3417159844211649089 ) ) ;
#6901=VERTEX_POINT ( 'NONE', #13102 ) ;
#6903=CARTESIAN_POINT ( 'NONE',  ( 26.93262652789482559, -72.35629361427136530, -11.21074450457773075 ) ) ;
#6904=CARTESIAN_POINT ( 'NONE',  ( 8.114520564299999350, -37.85480374339999798, -21.62119288240000259 ) ) ;
#6905=CARTESIAN_POINT ( 'NONE',  ( 21.39667837337682599, -35.15480553054729285, -7.218929069207992377 ) ) ;
#6907=DIRECTION ( 'NONE',  ( 0.3687499999999814260, 0.000000000000000000, -0.9295286103719527793 ) ) ;
#6910=CARTESIAN_POINT ( 'NONE',  ( -2.616610288655701666, -19.48999941748984810, -23.72428921426985582 ) ) ;
#6911=ORIENTED_EDGE ( 'NONE', *, *, #25419, .F. ) ;
#6915=CARTESIAN_POINT ( 'NONE',  ( 40.70731707320000226, -84.00000000000000000, 7.215414233289999757 ) ) ;
#6916=CARTESIAN_POINT ( 'NONE',  ( 21.28200145869999815, -36.23996849270000098, -9.082471821829999570 ) ) ;
#6922=EDGE_CURVE ( 'NONE', #8136, #7650, #21657, .T. ) ;
#6923=CARTESIAN_POINT ( 'NONE',  ( 36.70830927769999619, -74.93175448689999030, -14.75000110549999910 ) ) ;
#6928=CARTESIAN_POINT ( 'NONE',  ( -12.04650752959999949, -69.29982884310000202, -25.46956806489999892 ) ) ;
#6929=CARTESIAN_POINT ( 'NONE',  ( -11.57811457420000067, -60.59341626269999637, 20.59243238690000410 ) ) ;
#6930=CARTESIAN_POINT ( 'NONE',  ( 7.244162156032840194, -74.18137224045423750, 40.29089741862549801 ) ) ;
#6931=DIRECTION ( 'NONE',  ( 0.000000000000000000, 1.000000000000000000, 0.000000000000000000 ) ) ;
#6933=DIRECTION ( 'NONE',  ( 1.000000000000000000, 0.000000000000000000, 0.000000000000000000 ) ) ;
#6940=DIRECTION ( 'NONE',  ( 1.000000000000000000, 0.000000000000000000, 0.000000000000000000 ) ) ;
#6944=CARTESIAN_POINT ( 'NONE',  ( 20.34628061889999984, -52.63293862049999916, 11.13082833170000008 ) ) ;
#6945=AXIS2_PLACEMENT_3D ( 'NONE', #3095, #7747, #16613 ) ;
#6948=CARTESIAN_POINT ( 'NONE',  ( 22.07840668539999740, -19.40610837500000230, 9.666972891260000367 ) ) ;
#6952=DIRECTION ( 'NONE',  ( 0.000000000000000000, -1.000000000000000000, 0.000000000000000000 ) ) ;
#6955=DIRECTION ( 'NONE',  ( 0.9942974773630094409, 0.000000000000000000, -0.1066420485059984408 ) ) ;
#6958=CARTESIAN_POINT ( 'NONE',  ( 20.83060772838619457, -19.47440675036266100, 9.481471874783228060 ) ) ;
#6959=CARTESIAN_POINT ( 'NONE',  ( 23.26489703562036127, -63.25226117637114243, -7.438063082557897943 ) ) ;
#6960=ORIENTED_EDGE ( 'NONE', *, *, #18432, .T. ) ;
#6961=ADVANCED_FACE ( 'NONE', ( #10756 ), #15991, .T. ) ;
#6962=AXIS2_PLACEMENT_3D ( 'NONE', #20801, #20655, #16259 ) ;
#6963=DIRECTION ( 'NONE',  ( -0.7071067811865475727, 0.000000000000000000, 0.7071067811865475727 ) ) ;
#6964=ORIENTED_EDGE ( 'NONE', *, *, #25734, .T. ) ;
#6965=AXIS2_PLACEMENT_3D ( 'NONE', #24075, #23939, #3978 ) ;
#6968=CARTESIAN_POINT ( 'NONE',  ( -10.93437413680000070, -19.50000027030000282, -21.85842452360000010 ) ) ;
#6972=CARTESIAN_POINT ( 'NONE',  ( -21.79612357827979707, -66.42276310376364279, 13.73860294033563356 ) ) ;
#6975=ORIENTED_EDGE ( 'NONE', *, *, #10244, .T. ) ;
#6976=LINE ( 'NONE', #13665, #21998 ) ;
#6977=CARTESIAN_POINT ( 'NONE',  ( -22.17563740510000159, -80.50000000000000000, -32.38675284270000532 ) ) ;
#6983=CIRCLE ( 'NONE', #5588, 38.75000000000000000 ) ;
#6984=AXIS2_PLACEMENT_3D ( 'NONE', #6618, #3600, #10005 ) ;
#6987=CARTESIAN_POINT ( 'NONE',  ( -10.20110288159999890, -80.00000000000000000, 41.00000000000000000 ) ) ;
#6988=CARTESIAN_POINT ( 'NONE',  ( -21.85457041760000152, -74.50000000000000000, -32.66023292159999869 ) ) ;
#6990=DIRECTION ( 'NONE',  ( 0.000000000000000000, 1.000000000000000000, 0.000000000000000000 ) ) ;
#6991=CARTESIAN_POINT ( 'NONE',  ( -7.486742987080038603, -73.99989313545945890, 38.95798903407855107 ) ) ;
#6992=CARTESIAN_POINT ( 'NONE',  ( -18.28420043339999879, -18.85622860559999836, 12.72554403070000184 ) ) ;
#6996=CARTESIAN_POINT ( 'NONE',  ( 1.353583911619999998E-12, -74.50000000000000000, 1.342925770590000058E-12 ) ) ;
#6997=CARTESIAN_POINT ( 'NONE',  ( 8.776868765820001528, -35.24001315249999777, -20.49278548850000092 ) ) ;
#6999=CYLINDRICAL_SURFACE ( 'NONE', #13505, 4.749999999999999112 ) ;
#7000=CARTESIAN_POINT ( 'NONE',  ( 46.91789432950000105, -79.86049234800000818, -2.756977921009999832 ) ) ;
#7002=CARTESIAN_POINT ( 'NONE',  ( 19.49544348199999888, -35.50000000000000000, -8.986258402430001624 ) ) ;
#7004=ORIENTED_EDGE ( 'NONE', *, *, #19062, .F. ) ;
#7005=CARTESIAN_POINT ( 'NONE',  ( 46.84518809242615589, -73.94545411799823853, -2.389775450614370911 ) ) ;
#7007=B_SPLINE_CURVE_WITH_KNOTS ( 'NONE', 5,
 ( #10977, #13329, #13482, #15813, #4607, #24725, #22236, #22390, #2436, #13635, #18012, #22543 ),
 .UNSPECIFIED., .F., .F.,
 ( 6, 3, 3, 6 ),
 ( 112.4516932879999871, 115.4092999559999981, 122.7593676410000114, 122.9563471670000041 ),
 .UNSPECIFIED. ) ;
#7008=DIRECTION ( 'NONE',  ( 0.000000000000000000, 1.000000000000000000, 0.000000000000000000 ) ) ;
#7014=B_SPLINE_CURVE_WITH_KNOTS ( 'NONE', 5,
 ( #19735, #252, #7082, #13617, #688, #11417 ),
 .UNSPECIFIED., .F., .F.,
 ( 6, 6 ),
 ( -4.007730545210000273, -3.491867373409999864 ),
 .UNSPECIFIED. ) ;
#7015=DIRECTION ( 'NONE',  ( -0.7071067811865470176, 0.000000000000000000, -0.7071067811865480168 ) ) ;
#7017=CARTESIAN_POINT ( 'NONE',  ( 27.49607050420000220, -67.46050995630001523, 1.934818144049999855 ) ) ;
#7018=CARTESIAN_POINT ( 'NONE',  ( 21.61406585437034522, -37.81672230097021981, -8.081625354649236925 ) ) ;
#7022=CARTESIAN_POINT ( 'NONE',  ( 40.70731707320000226, -74.50000000000000000, 7.215414233289999757 ) ) ;
#7023=ORIENTED_EDGE ( 'NONE', *, *, #25738, .T. ) ;
#7028=CARTESIAN_POINT ( 'NONE',  ( -3.252988965690000178, -74.00000000000000000, -30.32986301179999700 ) ) ;
#7033=CARTESIAN_POINT ( 'NONE',  ( -20.45998242170000125, -52.56313962710000709, 14.78974999389999923 ) ) ;
#7034=CARTESIAN_POINT ( 'NONE',  ( 25.93996424029923986, -74.31568735978206064, -29.40961401139750109 ) ) ;
#7037=CARTESIAN_POINT ( 'NONE',  ( 27.31181567105563346, -69.82812541820754859, 0.5419601338490444009 ) ) ;
#7040=CARTESIAN_POINT ( 'NONE',  ( 10.16215846479999918, -36.06062539180000215, -21.41592806629999757 ) ) ;
#7043=VERTEX_POINT ( 'NONE', #12050 ) ;
#7045=CARTESIAN_POINT ( 'NONE',  ( 7.261004788010000155, -74.03378462380000258, 40.00100507770000036 ) ) ;
#7047=AXIS2_PLACEMENT_3D ( 'NONE', #11448, #17592, #15829 ) ;
#7049=CARTESIAN_POINT ( 'NONE',  ( 23.53415771673985191, -19.48509740633723908, 1.431415487266915365 ) ) ;
#7051=CARTESIAN_POINT ( 'NONE',  ( -3.562216348787903275, -80.34292033684900503, 46.31451622703009718 ) ) ;
#7053=AXIS2_PLACEMENT_3D ( 'NONE', #17869, #28634, #17573 ) ;
#7054=CARTESIAN_POINT ( 'NONE',  ( 8.310288928540000342, -37.22172731869999751, -21.60320471790000241 ) ) ;
#7059=DIRECTION ( 'NONE',  ( 0.000000000000000000, 1.000000000000000000, 0.000000000000000000 ) ) ;
#7061=CARTESIAN_POINT ( 'NONE',  ( -0.8753677514297800721, -19.46426558493637060, -22.01818526256528230 ) ) ;
#7064=CARTESIAN_POINT ( 'NONE',  ( -13.46276276179999876, -19.49999999970000175, 20.39865906480000035 ) ) ;
#7066=ADVANCED_FACE ( 'NONE', ( #4124 ), #2745, .F. ) ;
#7067=LINE ( 'NONE', #24833, #23065 ) ;
#7068=CARTESIAN_POINT ( 'NONE',  ( -12.06432294940000105, -66.82248673960000929, -24.54885029159999732 ) ) ;
#7073=EDGE_LOOP ( 'NONE', ( #12750, #16646, #4920, #19700 ) ) ;
#7075=CARTESIAN_POINT ( 'NONE',  ( 36.37213528550000774, -74.83007510990000810, -14.84647098600000170 ) ) ;
#7076=CARTESIAN_POINT ( 'NONE',  ( -9.356041104380000917, -74.00000000000000000, -37.60355029590000697 ) ) ;
#7080=CARTESIAN_POINT ( 'NONE',  ( -11.77384491379999965, -59.03025262839999954, 20.31645086680000389 ) ) ;
#7081=DIRECTION ( 'NONE',  ( 0.000000000000000000, -1.000000000000000000, 0.000000000000000000 ) ) ;
#7082=CARTESIAN_POINT ( 'NONE',  ( 20.21912291310000143, -36.00000000000000000, -9.726844800120000301 ) ) ;
#7083=CARTESIAN_POINT ( 'NONE',  ( 18.93809058890547448, -18.60284036879449943, 10.27270654917301762 ) ) ;
#7084=CARTESIAN_POINT ( 'NONE',  ( -11.90443957499999961, -64.24504445130001784, -23.68393584109999850 ) ) ;
#7087=CARTESIAN_POINT ( 'NONE',  ( -7.256994698139999755, -74.37142462010000088, -40.28432270869999599 ) ) ;
#7089=VERTEX_POINT ( 'NONE', #8344 ) ;
#7093=EDGE_CURVE ( 'NONE', #25766, #4968, #25980, .T. ) ;
#7094=CARTESIAN_POINT ( 'NONE',  ( 20.94731949980000252, -52.62618816489948159, 10.41165191589998962 ) ) ;
#7097=CARTESIAN_POINT ( 'NONE',  ( -7.239203719582017804, -74.26034152684405854, -40.39659210438060200 ) ) ;
#7098=EDGE_CURVE ( 'NONE', #25224, #20206, #19029, .T. ) ;
#7099=CARTESIAN_POINT ( 'NONE',  ( 19.35838836099999938, -19.15810970359999743, 10.50069124240000029 ) ) ;
#7100=CARTESIAN_POINT ( 'NONE',  ( -21.54806777370000148, -66.92971392940000896, 14.85312681689999970 ) ) ;
#7104=PLANE ( 'NONE',  #3235 ) ;
#7105=CARTESIAN_POINT ( 'NONE',  ( 26.80851110240000068, -72.43053626620000784, -11.12358378779999946 ) ) ;
#7107=CARTESIAN_POINT ( 'NONE',  ( 21.05437574795876188, -19.47731532787699038, 9.460113418286871578 ) ) ;
#7109=EDGE_LOOP ( 'NONE', ( #15317, #431, #4580, #26345 ) ) ;
#7113=CIRCLE ( 'NONE', #23829, 28.68388914670000034 ) ;
#7114=CARTESIAN_POINT ( 'NONE',  ( -1.776356839399999804E-15, -19.00000000000000000, 0.000000000000000000 ) ) ;
#7115=DIRECTION ( 'NONE',  ( 0.000000000000000000, 1.000000000000000000, 0.000000000000000000 ) ) ;
#7117=ORIENTED_EDGE ( 'NONE', *, *, #17777, .T. ) ;
#7120=CARTESIAN_POINT ( 'NONE',  ( -17.13033212710000086, -72.00000000000000000, 23.49748962700000021 ) ) ;
#7121=CARTESIAN_POINT ( 'NONE',  ( 47.13608539959999888, -74.52720457959999578, -1.647993573179999949 ) ) ;
#7122=VERTEX_POINT ( 'NONE', #2107 ) ;
#7128=EDGE_LOOP ( 'NONE', ( #8787, #8572, #12185, #4360, #23389, #1730 ) ) ;
#7129=EDGE_CURVE ( 'NONE', #15684, #22913, #12262, .T. ) ;
#7130=CARTESIAN_POINT ( 'NONE',  ( 36.34782515470000419, -74.05802478990000282, -14.27927808980000002 ) ) ;
#7132=DIRECTION ( 'NONE',  ( 0.000000000000000000, 1.000000000000000000, 0.000000000000000000 ) ) ;
#7133=CARTESIAN_POINT ( 'NONE',  ( -21.96310081540000070, -74.00000000000000000, -32.01947790320000564 ) ) ;
#7134=ORIENTED_EDGE ( 'NONE', *, *, #7754, .T. ) ;
#7138=CARTESIAN_POINT ( 'NONE',  ( -17.60583313680000472, -18.50000000000000000, 11.52657685249999986 ) ) ;
#7140=FACE_OUTER_BOUND ( 'NONE', #10514, .T. ) ;
#7141=AXIS2_PLACEMENT_3D ( 'NONE', #23647, #10635, #19277 ) ;
#7145=DIRECTION ( 'NONE',  ( -0.000000000000000000, 1.000000000000000000, 0.000000000000000000 ) ) ;
#7146=ORIENTED_EDGE ( 'NONE', *, *, #4159, .T. ) ;
#7147=CARTESIAN_POINT ( 'NONE',  ( 46.43423234700000535, -80.49808279690000745, -3.486565683130000259 ) ) ;
#7148=CARTESIAN_POINT ( 'NONE',  ( -11.65446625000000047, -63.14742133130000923, -22.75868051570000006 ) ) ;
#7150=TOROIDAL_SURFACE ( 'NONE', #23429, 2.500000000000000000, 0.5000000000000000000 ) ;
#7151=CARTESIAN_POINT ( 'NONE',  ( 25.21073747289999645, -68.18737760160000505, -8.386242643919999296 ) ) ;
#7154=CARTESIAN_POINT ( 'NONE',  ( -11.91166822033579464, -71.21053272331209882, -26.23707332927977021 ) ) ;
#7156=CARTESIAN_POINT ( 'NONE',  ( 28.57122076013681422, -72.72581502554379540, 1.952398001462756216 ) ) ;
#7157=LINE ( 'NONE', #20555, #26056 ) ;
#7164=CARTESIAN_POINT ( 'NONE',  ( -16.49390888960000368, -74.50000000000000000, 44.28897684009999836 ) ) ;
#7166=CARTESIAN_POINT ( 'NONE',  ( -10.55247273420000020, -18.86819686409999974, -21.60718219059999967 ) ) ;
#7167=CARTESIAN_POINT ( 'NONE',  ( 21.64462882888506812, -37.86826266693650211, -8.165772047040821491 ) ) ;
#7168=ORIENTED_EDGE ( 'NONE', *, *, #7993, .T. ) ;
#7169=DIRECTION ( 'NONE',  ( 1.000000000000000000, 0.000000000000000000, 0.000000000000000000 ) ) ;
#7172=ORIENTED_EDGE ( 'NONE', *, *, #22557, .T. ) ;
#7173=EDGE_CURVE ( 'NONE', #6525, #16196, #14034, .T. ) ;
#7174=AXIS2_PLACEMENT_3D ( 'NONE', #5946, #26211, #28108 ) ;
#7175=CARTESIAN_POINT ( 'NONE',  ( 20.63161943080000071, -19.46510050319999863, -7.734358783100000245 ) ) ;
#7180=CARTESIAN_POINT ( 'NONE',  ( -19.57536200539999882, -26.03958238319999907, 14.34081999809999886 ) ) ;
#7181=CARTESIAN_POINT ( 'NONE',  ( 43.75000000000000000, -84.50000000000000000, 5.357814579270000097E-15 ) ) ;
#7182=CARTESIAN_POINT ( 'NONE',  ( 31.15598256050000003, -72.92631784149999419, -20.30650074509999925 ) ) ;
#7183=CARTESIAN_POINT ( 'NONE',  ( -14.68358879805363060, -74.18174932740166128, 36.27808831497246445 ) ) ;
#7184=AXIS2_PLACEMENT_3D ( 'NONE', #3379, #8285, #28671 ) ;
#7185=EDGE_CURVE ( 'NONE', #7833, #22866, #27400, .T. ) ;
#7187=AXIS2_PLACEMENT_3D ( 'NONE', #13302, #20011, #8931 ) ;
#7188=EDGE_LOOP ( 'NONE', ( #2172, #12058, #2808, #26898 ) ) ;
#7189=DIRECTION ( 'NONE',  ( 0.000000000000000000, 1.000000000000000000, 0.000000000000000000 ) ) ;
#7191=ORIENTED_EDGE ( 'NONE', *, *, #18544, .F. ) ;
#7193=CARTESIAN_POINT ( 'NONE',  ( 7.250133233359999707, -73.75841684550000821, 39.12193274490000050 ) ) ;
#7194=CARTESIAN_POINT ( 'NONE',  ( 46.63086251900000434, -74.05159139319999895, -3.730496185299999823 ) ) ;
#7195=CARTESIAN_POINT ( 'NONE',  ( 23.52750467767722142, -19.48498740571179866, 1.429708917240688937 ) ) ;
#7196=CARTESIAN_POINT ( 'NONE',  ( 26.98670340789999855, -72.82938977469999031, -9.720255250690000182 ) ) ;
#7198=CARTESIAN_POINT ( 'NONE',  ( 8.201563467870000679, -37.53730314839999949, -21.64399269869999642 ) ) ;
#7199=CARTESIAN_POINT ( 'NONE',  ( 8.697618611485006923, -19.48148083423015109, -19.87404037427484838 ) ) ;
#7200=ORIENTED_EDGE ( 'NONE', *, *, #27497, .T. ) ;
#7202=DIRECTION ( 'NONE',  ( 0.9704142011833034598, 0.000000000000000000, 0.2414462220490750932 ) ) ;
#7203=CARTESIAN_POINT ( 'NONE',  ( 21.53806854011714478, -36.56992522606418561, -6.948750312138934682 ) ) ;
#7204=CARTESIAN_POINT ( 'NONE',  ( -1.681229913738337967, -19.46756325247292807, -22.31722361663701903 ) ) ;
#7206=CARTESIAN_POINT ( 'NONE',  ( -19.92984078955770499, -18.50000000000000000, 15.63765909864717152 ) ) ;
#7209=CARTESIAN_POINT ( 'NONE',  ( 21.72762743471350788, -37.33446486334822367, -8.509936560388821292 ) ) ;
#7210=CIRCLE ( 'NONE', #3922, 0.4999999999999997224 ) ;
#7213=ORIENTED_EDGE ( 'NONE', *, *, #3002, .T. ) ;
#7215=EDGE_CURVE ( 'NONE', #3837, #19973, #23428, .T. ) ;
#7217=AXIS2_PLACEMENT_3D ( 'NONE', #24584, #18173, #4917 ) ;
#7220=FACE_OUTER_BOUND ( 'NONE', #28537, .T. ) ;
#7221=CARTESIAN_POINT ( 'NONE',  ( 20.52569424150000188, -35.38531346950000511, -8.770435587459999738 ) ) ;
#7225=CARTESIAN_POINT ( 'NONE',  ( -0.5335602090290000321, -52.63293862049999916, -23.18581005440000098 ) ) ;
#7226=DIRECTION ( 'NONE',  ( 1.000000000000000000, 0.000000000000000000, 0.000000000000000000 ) ) ;
#7227=EDGE_CURVE ( 'NONE', #24310, #12443, #14797, .T. ) ;
#7230=ORIENTED_EDGE ( 'NONE', *, *, #3758, .T. ) ;
#7233=ORIENTED_EDGE ( 'NONE', *, *, #4873, .F. ) ;
#7237=CIRCLE ( 'NONE', #7704, 0.5000000000000004441 ) ;
#7239=CARTESIAN_POINT ( 'NONE',  ( -7.224488193841309247, -74.42768721721228076, -40.61475266807387641 ) ) ;
#7240=CARTESIAN_POINT ( 'NONE',  ( -14.02382502650000085, -74.01102208230000201, 36.34092783020000184 ) ) ;
#7241=CARTESIAN_POINT ( 'NONE',  ( 11.12357766309999896, -72.43053616469998701, -26.80850844170000258 ) ) ;
#7242=B_SPLINE_CURVE_WITH_KNOTS ( 'NONE', 5,
 ( #22356, #17983, #2116, #10951, #19861, #2400 ),
 .UNSPECIFIED., .F., .F.,
 ( 6, 6 ),
 ( -66.18347591719999912, -36.59856967589999499 ),
 .UNSPECIFIED. ) ;
#7244=ORIENTED_EDGE ( 'NONE', *, *, #25921, .F. ) ;
#7246=CARTESIAN_POINT ( 'NONE',  ( 8.521725336259999395, -22.48306963330000130, -20.31493383569999978 ) ) ;
#7249=CARTESIAN_POINT ( 'NONE',  ( 7.188502612221723709, -73.76099270142834996, -38.70686962976383683 ) ) ;
#7250=EDGE_LOOP ( 'NONE', ( #11774, #9101, #28431, #26460 ) ) ;
#7254=EDGE_CURVE ( 'NONE', #5383, #7122, #17136, .T. ) ;
#7260=ADVANCED_FACE ( 'NONE', ( #9935 ), #812, .F. ) ;
#7261=EDGE_LOOP ( 'NONE', ( #3084, #13307, #23431, #20726, #7023 ) ) ;
#7264=CARTESIAN_POINT ( 'NONE',  ( 46.85181496819999580, -74.07956791590001444, -2.486435421679999980 ) ) ;
#7265=ORIENTED_EDGE ( 'NONE', *, *, #14844, .F. ) ;
#7266=CARTESIAN_POINT ( 'NONE',  ( 7.249694362036529505, -73.91587151478432816, -39.90536558169799974 ) ) ;
#7269=CARTESIAN_POINT ( 'NONE',  ( -2.969720195599999890, -65.80499425489999510, -26.85431770659999984 ) ) ;
#7270=CARTESIAN_POINT ( 'NONE',  ( -14.67079327179999915, -67.87586646439999072, 22.52608794949999904 ) ) ;
#7272=DIRECTION ( 'NONE',  ( 0.9952295494196654602, 0.000000000000000000, -0.09756097560976760563 ) ) ;
#7273=PLANE ( 'NONE',  #22049 ) ;
#7274=CARTESIAN_POINT ( 'NONE',  ( 26.23106671699999737, -64.35840483370000698, 1.472051099300000221 ) ) ;
#7275=LINE ( 'NONE', #16142, #26446 ) ;
#7276=ORIENTED_EDGE ( 'NONE', *, *, #2963, .T. ) ;
#7277=CARTESIAN_POINT ( 'NONE',  ( -0.5256381167571819724, -45.99935878244429688, -22.95428131896234092 ) ) ;
#7279=CARTESIAN_POINT ( 'NONE',  ( 36.62847051954670263, -74.18064277860715094, -14.32357927737881553 ) ) ;
#7280=ORIENTED_EDGE ( 'NONE', *, *, #4882, .T. ) ;
#7282=CARTESIAN_POINT ( 'NONE',  ( 21.33526310999999964, -62.97603269449999885, 11.59349340770000047 ) ) ;
#7283=CARTESIAN_POINT ( 'NONE',  ( 8.988996102879999839, -34.66800400750000222, -19.43643858049999906 ) ) ;
#7286=ORIENTED_EDGE ( 'NONE', *, *, #17324, .T. ) ;
#7287=CARTESIAN_POINT ( 'NONE',  ( 45.89652018349999452, -80.18584073460000639, -4.323400012419999605 ) ) ;
#7290=CARTESIAN_POINT ( 'NONE',  ( -12.21854180399999912, -18.61865655080000082, 18.67250271059999989 ) ) ;
#7291=CARTESIAN_POINT ( 'NONE',  ( -12.69354674090000046, -63.63799337809999912, -20.95011387349999765 ) ) ;
#7292=CARTESIAN_POINT ( 'NONE',  ( 26.22359489970000013, -71.21989987509999764, -9.687831617969999698 ) ) ;
#7295=ORIENTED_EDGE ( 'NONE', *, *, #1602, .T. ) ;
#7301=VERTEX_POINT ( 'NONE', #6273 ) ;
#7302=DIRECTION ( 'NONE',  ( 0.000000000000000000, -1.000000000000000000, 0.000000000000000000 ) ) ;
#7303=CARTESIAN_POINT ( 'NONE',  ( 21.30133042140352373, -35.02996653984773445, -7.508028375805006149 ) ) ;
#7305=CARTESIAN_POINT ( 'NONE',  ( 23.08854236903368218, -49.87586154376155179, -0.5737623537064138191 ) ) ;
#7308=CARTESIAN_POINT ( 'NONE',  ( 9.617235035043430358, -59.75166407288456583, -23.68427203224058530 ) ) ;
#7310=CARTESIAN_POINT ( 'NONE',  ( 0.000000000000000000, -89.00000000000000000, 0.000000000000000000 ) ) ;
#7311=CARTESIAN_POINT ( 'NONE',  ( -20.76808354211960150, -63.08717869840388204, 12.74414642584173407 ) ) ;
#7313=EDGE_LOOP ( 'NONE', ( #5373, #6644, #8345, #22424, #14308 ) ) ;
#7314=CARTESIAN_POINT ( 'NONE',  ( 20.51869861192218281, -18.95847997710646027, -7.692027150944580782 ) ) ;
#7316=DIRECTION ( 'NONE',  ( 1.000000000000000000, 0.000000000000000000, 0.000000000000000000 ) ) ;
#7317=EDGE_LOOP ( 'NONE', ( #785, #13622, #14146, #18675 ) ) ;
#7321=DIRECTION ( 'NONE',  ( -0.7071067811865474617, 0.000000000000000000, -0.7071067811865474617 ) ) ;
#7325=EDGE_CURVE ( 'NONE', #2162, #12777, #12955, .T. ) ;
#7326=B_SPLINE_CURVE_WITH_KNOTS ( 'NONE', 3,
 ( #26580, #17408, #2401, #24100, #11259, #19724 ),
 .UNSPECIFIED., .F., .F.,
 ( 4, 2, 4 ),
 ( 0.000000000000000000, 0.5000000000000000000, 1.000000000000000000 ),
 .UNSPECIFIED. ) ;
#7327=CARTESIAN_POINT ( 'NONE',  ( 27.29208946090000154, -66.82248673960000929, 1.826414992130000137 ) ) ;
#7328=CARTESIAN_POINT ( 'NONE',  ( -10.72007167189999777, -18.61782383720000311, 18.81070191750000120 ) ) ;
#7331=CARTESIAN_POINT ( 'NONE',  ( -19.35716652280000005, -18.50000000000000000, 15.34467299940000018 ) ) ;
#7332=DIRECTION ( 'NONE',  ( 0.000000000000000000, 1.000000000000000000, 0.000000000000000000 ) ) ;
#7335=CARTESIAN_POINT ( 'NONE',  ( 7.509443212019999869, -18.50000000000000000, -19.64862788269999783 ) ) ;
#7336=B_SPLINE_SURFACE_WITH_KNOTS ( 'NONE', 5, 5, ( 
 ( #13026, #17425, #28487, #21507, #19455, #1989 ),
 ( #14790, #1568, #10409, #15204, #21939, #24118 ),
 ( #13180, #4154, #10831, #28627, #28202, #8659 ),
 ( #1423, #8235, #15350, #14928, #10267, #6045 ),
 ( #19181, #5908, #23833, #3873, #21653, #5031 ),
 ( #548, #22089, #8804, #4891, #26900, #13472 ) ),
 .UNSPECIFIED., .F., .F., .F.,
 ( 6, 6 ),
 ( 6, 6 ),
 ( 7.598610046719999289, 9.882009902280000091 ),
 ( 0.000000000000000000, 0.3214525575110000477 ),
 .UNSPECIFIED. ) ;
#7337=FACE_OUTER_BOUND ( 'NONE', #28473, .T. ) ;
#7341=CARTESIAN_POINT ( 'NONE',  ( 9.235022047270001977, -35.95171755970000049, -20.04752849569999995 ) ) ;
#7342=CARTESIAN_POINT ( 'NONE',  ( 46.25000000000000000, -74.00000000000000000, -4.582575694960000057 ) ) ;
#7345=CARTESIAN_POINT ( 'NONE',  ( -40.30949744628526332, -74.19510049693010956, 7.243395527605200890 ) ) ;
#7347=LINE ( 'NONE', #22502, #6077 ) ;
#7348=CARTESIAN_POINT ( 'NONE',  ( -12.41213674656621890, -19.47453264959771246, 19.24115019510791669 ) ) ;
#7350=ORIENTED_EDGE ( 'NONE', *, *, #20855, .T. ) ;
#7351=CARTESIAN_POINT ( 'NONE',  ( -2.504890583376165658, -19.48260761093995086, -23.29076242136417108 ) ) ;
#7353=CARTESIAN_POINT ( 'NONE',  ( -1.164060375740000097, -45.99732788909999925, -23.00302772650000094 ) ) ;
#7358=CARTESIAN_POINT ( 'NONE',  ( 21.71814693700000021, -44.93138464870000348, -7.554088719500000160 ) ) ;
#7360=DIRECTION ( 'NONE',  ( 0.000000000000000000, 1.000000000000000000, 0.000000000000000000 ) ) ;
#7361=ORIENTED_EDGE ( 'NONE', *, *, #9993, .F. ) ;
#7367=CARTESIAN_POINT ( 'NONE',  ( 19.96643108339999984, -35.14332902089999777, -8.964388679729999865 ) ) ;
#7368=CARTESIAN_POINT ( 'NONE',  ( 7.220129148630540783, -73.62781383915867650, 39.34253424956806100 ) ) ;
#7369=CIRCLE ( 'NONE', #12904, 3.750000000000000000 ) ;
#7370=CARTESIAN_POINT ( 'NONE',  ( 8.677144207910000517, -37.95796631070000160, -21.92880662259999980 ) ) ;
#7371=CARTESIAN_POINT ( 'NONE',  ( 21.61812661869999985, -36.72157724490000419, -8.702650991499998767 ) ) ;
#7373=DIRECTION ( 'NONE',  ( 0.000000000000000000, 1.000000000000000000, 0.000000000000000000 ) ) ;
#7374=ORIENTED_EDGE ( 'NONE', *, *, #8540, .T. ) ;
#7376=AXIS2_PLACEMENT_3D ( 'NONE', #19099, #1340, #27987 ) ;
#7377=DIRECTION ( 'NONE',  ( 0.000000000000000000, 1.000000000000000000, 0.000000000000000000 ) ) ;
#7378=ORIENTED_EDGE ( 'NONE', *, *, #191, .F. ) ;
#7384=EDGE_CURVE ( 'NONE', #13154, #11916, #15024, .T. ) ;
#7386=CARTESIAN_POINT ( 'NONE',  ( -7.220129148633156468, -73.62781383918019174, -39.34253424959684509 ) ) ;
#7388=CARTESIAN_POINT ( 'NONE',  ( -14.93121066289999987, -74.50000000000000000, 36.29905574720000061 ) ) ;
#7391=VERTEX_POINT ( 'NONE', #15591 ) ;
#7392=CIRCLE ( 'NONE', #24124, 3.000000000000000888 ) ;
#7393=CARTESIAN_POINT ( 'NONE',  ( -12.05351144729999824, -70.58794772379999927, -25.57911838539999749 ) ) ;
#7394=CARTESIAN_POINT ( 'NONE',  ( 8.982220866290001382, -19.48263932869999948, -19.39107707569999661 ) ) ;
#7396=EDGE_CURVE ( 'NONE', #28554, #22934, #16820, .T. ) ;
#7397=DIRECTION ( 'NONE',  ( 1.000000000000000000, 0.000000000000000000, 0.000000000000000000 ) ) ;
#7398=CARTESIAN_POINT ( 'NONE',  ( -39.12175830409999122, -73.75838856979999036, -7.250123850439999629 ) ) ;
#7402=DIRECTION ( 'NONE',  ( 0.000000000000000000, 1.000000000000000000, 0.000000000000000000 ) ) ;
#7406=AXIS2_PLACEMENT_3D ( 'NONE', #22240, #9116, #2441 ) ;
#7408=AXIS2_PLACEMENT_3D ( 'NONE', #23388, #3295, #20927 ) ;
#7410=CARTESIAN_POINT ( 'NONE',  ( 9.393614001710000494, -38.00000000000000000, -22.97877290430000130 ) ) ;
#7411=CARTESIAN_POINT ( 'NONE',  ( 11.21184057910000043, -36.00000000000000000, -22.05994369109999909 ) ) ;
#7412=VERTEX_POINT ( 'NONE', #11207 ) ;
#7413=CARTESIAN_POINT ( 'NONE',  ( 7.216929735086898390, -73.61493928631104211, -39.30828467231233958 ) ) ;
#7414=CARTESIAN_POINT ( 'NONE',  ( -11.76694263665041262, -63.20675823528085147, 21.38603125774777425 ) ) ;
#7417=CARTESIAN_POINT ( 'NONE',  ( -2.606614045719999773, -69.52108470319998901, -27.18390150700000163 ) ) ;
#7418=ADVANCED_FACE ( 'NONE', ( #13709 ), #4967, .F. ) ;
#7419=CARTESIAN_POINT ( 'NONE',  ( -14.56435550020000136, -68.97522950350000315, 22.81609951000000081 ) ) ;
#7421=EDGE_CURVE ( 'NONE', #12917, #18911, #3264, .T. ) ;
#7422=DIRECTION ( 'NONE',  ( 0.000000000000000000, 1.000000000000000000, 0.000000000000000000 ) ) ;
#7424=CARTESIAN_POINT ( 'NONE',  ( 25.16979986939999847, -65.00127508749999095, 0.1507740601240000200 ) ) ;
#7425=CARTESIAN_POINT ( 'NONE',  ( 19.49544348199999888, -35.50000000000000000, -8.986258402430001624 ) ) ;
#7426=EDGE_LOOP ( 'NONE', ( #26743, #12938, #11192, #1031 ) ) ;
#7427=AXIS2_PLACEMENT_3D ( 'NONE', #53, #15608, #13422 ) ;
#7428=FACE_OUTER_BOUND ( 'NONE', #23993, .T. ) ;
#7429=EDGE_CURVE ( 'NONE', #15559, #9997, #3232, .T. ) ;
#7430=CARTESIAN_POINT ( 'NONE',  ( -7.405876894974190883, -73.99964090891569413, 39.17806186240734689 ) ) ;
#7431=CARTESIAN_POINT ( 'NONE',  ( 36.74680559931929480, -74.42334987367621579, -14.56713157595660668 ) ) ;
#7432=ORIENTED_EDGE ( 'NONE', *, *, #11997, .F. ) ;
#7439=CARTESIAN_POINT ( 'NONE',  ( 21.71348175089999799, -64.04267428580000399, 11.73101879090000033 ) ) ;
#7440=CARTESIAN_POINT ( 'NONE',  ( 8.965452453730000215, -34.82094141099999973, -19.92119506740000290 ) ) ;
#7442=CARTESIAN_POINT ( 'NONE',  ( 36.74383121569999844, -74.66666669110000498, -14.69280905019999928 ) ) ;
#7444=CARTESIAN_POINT ( 'NONE',  ( 47.15414012749999983, -79.55218225590000714, -1.873848225679999757 ) ) ;
#7447=CARTESIAN_POINT ( 'NONE',  ( -11.41034487649999996, -19.46528075099999811, 19.03911974529999895 ) ) ;
#7448=CARTESIAN_POINT ( 'NONE',  ( -12.45267061699999900, -63.62177041899999352, -21.09031584749999766 ) ) ;
#7450=CARTESIAN_POINT ( 'NONE',  ( 37.09477810047854973, -79.93445530391007026, -14.10616743337098455 ) ) ;
#7451=CARTESIAN_POINT ( 'NONE',  ( 25.33520104860000188, -65.80271452349998640, -10.35056844610000049 ) ) ;
#7454=DIRECTION ( 'NONE',  ( 1.000000000000000000, 0.000000000000000000, 0.000000000000000000 ) ) ;
#7456=CARTESIAN_POINT ( 'NONE',  ( -13.39932972679999956, -27.00850923819999849, 20.26025068540000262 ) ) ;
#7458=EDGE_LOOP ( 'NONE', ( #17312, #21391, #23832, #6561 ) ) ;
#7462=ORIENTED_EDGE ( 'NONE', *, *, #4641, .T. ) ;
#7463=CARTESIAN_POINT ( 'NONE',  ( 39.64169929330000031, -73.82505178019999903, 7.260629316899999353 ) ) ;
#7464=CARTESIAN_POINT ( 'NONE',  ( -10.50201809968876354, -19.47159322330747599, -20.11218106846735765 ) ) ;
#7465=CARTESIAN_POINT ( 'NONE',  ( 7.105427357599999217E-15, -74.50000000000000000, 3.552713678799999608E-15 ) ) ;
#7467=CARTESIAN_POINT ( 'NONE',  ( 46.25000000000000000, -80.00000000000000000, -4.582575694960000057 ) ) ;
#7468=ORIENTED_EDGE ( 'NONE', *, *, #25001, .F. ) ;
#7469=EDGE_CURVE ( 'NONE', #8141, #2786, #9712, .T. ) ;
#7470=CARTESIAN_POINT ( 'NONE',  ( 4.882943008269999509E-15, -74.50000000000000000, -40.00000000000000000 ) ) ;
#7473=ORIENTED_EDGE ( 'NONE', *, *, #1529, .T. ) ;
#7478=EDGE_CURVE ( 'NONE', #27002, #16095, #10184, .T. ) ;
#7482=CARTESIAN_POINT ( 'NONE',  ( 27.75394116159999669, -74.50000000000000000, -27.75394116159999669 ) ) ;
#7483=CARTESIAN_POINT ( 'NONE',  ( -14.87486851012731393, -74.34009834986436260, 36.29443389971319078 ) ) ;
#7485=TOROIDAL_SURFACE ( 'NONE', #11142, 7.750000000000000000, 0.5000000000000000000 ) ;
#7486=ORIENTED_EDGE ( 'NONE', *, *, #19652, .T. ) ;
#7487=CARTESIAN_POINT ( 'NONE',  ( 9.885503723209998483, -36.00000000000000000, -20.33566493420000043 ) ) ;
#7488=FACE_BOUND ( 'NONE', #6490, .T. ) ;
#7489=CARTESIAN_POINT ( 'NONE',  ( 20.76816312569999923, -36.14487676950000150, -8.994776261610001100 ) ) ;
#7491=ORIENTED_EDGE ( 'NONE', *, *, #2333, .T. ) ;
#7492=DIRECTION ( 'NONE',  ( 0.000000000000000000, -1.000000000000000000, 0.000000000000000000 ) ) ;
#7494=CARTESIAN_POINT ( 'NONE',  ( -20.89470113654807193, -64.89165741046112146, 14.23290170999320736 ) ) ;
#7497=CARTESIAN_POINT ( 'NONE',  ( -20.45998242170000125, -45.73899999920000425, 14.78974999389999923 ) ) ;
#7502=EDGE_CURVE ( 'NONE', #20928, #22701, #19476, .T. ) ;
#7504=AXIS2_PLACEMENT_3D ( 'NONE', #6996, #15859, #27103 ) ;
#7505=CARTESIAN_POINT ( 'NONE',  ( 23.98359025029999714, -18.62222165789999906, 1.917870889060000028 ) ) ;
#7506=DIRECTION ( 'NONE',  ( 0.2414462220490753985, 0.000000000000000000, 0.9704142011833032377 ) ) ;
#7510=CARTESIAN_POINT ( 'NONE',  ( -2.584367914690000045, -39.30675845289999870, -24.46232226030000234 ) ) ;
#7512=EDGE_CURVE ( 'NONE', #12727, #5555, #5549, .T. ) ;
#7513=DIRECTION ( 'NONE',  ( 0.8077658500622459936, 0.000000000000000000, -0.5895034617991798953 ) ) ;
#7516=CARTESIAN_POINT ( 'NONE',  ( 21.79505839750000007, -40.73328259210000368, -8.465915579709999861 ) ) ;
#7517=DIRECTION ( 'NONE',  ( 0.000000000000000000, -1.000000000000000000, 0.000000000000000000 ) ) ;
#7518=FACE_OUTER_BOUND ( 'NONE', #10158, .T. ) ;
#7526=CARTESIAN_POINT ( 'NONE',  ( 40.00000000000000000, -69.00000000000000000, 5.786765616290000531E-15 ) ) ;
#7527=CARTESIAN_POINT ( 'NONE',  ( 21.21808932789999957, -34.59820509829999935, -7.670972970090000231 ) ) ;
#7528=CARTESIAN_POINT ( 'NONE',  ( 23.29172356445612024, -59.74599976188999761, 10.44929617870533534 ) ) ;
#7530=DIRECTION ( 'NONE',  ( 0.000000000000000000, 1.000000000000000000, 0.000000000000000000 ) ) ;
#7531=CARTESIAN_POINT ( 'NONE',  ( 21.84310887519999866, -37.95394735069999825, -8.556787659450000305 ) ) ;
#7534=ORIENTED_EDGE ( 'NONE', *, *, #19822, .T. ) ;
#7535=FILL_AREA_STYLE ('',( #18595 ) ) ;
#7537=VERTEX_POINT ( 'NONE', #25507 ) ;
#7541=EDGE_CURVE ( 'NONE', #23580, #7650, #4574, .T. ) ;
#7544=CARTESIAN_POINT ( 'NONE',  ( -12.05063396398067965, -64.89165752751554805, -22.22490323539291524 ) ) ;
#7545=AXIS2_PLACEMENT_3D ( 'NONE', #24391, #8777, #1818 ) ;
#7546=CARTESIAN_POINT ( 'NONE',  ( -7.244162156032069255, -74.18137224046682832, -40.29089741864455476 ) ) ;
#7547=AXIS2_PLACEMENT_3D ( 'NONE', #4511, #2340, #4662 ) ;
#7549=DIRECTION ( 'NONE',  ( 0.7071067811865474617, 0.000000000000000000, 0.7071067811865474617 ) ) ;
#7552=CYLINDRICAL_SURFACE ( 'NONE', #17153, 10.00000000000000000 ) ;
#7554=CARTESIAN_POINT ( 'NONE',  ( -2.488381629358669134, -57.43018252028311821, -24.62423963244554059 ) ) ;
#7555=CARTESIAN_POINT ( 'NONE',  ( 19.50599165336712915, -19.46426558497125470, 10.25100193001445170 ) ) ;
#7556=ORIENTED_EDGE ( 'NONE', *, *, #19652, .F. ) ;
#7558=EDGE_CURVE ( 'NONE', #21778, #4525, #1501, .T. ) ;
#7559=CARTESIAN_POINT ( 'NONE',  ( -1.980680968570000200, -57.88555731719999642, -23.85230741780000230 ) ) ;
#7561=DIRECTION ( 'NONE',  ( 6.106226635439999831E-16, 0.000000000000000000, 1.000000000000000000 ) ) ;
#7564=ORIENTED_EDGE ( 'NONE', *, *, #10088, .T. ) ;
#7565=ORIENTED_EDGE ( 'NONE', *, *, #12031, .F. ) ;
#7567=CARTESIAN_POINT ( 'NONE',  ( 21.94388422209999945, -37.05206035260000164, -9.022696796810000919 ) ) ;
#7568=CARTESIAN_POINT ( 'NONE',  ( 47.25000000000000000, -75.00000000000000000, -13.75000000000000000 ) ) ;
#7569=EDGE_LOOP ( 'NONE', ( #25031, #12256, #27068, #5519 ) ) ;
#7570=CARTESIAN_POINT ( 'NONE',  ( 7.249551406111377716, -74.03750509262690116, -40.08893529128285138 ) ) ;
#7571=CARTESIAN_POINT ( 'NONE',  ( -10.61287167059999881, -19.46510050329999686, 19.30934957549999709 ) ) ;
#7572=VERTEX_POINT ( 'NONE', #8563 ) ;
#7573=CARTESIAN_POINT ( 'NONE',  ( 21.70991749090000056, -40.75155002500000023, -6.890073352940000007 ) ) ;
#7574=CARTESIAN_POINT ( 'NONE',  ( -2.647831762760000096, -64.47176800949999631, -25.90231288840000090 ) ) ;
#7576=ORIENTED_EDGE ( 'NONE', *, *, #331, .F. ) ;
#7577=CARTESIAN_POINT ( 'NONE',  ( 36.29989756469999662, -74.04896632250000721, -14.30540807509999901 ) ) ;
#7579=CARTESIAN_POINT ( 'NONE',  ( 25.43931335289999751, -61.67863912290000172, 1.361017498729999886 ) ) ;
#7580=CARTESIAN_POINT ( 'NONE',  ( 36.22844186549999534, -74.00000000000000000, -13.75000000000000000 ) ) ;
#7582=CARTESIAN_POINT ( 'NONE',  ( -0.5856137342820000313, -19.46510053389999939, -22.02591827759999887 ) ) ;
#7584=CARTESIAN_POINT ( 'NONE',  ( -7.285364666873626938, -73.99996940651281818, 39.64792326107047415 ) ) ;
#7585=CARTESIAN_POINT ( 'NONE',  ( 36.70128390686866737, -74.28717797990978511, -14.45333729646541698 ) ) ;
#7587=CARTESIAN_POINT ( 'NONE',  ( -13.64864847579999996, -18.50000000000000000, 18.87892408420000123 ) ) ;
#7591=FACE_OUTER_BOUND ( 'NONE', #22899, .T. ) ;
#7594=CARTESIAN_POINT ( 'NONE',  ( 25.86648679569999842, -67.35799111629999913, -10.65566745589999975 ) ) ;
#7599=DIRECTION ( 'NONE',  ( 0.000000000000000000, 1.000000000000000000, 0.000000000000000000 ) ) ;
#7600=EDGE_LOOP ( 'NONE', ( #11237, #10210, #24794, #19867 ) ) ;
#7602=CARTESIAN_POINT ( 'NONE',  ( -12.95621714570000016, -27.03158182010000132, 19.72987597090000023 ) ) ;
#7604=EDGE_CURVE ( 'NONE', #26673, #12661, #3915, .T. ) ;
#7605=VERTEX_POINT ( 'NONE', #15104 ) ;
#7606=CIRCLE ( 'NONE', #24308, 0.5000000000000027756 ) ;
#7607=CARTESIAN_POINT ( 'NONE',  ( 6.483702463809999749E-15, -84.50000000000000000, -40.00000000000000000 ) ) ;
#7608=EDGE_CURVE ( 'NONE', #9894, #7605, #21814, .T. ) ;
#7609=CARTESIAN_POINT ( 'NONE',  ( 40.70731707320000226, -74.50000000000000000, 7.215414233289999757 ) ) ;
#7613=CARTESIAN_POINT ( 'NONE',  ( 46.96553338548562095, -79.70204288960100314, -2.546098179092394886 ) ) ;
#7614=ORIENTED_EDGE ( 'NONE', *, *, #13110, .T. ) ;
#7617=DIRECTION ( 'NONE',  ( 0.09756097560976655092, 0.000000000000000000, -0.9952295494196655712 ) ) ;
#7621=CARTESIAN_POINT ( 'NONE',  ( -0.7490697104619999935, -79.69325168709998763, 47.25079635160000180 ) ) ;
#7622=CARTESIAN_POINT ( 'NONE',  ( 22.35420140607709527, -19.18584080450712648, 9.881343207706809295 ) ) ;
#7624=DIRECTION ( 'NONE',  ( 1.000000000000000000, 0.000000000000000000, 0.000000000000000000 ) ) ;
#7626=CARTESIAN_POINT ( 'NONE',  ( -19.88518777170000007, -26.02764329579999725, 14.47991441779999988 ) ) ;
#7629=CARTESIAN_POINT ( 'NONE',  ( 22.76484527320000240, -58.91972909429999561, -9.111819319440000342 ) ) ;
#7630=CIRCLE ( 'NONE', #23871, 0.5000000000000004441 ) ;
#7631=EDGE_CURVE ( 'NONE', #21711, #17492, #26831, .T. ) ;
#7633=LINE ( 'NONE', #16350, #1207 ) ;
#7634=CONICAL_SURFACE ( 'NONE', #2500, 21.99999999999999645, 0.03490658503990158590 ) ;
#7635=CARTESIAN_POINT ( 'NONE',  ( 21.22368013470000037, -36.46178979729999980, -8.714942773269999776 ) ) ;
#7638=CARTESIAN_POINT ( 'NONE',  ( 47.19280574540000117, -74.66665734379999719, -1.149945984370000174 ) ) ;
#7641=CYLINDRICAL_SURFACE ( 'NONE', #22692, 7.250000000000004441 ) ;
#7642=CARTESIAN_POINT ( 'NONE',  ( 7.843434090700001526, -40.74566548840000024, -21.60733108830000049 ) ) ;
#7646=DIRECTION ( 'NONE',  ( 0.000000000000000000, 1.000000000000000000, 0.000000000000000000 ) ) ;
#7648=CARTESIAN_POINT ( 'NONE',  ( -13.39873670630472446, -19.49660132354000197, 20.21730935084874048 ) ) ;
#7650=VERTEX_POINT ( 'NONE', #24454 ) ;
#7651=CARTESIAN_POINT ( 'NONE',  ( 19.47999862770000234, -18.50000000000000000, -7.780772602109999880 ) ) ;
#7655=AXIS2_PLACEMENT_3D ( 'NONE', #15560, #8425, #21991 ) ;
#7656=DIRECTION ( 'NONE',  ( 0.000000000000000000, -1.000000000000000000, 0.000000000000000000 ) ) ;
#7659=CARTESIAN_POINT ( 'NONE',  ( 21.46720264400000033, -36.56420440560000173, -7.810721578089999895 ) ) ;
#7660=DIRECTION ( 'NONE',  ( 1.000000000000000000, 0.000000000000000000, 0.000000000000000000 ) ) ;
#7662=ORIENTED_EDGE ( 'NONE', *, *, #11222, .F. ) ;
#7663=CARTESIAN_POINT ( 'NONE',  ( -32.73892505050000068, -74.50000000299999670, -22.13232332930000013 ) ) ;
#7664=CARTESIAN_POINT ( 'NONE',  ( 47.16620867047740973, -74.55684918557169283, -1.099331675085676086 ) ) ;
#7670=CARTESIAN_POINT ( 'NONE',  ( 21.32186554389999600, -35.14390151279999230, -7.472189324920000431 ) ) ;
#7671=CARTESIAN_POINT ( 'NONE',  ( 7.242474372560842255, -73.77182148714507548, 39.65872146204866056 ) ) ;
#7672=CARTESIAN_POINT ( 'NONE',  ( -14.19074604640000103, -64.47177095450000195, 21.84081649480000209 ) ) ;
#7674=DIRECTION ( 'NONE',  ( 0.000000000000000000, 1.000000000000000000, 0.000000000000000000 ) ) ;
#7678=CARTESIAN_POINT ( 'NONE',  ( -0.9701750278467260458, -66.11532767438119151, -25.60589888208034992 ) ) ;
#7679=CARTESIAN_POINT ( 'NONE',  ( -12.30070879700853581, -60.59571579695742827, -20.16720528227978804 ) ) ;
#7680=ORIENTED_EDGE ( 'NONE', *, *, #17536, .F. ) ;
#7681=FACE_OUTER_BOUND ( 'NONE', #4695, .T. ) ;
#7682=B_SPLINE_CURVE_WITH_KNOTS ( 'NONE', 5,
 ( #9363, #26864, #27302, #18264, #22497, #27157 ),
 .UNSPECIFIED., .F., .F.,
 ( 6, 6 ),
 ( 0.000000000000000000, 1.000000000000000000 ),
 .UNSPECIFIED. ) ;
#7686=FACE_OUTER_BOUND ( 'NONE', #4050, .T. ) ;
#7687=AXIS2_PLACEMENT_3D ( 'NONE', #3308, #9850, #1146 ) ;
#7688=CARTESIAN_POINT ( 'NONE',  ( 27.75394116159999669, -74.50000000000000000, -27.75394116159999669 ) ) ;
#7690=CARTESIAN_POINT ( 'NONE',  ( -13.85848666890000125, -57.40875702409999803, 21.24403892489999990 ) ) ;
#7691=CIRCLE ( 'NONE', #24887, 30.50381168839999901 ) ;
#7693=CARTESIAN_POINT ( 'NONE',  ( 7.704476223350000375, -25.49730309679999607, -20.86759468720000044 ) ) ;
#7694=DIRECTION ( 'NONE',  ( 0.000000000000000000, 1.000000000000000000, 0.000000000000000000 ) ) ;
#7698=ORIENTED_EDGE ( 'NONE', *, *, #8829, .T. ) ;
#7699=EDGE_CURVE ( 'NONE', #321, #27403, #4534, .T. ) ;
#7703=ORIENTED_EDGE ( 'NONE', *, *, #13945, .T. ) ;
#7704=AXIS2_PLACEMENT_3D ( 'NONE', #28588, #8754, #18109 ) ;
#7708=CARTESIAN_POINT ( 'NONE',  ( 9.226666976270866627, -71.28737387527178271, -26.41755886876856252 ) ) ;
#7709=CARTESIAN_POINT ( 'NONE',  ( -11.19714568606054250, -58.31259697909283801, 20.53605202907456828 ) ) ;
#7711=CARTESIAN_POINT ( 'NONE',  ( -3.564772898129999756, -71.37991020869999659, -28.09246512229999837 ) ) ;
#7712=AXIS2_PLACEMENT_3D ( 'NONE', #5348, #2883, #5202 ) ;
#7717=CARTESIAN_POINT ( 'NONE',  ( 25.49275922260000016, -60.21420103860000239, 1.382187155250000243 ) ) ;
#7722=CARTESIAN_POINT ( 'NONE',  ( 18.94592262313601339, -19.18584073473548557, -9.024080787555618599 ) ) ;
#7725=DIRECTION ( 'NONE',  ( 0.000000000000000000, 1.000000000000000000, 0.000000000000000000 ) ) ;
#7726=CARTESIAN_POINT ( 'NONE',  ( -31.99184496219999829, -74.00000000000000000, -21.97155633679999909 ) ) ;
#7728=CARTESIAN_POINT ( 'NONE',  ( -2.131628207280000317E-15, -89.50000000000000000, 3.042011087470000117E-15 ) ) ;
#7729=ORIENTED_EDGE ( 'NONE', *, *, #12974, .F. ) ;
#7732=CARTESIAN_POINT ( 'NONE',  ( -12.38417342259999998, -18.50000000000000000, 18.05449715319999981 ) ) ;
#7733=CARTESIAN_POINT ( 'NONE',  ( -14.76023875769999982, -79.50000000000000000, 45.51464203040000456 ) ) ;
#7736=EDGE_CURVE ( 'NONE', #212, #13629, #2171, .T. ) ;
#7737=ORIENTED_EDGE ( 'NONE', *, *, #9030, .T. ) ;
#7738=CARTESIAN_POINT ( 'NONE',  ( -12.91055359849999995, -19.42972397700000187, 19.51083068160000167 ) ) ;
#7742=DIRECTION ( 'NONE',  ( 0.000000000000000000, 1.000000000000000000, 0.000000000000000000 ) ) ;
#7743=CARTESIAN_POINT ( 'NONE',  ( 40.00088822930000276, -74.03376264999999989, 7.260991986090000516 ) ) ;
#7744=FACE_OUTER_BOUND ( 'NONE', #15804, .T. ) ;
#7746=CARTESIAN_POINT ( 'NONE',  ( -11.63786782471469472, -61.15154959429087000, -22.95545206538188765 ) ) ;
#7747=DIRECTION ( 'NONE',  ( 0.000000000000000000, 1.000000000000000000, 0.000000000000000000 ) ) ;
#7749=CARTESIAN_POINT ( 'NONE',  ( -32.63463619529999704, -80.04555047089999675, -21.80756975740000314 ) ) ;
#7750=CARTESIAN_POINT ( 'NONE',  ( 8.805019331468974642, -34.63244845351142942, -20.36793970997746683 ) ) ;
#7754=EDGE_CURVE ( 'NONE', #12707, #18811, #15691, .T. ) ;
#7755=B_SPLINE_CURVE_WITH_KNOTS ( 'NONE', 5,
 ( #17138, #23430, #16865, #3741, #26028, #6052, #10542, #4018, #3467, #14934, #8111, #1290, #17000, #26177, #25754, #5781, #12460, #12746 ),
 .UNSPECIFIED., .F., .F.,
 ( 6, 3, 3, 3, 3, 6 ),
 ( 0.000000000000000000, 1.124498255620000053, 2.252774941530000241, 3.380756636300000118, 4.508382774210000221, 5.576981603840000190 ),
 .UNSPECIFIED. ) ;
#7757=CARTESIAN_POINT ( 'NONE',  ( -2.677182103140000132E-13, -79.50000000000000000, 47.25000000000000000 ) ) ;
#7758=CARTESIAN_POINT ( 'NONE',  ( -14.55867152370000106, -64.24504444460001196, 22.15151623919999935 ) ) ;
#7759=EDGE_LOOP ( 'NONE', ( #16606, #21561, #15892, #17329 ) ) ;
#7763=EDGE_CURVE ( 'NONE', #9163, #5413, #24601, .T. ) ;
#7764=CARTESIAN_POINT ( 'NONE',  ( -14.47093452609578534, -74.09305993903939225, 36.25954071149890012 ) ) ;
#7765=CARTESIAN_POINT ( 'NONE',  ( 26.33945410830000000, -66.61054971519999413, 1.262719925200000093 ) ) ;
#7768=CARTESIAN_POINT ( 'NONE',  ( -21.81265874808163829, -79.50000017620000392, -32.68025371919490141 ) ) ;
#7772=CARTESIAN_POINT ( 'NONE',  ( 9.325629373129999067, -40.69288195509999895, -22.74921183549999881 ) ) ;
#7774=ORIENTED_EDGE ( 'NONE', *, *, #21515, .T. ) ;
#7775=CARTESIAN_POINT ( 'NONE',  ( -39.52985788725224126, -73.70809116064897637, 7.234868202893387945 ) ) ;
#7782=CARTESIAN_POINT ( 'NONE',  ( -2.619967198309999912, -19.39383846079999785, -24.29735868990000114 ) ) ;
#7783=DIRECTION ( 'NONE',  ( -0.9704142011833033488, 0.000000000000000000, 0.2414462220490755373 ) ) ;
#7785=CARTESIAN_POINT ( 'NONE',  ( -1.324264341383242671, -74.17281256843145343, 47.12808568046521174 ) ) ;
#7787=CARTESIAN_POINT ( 'NONE',  ( 22.74921183549999881, -40.69288195330000235, -9.325629373219999962 ) ) ;
#7789=CARTESIAN_POINT ( 'NONE',  ( 19.97576656849999921, -38.00000000000000000, -19.97576656849999921 ) ) ;
#7791=ORIENTED_EDGE ( 'NONE', *, *, #16493, .T. ) ;
#7796=CARTESIAN_POINT ( 'NONE',  ( 19.48147788520000034, -35.35038603809999813, -8.986868840649998802 ) ) ;
#7798=CARTESIAN_POINT ( 'NONE',  ( -14.55867152370000106, -64.24504444460001196, 22.15151623919999935 ) ) ;
#7799=DIRECTION ( 'NONE',  ( -0.9704142011833033488, 0.000000000000000000, 0.2414462220490755373 ) ) ;
#7800=CIRCLE ( 'NONE', #11489, 0.5000000000000004441 ) ;
#7801=CARTESIAN_POINT ( 'NONE',  ( 20.54345333939999918, -28.54983945669999912, -8.512196249269999626 ) ) ;
#7803=CARTESIAN_POINT ( 'NONE',  ( -0.8905265619203176497, -65.59529214041724288, -25.37156426618551563 ) ) ;
#7804=CARTESIAN_POINT ( 'NONE',  ( -4.459621975350000156, -72.00000000000000000, -28.73485931899999812 ) ) ;
#7806=CARTESIAN_POINT ( 'NONE',  ( 40.65508461000000295, -75.00000000000000000, -14.75000000000000000 ) ) ;
#7808=CARTESIAN_POINT ( 'NONE',  ( -7.191786296970000159, -73.49999903349998931, 39.02948049420000132 ) ) ;
#7809=DIRECTION ( 'NONE',  ( 0.000000000000000000, -1.000000000000000000, 0.000000000000000000 ) ) ;
#7811=TOROIDAL_SURFACE ( 'NONE', #20835, 10.50000000000000000, 0.5000000000000000000 ) ;
#7812=CARTESIAN_POINT ( 'NONE',  ( 27.75394116159999669, -74.50000000000000000, -27.75394116159999669 ) ) ;
#7813=ADVANCED_FACE ( 'NONE', ( #881 ), #26366, .T. ) ;
#7814=CARTESIAN_POINT ( 'NONE',  ( -22.60001347469999899, -71.86394619589999877, 17.39035019129999782 ) ) ;
#7817=B_SPLINE_CURVE_WITH_KNOTS ( 'NONE', 5,
 ( #12260, #5147, #27602, #18976, #18555, #23079 ),
 .UNSPECIFIED., .F., .F.,
 ( 6, 6 ),
 ( 0.000000000000000000, 1.000000000000000000 ),
 .UNSPECIFIED. ) ;
#7819=DIRECTION ( 'NONE',  ( 1.000000000000000000, 0.000000000000000000, 0.000000000000000000 ) ) ;
#7821=DIRECTION ( 'NONE',  ( 0.000000000000000000, 1.000000000000000000, 0.000000000000000000 ) ) ;
#7824=CARTESIAN_POINT ( 'NONE',  ( 25.26718046270000073, -19.50000000000000000, 6.129403842640000377 ) ) ;
#7825=AXIS2_PLACEMENT_3D ( 'NONE', #28198, #7830, #23830 ) ;
#7826=VERTEX_POINT ( 'NONE', #16136 ) ;
#7827=LINE ( 'NONE', #20662, #20216 ) ;
#7830=DIRECTION ( 'NONE',  ( 0.000000000000000000, -1.000000000000000000, 0.000000000000000000 ) ) ;
#7831=CYLINDRICAL_SURFACE ( 'NONE', #15321, 0.5000000000000004441 ) ;
#7832=CARTESIAN_POINT ( 'NONE',  ( -11.26036340160000115, -74.00000000000000000, 46.75000000000000000 ) ) ;
#7833=VERTEX_POINT ( 'NONE', #11768 ) ;
#7835=CARTESIAN_POINT ( 'NONE',  ( 7.879643458700000380, -36.30219044630000269, -21.38844997820000060 ) ) ;
#7838=CARTESIAN_POINT ( 'NONE',  ( -22.03254124284932658, -73.99999999999018030, -32.03023314507256458 ) ) ;
#7839=ORIENTED_EDGE ( 'NONE', *, *, #25700, .F. ) ;
#7843=CARTESIAN_POINT ( 'NONE',  ( -20.47152924590000111, -62.13502028410000122, 12.48990793220000128 ) ) ;
#7847=CARTESIAN_POINT ( 'NONE',  ( 18.85230044170000241, -18.50000000000000000, -8.028472989549999994 ) ) ;
#7849=VERTEX_POINT ( 'NONE', #27675 ) ;
#7853=CARTESIAN_POINT ( 'NONE',  ( 36.75479982430000092, -80.17662510629999417, -13.92713283259999990 ) ) ;
#7854=CARTESIAN_POINT ( 'NONE',  ( -3.360703170350179736, -72.70510570383657978, -28.43098690957443253 ) ) ;
#7856=B_SPLINE_CURVE_WITH_KNOTS ( 'NONE', 3,
 ( #27268, #14288, #20998, #2795, #20559, #18380, #25081, #23183, #16323, #3092, #1062, #27412, #22903, #3229, #7464, #16172, #11649, #2942, #25234, #5262, #11805, #14149, #11946, #20858, #628, #27705, #917, #9475, #9760, #18671, #27569, #6665, #26785, #11447, #6968 ),
 .UNSPECIFIED., .F., .F.,
 ( 4, 2, 2, 2, 2, 2, 2, 1, 1, 2, 2, 2, 2, 1, 1, 1, 2, 2, 2, 4 ),
 ( 0.000000000000000000, 0.1249999999999768796, 0.1874999999999658051, 0.2187499999999586442, 0.2499999999999514833, 0.3749999999999271694, 0.4374999999999163447, 0.4687499999999097389, 0.4843749999999049649, 0.4921874999999038547, 0.4999999999999027445, 0.6249999999998862021, 0.6874999999998778755, 0.7187499999998737676, 0.7343749999998731015, 0.7421874999998727684, 0.7460937499998714362, 0.7499999999998701039, 0.8749999999999350520, 1.000000000000000000 ),
 .UNSPECIFIED. ) ;
#7858=DIRECTION ( 'NONE',  ( 0.000000000000000000, -1.000000000000000000, 0.000000000000000000 ) ) ;
#7859=CARTESIAN_POINT ( 'NONE',  ( -0.2062713637372527997, -79.57920433296374085, 47.24999999999999289 ) ) ;
#7860=VERTEX_POINT ( 'NONE', #16580 ) ;
#7861=EDGE_CURVE ( 'NONE', #17644, #27454, #3898, .T. ) ;
#7862=CARTESIAN_POINT ( 'NONE',  ( 47.19280906450000401, -74.66667022419999000, -1.149928383719999836 ) ) ;
#7863=ORIENTED_EDGE ( 'NONE', *, *, #3255, .F. ) ;
#7864=CARTESIAN_POINT ( 'NONE',  ( 22.14137210359999841, -52.59522851940000265, 10.05377507689999916 ) ) ;
#7866=VERTEX_POINT ( 'NONE', #14798 ) ;
#7867=CARTESIAN_POINT ( 'NONE',  ( -10.00000000000000000, -89.00000000000000000, 1.224606353819999829E-15 ) ) ;
#7871=CARTESIAN_POINT ( 'NONE',  ( 23.93312658989999875, -65.07443093669999712, -7.727579958389999781 ) ) ;
#7873=CARTESIAN_POINT ( 'NONE',  ( 46.71300948029226419, -79.88636854212663252, -3.440413976676875762 ) ) ;
#7874=ORIENTED_EDGE ( 'NONE', *, *, #2284, .T. ) ;
#7878=DIRECTION ( 'NONE',  ( 0.000000000000000000, 1.000000000000000000, 0.000000000000000000 ) ) ;
#7879=AXIS2_PLACEMENT_3D ( 'NONE', #22610, #11505, #13852 ) ;
#7880=DIRECTION ( 'NONE',  ( 1.000000000000000000, 0.000000000000000000, 0.000000000000000000 ) ) ;
#7883=AXIS2_PLACEMENT_3D ( 'NONE', #21071, #9833, #18740 ) ;
#7884=CARTESIAN_POINT ( 'NONE',  ( -0.7391264416729999009, -79.72071032069999319, 47.25072614749999644 ) ) ;
#7889=CARTESIAN_POINT ( 'NONE',  ( 4.882943008269999509E-15, -74.50000000000000000, -40.00000000000000000 ) ) ;
#7890=CARTESIAN_POINT ( 'NONE',  ( 30.10554275930000045, -74.00208038259998489, -25.08120035429999817 ) ) ;
#7895=AXIS2_PLACEMENT_3D ( 'NONE', #16057, #2532, #17962 ) ;
#7899=CARTESIAN_POINT ( 'NONE',  ( 9.510880446319999848, -36.06003250090000023, -20.82958080039999871 ) ) ;
#7900=CARTESIAN_POINT ( 'NONE',  ( -40.28268501247167421, -74.17548517140301101, -7.244487271028503983 ) ) ;
#7901=CARTESIAN_POINT ( 'NONE',  ( 21.72762743530000051, -37.33446486360000449, -8.509936561279999978 ) ) ;
#7910=ORIENTED_EDGE ( 'NONE', *, *, #7325, .T. ) ;
#7911=CARTESIAN_POINT ( 'NONE',  ( -40.29875214199796574, -74.18716007598280271, 7.243843118860064934 ) ) ;
#7913=CARTESIAN_POINT ( 'NONE',  ( 23.30859914190000026, -49.64525644009999894, -9.491876184740000610 ) ) ;
#7917=CARTESIAN_POINT ( 'NONE',  ( -14.27099507389999999, -74.08594823550001252, 36.51725837320000068 ) ) ;
#7918=CARTESIAN_POINT ( 'NONE',  ( -2.640278312650000014, -19.41837863920000018, -23.60024879370000050 ) ) ;
#7924=CARTESIAN_POINT ( 'NONE',  ( -39.23631980030000221, -73.50064222389998747, -7.229366192830000593 ) ) ;
#7926=CARTESIAN_POINT ( 'NONE',  ( -10.58792824859999904, -27.05112424559999695, -20.39366723639999890 ) ) ;
#7930=CARTESIAN_POINT ( 'NONE',  ( -10.20110288159999890, -80.00000000000000000, 41.00000000000000000 ) ) ;
#7931=CARTESIAN_POINT ( 'NONE',  ( 36.24656994149999889, -79.27200282849999269, -15.05817610060000078 ) ) ;
#7932=DIRECTION ( 'NONE',  ( 1.000000000000000000, 0.000000000000000000, 0.000000000000000000 ) ) ;
#7935=ADVANCED_FACE ( 'NONE', ( #6347 ), #9825, .T. ) ;
#7936=TOROIDAL_SURFACE ( 'NONE', #1008, 10.50000000000000000, 0.5000000000000000000 ) ;
#7938=ORIENTED_EDGE ( 'NONE', *, *, #22270, .T. ) ;
#7939=CARTESIAN_POINT ( 'NONE',  ( -24.63993737860000266, -72.00000000000000000, 17.98210258840000009 ) ) ;
#7942=EDGE_CURVE ( 'NONE', #10479, #5689, #7755, .T. ) ;
#7943=DIRECTION ( 'NONE',  ( 0.000000000000000000, 1.000000000000000000, 0.000000000000000000 ) ) ;
#7944=EDGE_CURVE ( 'NONE', #23662, #17905, #18531, .T. ) ;
#7945=VERTEX_POINT ( 'NONE', #3597 ) ;
#7949=CARTESIAN_POINT ( 'NONE',  ( 23.57688669830000094, -73.34335239639999315, -30.75933940510000042 ) ) ;
#7950=DIRECTION ( 'NONE',  ( -0.9408314849018032389, 0.000000000000000000, 0.3388747807339287932 ) ) ;
#7957=CIRCLE ( 'NONE', #16339, 4.750000000000000000 ) ;
#7961=DIRECTION ( 'NONE',  ( 0.000000000000000000, 1.000000000000000000, 0.000000000000000000 ) ) ;
#7964=EDGE_CURVE ( 'NONE', #9320, #21728, #25890, .T. ) ;
#7965=ORIENTED_EDGE ( 'NONE', *, *, #12776, .T. ) ;
#7969=ORIENTED_EDGE ( 'NONE', *, *, #6439, .T. ) ;
#7971=CARTESIAN_POINT ( 'NONE',  ( 9.720255118479999012, -72.82938648530000592, -26.98670296669999757 ) ) ;
#7972=CARTESIAN_POINT ( 'NONE',  ( 7.356933664330000511, -36.56811125370000326, -21.47791242339999940 ) ) ;
#7973=AXIS2_PLACEMENT_3D ( 'NONE', #25497, #25368, #22894 ) ;
#7975=CARTESIAN_POINT ( 'NONE',  ( -22.13524825866949897, -74.09417207393364890, -32.44781384942801594 ) ) ;
#7976=ORIENTED_EDGE ( 'NONE', *, *, #12380, .F. ) ;
#7979=CARTESIAN_POINT ( 'NONE',  ( -32.74238892021038083, -74.28135380449873537, -22.20662981729911323 ) ) ;
#7981=ORIENTED_EDGE ( 'NONE', *, *, #11049, .F. ) ;
#7984=CARTESIAN_POINT ( 'NONE',  ( -1.420008363560000042, -19.15770089200000115, -22.10039692550000012 ) ) ;
#7986=ORIENTED_EDGE ( 'NONE', *, *, #14662, .F. ) ;
#7989=CARTESIAN_POINT ( 'NONE',  ( 36.70830968599999977, -79.00000000000000000, -14.75000000000000000 ) ) ;
#7991=VECTOR ( 'NONE', #16337, 1000.000000000000000 ) ;
#7992=CIRCLE ( 'NONE', #26604, 4.750000000000000888 ) ;
#7993=EDGE_CURVE ( 'NONE', #27297, #12297, #20057, .T. ) ;
#7994=CARTESIAN_POINT ( 'NONE',  ( 36.76713440047162607, -79.42549758800066684, -14.65509726804374679 ) ) ;
#7997=VERTEX_POINT ( 'NONE', #6499 ) ;
#7999=CARTESIAN_POINT ( 'NONE',  ( 46.72780802417965162, -73.83257802372662582, -2.701702527458963665 ) ) ;
#8003=ORIENTED_EDGE ( 'NONE', *, *, #15980, .F. ) ;
#8004=EDGE_CURVE ( 'NONE', #18698, #3896, #15870, .T. ) ;
#8006=CARTESIAN_POINT ( 'NONE',  ( 47.25008975959999447, -74.83017303949999643, -0.5756401097749999085 ) ) ;
#8008=CARTESIAN_POINT ( 'NONE',  ( 40.70731707320000226, -74.50000000000000000, 7.215414233289999757 ) ) ;
#8009=CARTESIAN_POINT ( 'NONE',  ( 9.644866014229998896, -36.00000000000000000, -20.16453884109999706 ) ) ;
#8010=CARTESIAN_POINT ( 'NONE',  ( -11.73327706972289697, -62.33680847863706731, -23.17541252891790649 ) ) ;
#8011=DIRECTION ( 'NONE',  ( 1.000000000000000000, 0.000000000000000000, 0.000000000000000000 ) ) ;
#8012=ORIENTED_EDGE ( 'NONE', *, *, #15980, .T. ) ;
#8014=FACE_OUTER_BOUND ( 'NONE', #12387, .T. ) ;
#8017=CARTESIAN_POINT ( 'NONE',  ( -2.580650340169999613, -54.98594849529999351, -25.17323918700000362 ) ) ;
#8022=FACE_OUTER_BOUND ( 'NONE', #27548, .T. ) ;
#8024=CARTESIAN_POINT ( 'NONE',  ( 29.84865827459999821, -73.21937500890000194, -25.22286250999999879 ) ) ;
#8025=CARTESIAN_POINT ( 'NONE',  ( -16.01432518157788465, -72.70510571236322050, 23.73092384619475936 ) ) ;
#8027=AXIS2_PLACEMENT_3D ( 'NONE', #3344, #27689, #3483 ) ;
#8029=CIRCLE ( 'NONE', #11748, 6.750000000000000000 ) ;
#8031=ORIENTED_EDGE ( 'NONE', *, *, #22080, .F. ) ;
#8033=CARTESIAN_POINT ( 'NONE',  ( -39.79858521607874167, -73.85166138383344503, -7.247217007272896971 ) ) ;
#8034=B_SPLINE_CURVE_WITH_KNOTS ( 'NONE', 5,
 ( #7225, #16233, #835, #4887, #14217, #11716, #4738, #14061, #22814 ),
 .UNSPECIFIED., .F., .F.,
 ( 6, 3, 6 ),
 ( 0.000000000000000000, 0.5000000000000000000, 1.000000000000000000 ),
 .UNSPECIFIED. ) ;
#8037=EDGE_LOOP ( 'NONE', ( #6049, #18145, #26210, #12524 ) ) ;
#8042=ORIENTED_EDGE ( 'NONE', *, *, #21842, .T. ) ;
#8049=CARTESIAN_POINT ( 'NONE',  ( 25.72091892060000262, -71.70959084179999365, 11.50978681670000014 ) ) ;
#8052=CARTESIAN_POINT ( 'NONE',  ( 9.356041104380000917, -74.50000000000000000, 37.60355029590000697 ) ) ;
#8055=DIRECTION ( 'NONE',  ( 1.000000000000000000, 0.000000000000000000, 0.000000000000000000 ) ) ;
#8061=CARTESIAN_POINT ( 'NONE',  ( 7.859713442080000334, -62.11705451429999414, -22.72424446479999816 ) ) ;
#8062=CARTESIAN_POINT ( 'NONE',  ( -39.18035607909999385, -73.62951539690000402, -7.219507042800000107 ) ) ;
#8068=TOROIDAL_SURFACE ( 'NONE', #28069, 39.75000000000000000, 0.5000000000000000000 ) ;
#8072=DIRECTION ( 'NONE',  ( -0.09756097560976667582, 0.000000000000000000, -0.9952295494196654602 ) ) ;
#8075=AXIS2_PLACEMENT_3D ( 'NONE', #4095, #28571, #8606 ) ;
#8077=CARTESIAN_POINT ( 'NONE',  ( 21.92880668189999938, -37.95796630759999601, -8.677144286330001677 ) ) ;
#8080=CARTESIAN_POINT ( 'NONE',  ( -12.47307327141018263, -62.13475794627616011, -20.48184207972035864 ) ) ;
#8086=DIRECTION ( 'NONE',  ( 1.000000000000000000, 0.000000000000000000, 0.000000000000000000 ) ) ;
#8087=CARTESIAN_POINT ( 'NONE',  ( 21.98819667889999963, -72.24515058779999777, -30.92234068899999855 ) ) ;
#8088=CARTESIAN_POINT ( 'NONE',  ( -22.96356986949999879, -71.26873020080000742, 15.97477082700000217 ) ) ;
#8089=CARTESIAN_POINT ( 'NONE',  ( 19.97576656849999921, -36.00000000000000000, -19.97576656849999921 ) ) ;
#8091=AXIS2_PLACEMENT_3D ( 'NONE', #20657, #7821, #5763 ) ;
#8095=CARTESIAN_POINT ( 'NONE',  ( -10.93437413680000070, -19.50000027030000282, -21.85842452360000010 ) ) ;
#8099=CARTESIAN_POINT ( 'NONE',  ( -2.453168467159999810, -64.58097839929999395, -25.72104876729999745 ) ) ;
#8100=AXIS2_PLACEMENT_3D ( 'NONE', #13040, #28776, #26324 ) ;
#8102=CARTESIAN_POINT ( 'NONE',  ( -19.49041480450000208, -52.62618816519999854, 12.93508487010000074 ) ) ;
#8103=CARTESIAN_POINT ( 'NONE',  ( 2.798556025240000070E-15, -74.00000000000000000, 3.175502518160000051E-15 ) ) ;
#8106=VERTEX_POINT ( 'NONE', #405 ) ;
#8108=DIRECTION ( 'NONE',  ( 0.9704142011833034598, 0.000000000000000000, -0.2414462220490750377 ) ) ;
#8109=CARTESIAN_POINT ( 'NONE',  ( -14.59815756470000103, -79.67649849320000044, 36.63377403959999867 ) ) ;
#8110=AXIS2_PLACEMENT_3D ( 'NONE', #18138, #4588, #27037 ) ;
#8111=CARTESIAN_POINT ( 'NONE',  ( -17.49621775540000002, -18.50000000000000000, 12.96682185270000076 ) ) ;
#8115=CARTESIAN_POINT ( 'NONE',  ( -19.84213263739999888, -59.03816558840000539, 12.43676266369999972 ) ) ;
#8119=EDGE_CURVE ( 'NONE', #9278, #13587, #27441, .T. ) ;
#8125=CARTESIAN_POINT ( 'NONE',  ( 1.509903313490000218E-14, -80.50000000000000000, 40.00000000000000000 ) ) ;
#8126=CARTESIAN_POINT ( 'NONE',  ( 36.54853060579999635, -79.95823378070001297, -14.43173195999999869 ) ) ;
#8127=ORIENTED_EDGE ( 'NONE', *, *, #11125, .F. ) ;
#8129=ADVANCED_FACE ( 'NONE', ( #24421 ), #4623, .T. ) ;
#8130=AXIS2_PLACEMENT_3D ( 'NONE', #26487, #17307, #13211 ) ;
#8134=ORIENTED_EDGE ( 'NONE', *, *, #5861, .F. ) ;
#8135=CARTESIAN_POINT ( 'NONE',  ( 46.45856493942430632, -73.64909968962108167, -3.295201590591422924 ) ) ;
#8136=VERTEX_POINT ( 'NONE', #18010 ) ;
#8138=CARTESIAN_POINT ( 'NONE',  ( 21.01614117329999942, -55.04870336940000186, 10.45594076380000104 ) ) ;
#8139=B_SPLINE_CURVE_WITH_KNOTS ( 'NONE', 5,
 ( #11711, #16382, #22962, #25292, #19004, #16227 ),
 .UNSPECIFIED., .F., .F.,
 ( 6, 6 ),
 ( 0.000000000000000000, 1.000000000000000000 ),
 .UNSPECIFIED. ) ;
#8140=CARTESIAN_POINT ( 'NONE',  ( 7.215414233289999757, -74.50000000000000000, 40.70731707320000226 ) ) ;
#8141=VERTEX_POINT ( 'NONE', #12018 ) ;
#8142=CARTESIAN_POINT ( 'NONE',  ( -38.62788938250000115, -74.00000000000000000, -7.627566167509999495 ) ) ;
#8143=FACE_OUTER_BOUND ( 'NONE', #4850, .T. ) ;
#8144=ORIENTED_EDGE ( 'NONE', *, *, #2493, .T. ) ;
#8145=CARTESIAN_POINT ( 'NONE',  ( 22.97877291159999658, -37.99999999279999230, -9.393614097370001303 ) ) ;
#8147=CARTESIAN_POINT ( 'NONE',  ( 25.49721913128534823, -67.92876907154627020, 10.87395732963725692 ) ) ;
#8148=VERTEX_POINT ( 'NONE', #25448 ) ;
#8151=DIRECTION ( 'NONE',  ( 0.000000000000000000, -1.000000000000000000, 0.000000000000000000 ) ) ;
#8153=ORIENTED_EDGE ( 'NONE', *, *, #20622, .F. ) ;
#8155=CARTESIAN_POINT ( 'NONE',  ( -2.901718461300000218, -80.37804848140000047, 46.68757613950000263 ) ) ;
#8156=CARTESIAN_POINT ( 'NONE',  ( -18.96815154839999806, -18.50000000000000000, 15.18612143080000010 ) ) ;
#8161=CARTESIAN_POINT ( 'NONE',  ( 38.70686962976383683, -73.76099270142834996, 7.188502612221721932 ) ) ;
#8162=FACE_OUTER_BOUND ( 'NONE', #23640, .T. ) ;
#8163=CARTESIAN_POINT ( 'NONE',  ( 23.74158351679999868, -72.51566206409999893, -30.51711889939999978 ) ) ;
#8166=CARTESIAN_POINT ( 'NONE',  ( 21.07002592539999952, -35.62472953780000040, -8.346733960690000842 ) ) ;
#8167=CIRCLE ( 'NONE', #28184, 7.249999999999999112 ) ;
#8169=DIRECTION ( 'NONE',  ( 0.000000000000000000, -1.000000000000000000, 0.000000000000000000 ) ) ;
#8171=ORIENTED_EDGE ( 'NONE', *, *, #1141, .F. ) ;
#8174=CARTESIAN_POINT ( 'NONE',  ( -0.5824085402257914712, -18.95847994161702132, -21.90536633182652437 ) ) ;
#8177=CARTESIAN_POINT ( 'NONE',  ( -11.35954001540000036, -77.00000000000000000, 45.25000000000000000 ) ) ;
#8180=VERTEX_POINT ( 'NONE', #2015 ) ;
#8181=DIRECTION ( 'NONE',  ( 0.000000000000000000, 1.000000000000000000, 0.000000000000000000 ) ) ;
#8182=CARTESIAN_POINT ( 'NONE',  ( -37.60355029590000697, -74.00000000000000000, 9.356041104380000917 ) ) ;
#8183=CARTESIAN_POINT ( 'NONE',  ( 39.40310785678461514, -73.65029154566123282, 7.225850277551550960 ) ) ;
#8185=CARTESIAN_POINT ( 'NONE',  ( 19.27348047750000148, -18.62200670700000060, -8.616470594819999107 ) ) ;
#8186=CARTESIAN_POINT ( 'NONE',  ( -14.66608903329999869, -74.46648494389999939, 36.47374631129999756 ) ) ;
#8188=DIRECTION ( 'NONE',  ( 1.000000000000000000, 0.000000000000000000, -1.887379141859999189E-15 ) ) ;
#8190=EDGE_CURVE ( 'NONE', #25683, #14668, #18155, .T. ) ;
#8193=CARTESIAN_POINT ( 'NONE',  ( 9.526335912539998674, -60.27919896120000232, -23.43111588329999861 ) ) ;
#8194=CARTESIAN_POINT ( 'NONE',  ( -39.59129699350000209, -73.90055525910000256, -7.279149876960000931 ) ) ;
#8195=CARTESIAN_POINT ( 'NONE',  ( 7.355131038309999703, -34.88462684899999999, -21.34291130700000139 ) ) ;
#8196=CARTESIAN_POINT ( 'NONE',  ( -10.70711398520000124, -19.40595403629999893, -21.59314527720000143 ) ) ;
#8202=CARTESIAN_POINT ( 'NONE',  ( 7.426815359109999903, -35.28814234100000391, -21.34788051319999980 ) ) ;
#8203=CARTESIAN_POINT ( 'NONE',  ( 21.47791241899999903, -36.56811125080000835, -7.356933755090000027 ) ) ;
#8204=CARTESIAN_POINT ( 'NONE',  ( -13.48313256510000002, -64.78279493179998383, 21.61455522920000050 ) ) ;
#8205=EDGE_LOOP ( 'NONE', ( #26928, #21662, #25226 ) ) ;
#8207=ADVANCED_FACE ( 'NONE', ( #6520 ), #19766, .F. ) ;
#8208=CARTESIAN_POINT ( 'NONE',  ( -32.75000000000000000, -69.50000000000000000, 6.890159016250000695E-16 ) ) ;
#8215=CARTESIAN_POINT ( 'NONE',  ( -7.135466578850000019, -73.50000064450000536, 38.71640869449999656 ) ) ;
#8216=CARTESIAN_POINT ( 'NONE',  ( 36.40080305694491614, -74.58594345823078697, -14.77956079794565980 ) ) ;
#8217=CARTESIAN_POINT ( 'NONE',  ( 23.56306528260000022, -73.81141447500000652, -31.03614770169999915 ) ) ;
#8218=EDGE_CURVE ( 'NONE', #4593, #6398, #2157, .T. ) ;
#8219=CARTESIAN_POINT ( 'NONE',  ( -22.71590082970000068, -71.15593401950000896, 16.24045227410000081 ) ) ;
#8221=CARTESIAN_POINT ( 'NONE',  ( -19.41155612407374420, -19.49371746088979762, 14.25750765975674739 ) ) ;
#8222=CARTESIAN_POINT ( 'NONE',  ( 6.850353628289999719, -36.56979901409999911, -21.56931449510000220 ) ) ;
#8225=CARTESIAN_POINT ( 'NONE',  ( -10.93437490840835480, -19.23820060856186487, -21.85842320415198614 ) ) ;
#8226=ORIENTED_EDGE ( 'NONE', *, *, #1571, .F. ) ;
#8227=CARTESIAN_POINT ( 'NONE',  ( 22.39433382880000067, -37.06245928150000424, -9.379298933899999469 ) ) ;
#8228=CARTESIAN_POINT ( 'NONE',  ( -2.565688225440000192, -58.62494694620000502, -24.98236248359999934 ) ) ;
#8229=CARTESIAN_POINT ( 'NONE',  ( 9.379298533759998335, -37.06245930440000080, -22.39433306820000169 ) ) ;
#8232=DIRECTION ( 'NONE',  ( 1.000000000000000000, 0.000000000000000000, 0.000000000000000000 ) ) ;
#8235=CARTESIAN_POINT ( 'NONE',  ( 21.48235967180000117, -35.71220925649999600, -7.023816322830000125 ) ) ;
#8237=CARTESIAN_POINT ( 'NONE',  ( -13.85848666890000125, -57.40875702409999803, 21.24403892489999990 ) ) ;
#8238=ORIENTED_EDGE ( 'NONE', *, *, #13476, .T. ) ;
#8240=VERTEX_POINT ( 'NONE', #10855 ) ;
#8243=AXIS2_PLACEMENT_3D ( 'NONE', #17246, #19427, #19154 ) ;
#8245=CARTESIAN_POINT ( 'NONE',  ( -32.19741970148672294, -74.02576585426132283, -22.07384625748134255 ) ) ;
#8247=ORIENTED_EDGE ( 'NONE', *, *, #9030, .F. ) ;
#8256=B_SPLINE_SURFACE_WITH_KNOTS ( 'NONE', 5, 5, ( 
 ( #20943, #15185, #26441, #16983, #8509, #26304 ),
 ( #12440, #28471, #15335, #15054, #8646, #12858 ),
 ( #13012, #24252, #26004, #5897, #14775, #3997 ),
 ( #6181, #21495, #23676, #12724, #3720, #10393 ),
 ( #23964, #1686, #21776, #1551, #21636, #28328 ),
 ( #1827, #10670, #26157, #12580, #19167, #8222 ) ),
 .UNSPECIFIED., .F., .F., .F.,
 ( 6, 6 ),
 ( 6, 6 ),
 ( 7.598609845240000382, 9.882010082849999932 ),
 ( 1.678547873260000101, 2.000000000000000000 ),
 .UNSPECIFIED. ) ;
#8257=DIRECTION ( 'NONE',  ( -1.000000000000000000, 0.000000000000000000, -7.486357007659997978E-17 ) ) ;
#8258=CARTESIAN_POINT ( 'NONE',  ( -1.559612570125768594, -80.07450989126839147, 47.08089326071244329 ) ) ;
#8260=CIRCLE ( 'NONE', #7825, 7.249999999999999112 ) ;
#8261=CARTESIAN_POINT ( 'NONE',  ( 47.25003036660000788, -74.81280582019999770, -0.5683001369479999676 ) ) ;
#8264=CARTESIAN_POINT ( 'NONE',  ( 20.73443730799999685, -53.84184168659999870, 10.63482208240000126 ) ) ;
#8268=CARTESIAN_POINT ( 'NONE',  ( 33.25000000000000000, -69.00000000000000000, -2.691640454479999860E-15 ) ) ;
#8270=CARTESIAN_POINT ( 'NONE',  ( 10.33698648600000070, -72.00000000000000000, -28.69894938910000093 ) ) ;
#8273=CARTESIAN_POINT ( 'NONE',  ( -0.6409979960822642653, -79.61491260298355144, 47.25010901152391796 ) ) ;
#8274=ORIENTED_EDGE ( 'NONE', *, *, #18840, .T. ) ;
#8275=EDGE_CURVE ( 'NONE', #12701, #18300, #26498, .T. ) ;
#8280=CARTESIAN_POINT ( 'NONE',  ( -1.158253037809999997, -52.63055504209999924, -23.23212522879999753 ) ) ;
#8281=CARTESIAN_POINT ( 'NONE',  ( 10.09279242184272718, -72.75205755911096617, -26.86115544024559298 ) ) ;
#8282=CARTESIAN_POINT ( 'NONE',  ( -12.07243358760000085, -67.46050599719998786, -24.77970463289999969 ) ) ;
#8283=VERTEX_POINT ( 'NONE', #18329 ) ;
#8285=DIRECTION ( 'NONE',  ( 0.000000000000000000, 1.000000000000000000, 0.000000000000000000 ) ) ;
#8287=DIRECTION ( 'NONE',  ( 1.000000000000000000, 0.000000000000000000, 0.000000000000000000 ) ) ;
#8288=CARTESIAN_POINT ( 'NONE',  ( 18.69415571529999909, -18.50000000000000000, 9.686494650060000211 ) ) ;
#8289=CARTESIAN_POINT ( 'NONE',  ( -17.13033212710000086, -72.00000000000000000, 23.49748962700000021 ) ) ;
#8291=ORIENTED_EDGE ( 'NONE', *, *, #8119, .F. ) ;
#8295=CARTESIAN_POINT ( 'NONE',  ( 21.31878868039999730, -36.49872739439999947, -8.228180139540000937 ) ) ;
#8296=CARTESIAN_POINT ( 'NONE',  ( 9.079731074819999748, -35.79879667440000190, -19.54912311329999852 ) ) ;
#8299=AXIS2_PLACEMENT_3D ( 'NONE', #19023, #25997, #10248 ) ;
#8300=EDGE_CURVE ( 'NONE', #14853, #2130, #6487, .T. ) ;
#8301=CIRCLE ( 'NONE', #5976, 38.75000000000000000 ) ;
#8304=CARTESIAN_POINT ( 'NONE',  ( 7.633405283620000148, -53.29445792060000286, -21.99751943120000064 ) ) ;
#8306=VERTEX_POINT ( 'NONE', #18473 ) ;
#8307=EDGE_CURVE ( 'NONE', #7391, #11754, #3710, .T. ) ;
#8309=CARTESIAN_POINT ( 'NONE',  ( -21.19242592198007813, -64.57498915307851917, 13.11476673155585360 ) ) ;
#8311=DIRECTION ( 'NONE',  ( 0.000000000000000000, 1.000000000000000000, 0.000000000000000000 ) ) ;
#8312=EDGE_LOOP ( 'NONE', ( #25904, #11385, #9181, #6352 ) ) ;
#8313=FACE_OUTER_BOUND ( 'NONE', #1689, .T. ) ;
#8318=CARTESIAN_POINT ( 'NONE',  ( -1.317572430653283666, -74.17424845055897720, 47.12932669921157469 ) ) ;
#8319=CIRCLE ( 'NONE', #14826, 2.000000000000001776 ) ;
#8320=CARTESIAN_POINT ( 'NONE',  ( 10.20110288159999890, -84.00000000000000000, -41.00000000000000000 ) ) ;
#8321=CARTESIAN_POINT ( 'NONE',  ( 8.029264327879999996, -63.60161137440000090, -23.19827344629999999 ) ) ;
#8323=CARTESIAN_POINT ( 'NONE',  ( 22.26607236109999732, -57.85578495419999712, 10.13866405869999987 ) ) ;
#8327=AXIS2_PLACEMENT_3D ( 'NONE', #13454, #20012, #4432 ) ;
#8330=DIRECTION ( 'NONE',  ( 0.000000000000000000, 1.000000000000000000, 0.000000000000000000 ) ) ;
#8334=ORIENTED_EDGE ( 'NONE', *, *, #5188, .F. ) ;
#8337=CARTESIAN_POINT ( 'NONE',  ( 19.80394448450000056, -31.61664686670000179, -8.966802299960001221 ) ) ;
#8340=SURFACE_SIDE_STYLE ('',( #16392 ) ) ;
#8344=CARTESIAN_POINT ( 'NONE',  ( -10.50000000000000000, -18.50000000000000000, 0.000000000000000000 ) ) ;
#8345=ORIENTED_EDGE ( 'NONE', *, *, #8900, .F. ) ;
#8346=AXIS2_PLACEMENT_3D ( 'NONE', #14656, #21096, #23828 ) ;
#8350=CARTESIAN_POINT ( 'NONE',  ( 22.08965024500000141, -19.46434222019999893, 0.09551833593859999916 ) ) ;
#8351=DIRECTION ( 'NONE',  ( 0.000000000000000000, -1.000000000000000000, 0.000000000000000000 ) ) ;
#8354=CARTESIAN_POINT ( 'NONE',  ( -22.65531121069999898, -72.00000193540000737, 18.22956418530000278 ) ) ;
#8356=CARTESIAN_POINT ( 'NONE',  ( -19.18665701145497238, -19.48886652642410056, 14.08555375221862427 ) ) ;
#8358=CARTESIAN_POINT ( 'NONE',  ( -10.70759194130000047, -18.50000000000000000, 18.17968849400000053 ) ) ;
#8362=CARTESIAN_POINT ( 'NONE',  ( 22.27253482889999958, -37.66179417780000449, -9.067412436450000612 ) ) ;
#8364=AXIS2_PLACEMENT_3D ( 'NONE', #22633, #13734, #24958 ) ;
#8366=CARTESIAN_POINT ( 'NONE',  ( -1.966302623820000095, -61.72813301749999937, -24.36653853009999793 ) ) ;
#8368=DIRECTION ( 'NONE',  ( -0.8830706733883036952, -0.000000000000000000, -0.4692400087391608854 ) ) ;
#8370=EDGE_CURVE ( 'NONE', #26269, #23532, #13467, .T. ) ;
#8371=ADVANCED_FACE ( 'NONE', ( #14515 ), #12449, .T. ) ;
#8372=ORIENTED_EDGE ( 'NONE', *, *, #16533, .T. ) ;
#8373=DIRECTION ( 'NONE',  ( 0.000000000000000000, 1.000000000000000000, 0.000000000000000000 ) ) ;
#8374=CARTESIAN_POINT ( 'NONE',  ( 27.89292634430000106, -74.00000000000000000, 12.34776042340000046 ) ) ;
#8376=CARTESIAN_POINT ( 'NONE',  ( 0.000000000000000000, -65.07443093669999712, 0.000000000000000000 ) ) ;
#8378=CARTESIAN_POINT ( 'NONE',  ( -22.15114526100514070, -74.12004522895882985, -32.51295459047183556 ) ) ;
#8379=TOROIDAL_SURFACE ( 'NONE', #17239, 7.750000000000000000, 0.5000000000000000000 ) ;
#8381=CARTESIAN_POINT ( 'NONE',  ( 22.35420147799999668, -19.18584080579999807, 9.881343264190000752 ) ) ;
#8383=CARTESIAN_POINT ( 'NONE',  ( -19.69730263860000008, -58.97490961110000285, 13.65699954170000119 ) ) ;
#8385=FACE_OUTER_BOUND ( 'NONE', #17034, .T. ) ;
#8392=CARTESIAN_POINT ( 'NONE',  ( -32.60339417960000219, -74.26163306789999297, -21.76180095249999980 ) ) ;
#8393=CARTESIAN_POINT ( 'NONE',  ( 37.00134709710000180, -80.06168491079999683, -13.64132839650000051 ) ) ;
#8396=AXIS2_PLACEMENT_3D ( 'NONE', #227, #9074, #1233 ) ;
#8398=CIRCLE ( 'NONE', #24722, 0.5000000000000027756 ) ;
#8400=CIRCLE ( 'NONE', #28421, 0.5000000000000004441 ) ;
#8402=ORIENTED_EDGE ( 'NONE', *, *, #11420, .T. ) ;
#8403=CARTESIAN_POINT ( 'NONE',  ( 22.54171623719999928, -56.21886023140000077, 10.13951573499999981 ) ) ;
#8404=CARTESIAN_POINT ( 'NONE',  ( 1.678657213230000024E-14, -74.00000000000000000, 7.838174553849999450E-15 ) ) ;
#8409=CARTESIAN_POINT ( 'NONE',  ( 19.52063838700000176, -35.55398684600000081, -8.985157197580001309 ) ) ;
#8412=CARTESIAN_POINT ( 'NONE',  ( 24.46803346076760732, -64.99740952387834625, 10.81838244473379440 ) ) ;
#8415=VECTOR ( 'NONE', #14354, 1000.000000000000000 ) ;
#8417=CARTESIAN_POINT ( 'NONE',  ( 23.40870142566227585, -59.03921358009447573, -0.5708395527905374411 ) ) ;
#8418=ORIENTED_EDGE ( 'NONE', *, *, #24879, .T. ) ;
#8420=CIRCLE ( 'NONE', #7545, 1.000000000000000888 ) ;
#8422=CARTESIAN_POINT ( 'NONE',  ( -19.35716650769999703, -18.50000000000000000, 15.34467347940000082 ) ) ;
#8423=ORIENTED_EDGE ( 'NONE', *, *, #8300, .T. ) ;
#8424=AXIS2_PLACEMENT_3D ( 'NONE', #26048, #28516, #23863 ) ;
#8425=DIRECTION ( 'NONE',  ( 0.000000000000000000, -1.000000000000000000, 0.000000000000000000 ) ) ;
#8426=B_SPLINE_CURVE_WITH_KNOTS ( 'NONE', 3,
 ( #5180, #23384, #12151, #14352, #14063, #23246, #3427, #27482 ),
 .UNSPECIFIED., .F., .F.,
 ( 4, 2, 2, 4 ),
 ( 0.000000000000000000, 0.4999999999999998890, 0.7499999999999998890, 1.000000000000000000 ),
 .UNSPECIFIED. ) ;
#8434=B_SPLINE_SURFACE_WITH_KNOTS ( 'NONE', 5, 5, ( 
 ( #18423, #22951, #820, #27313, #18570, #2839, #22798, #13751, #2990 ),
 ( #18860, #9662, #20762, #27461, #14198, #24975, #7353, #671, #22651 ),
 ( #1107, #7510, #13895, #25283, #16216, #25130, #2692, #18716, #11698 ),
 ( #27615, #5449, #16655, #16371, #5163, #14044, #23092, #23226, #3135 ),
 ( #11989, #20902, #968, #3274, #11549, #9806, #12131, #9945, #27745 ),
 ( #7782, #5858, #7918, #21456, #12402, #21314, #17073, #5991, #28429 ) ),
 .UNSPECIFIED., .F., .F., .F.,
 ( 6, 6 ),
 ( 6, 3, 6 ),
 ( 0.000000000000000000, 46.92994236210000025 ),
 ( 0.000000000000000000, 1.000000000000000000, 2.000000000000000000 ),
 .UNSPECIFIED. ) ;
#8437=ORIENTED_EDGE ( 'NONE', *, *, #25122, .T. ) ;
#8438=CARTESIAN_POINT ( 'NONE',  ( -39.81550290757894572, -73.86170940550850617, -7.247654292443082014 ) ) ;
#8441=CARTESIAN_POINT ( 'NONE',  ( 20.14644966349999677, -35.79581201140000246, -8.987973295479999791 ) ) ;
#8442=CARTESIAN_POINT ( 'NONE',  ( -35.88566914520000495, -74.00000000000000000, -26.69328098980000163 ) ) ;
#8443=ORIENTED_EDGE ( 'NONE', *, *, #20569, .T. ) ;
#8455=CARTESIAN_POINT ( 'NONE',  ( 23.42789372030000195, -57.47571039170000518, 0.04069560979510000037 ) ) ;
#8456=CARTESIAN_POINT ( 'NONE',  ( 22.66044434279999820, -66.11532834579999474, 11.96275783630000156 ) ) ;
#8459=CARTESIAN_POINT ( 'NONE',  ( 47.16974535660000356, -74.50000000000000000, -1.075756255579999987 ) ) ;
#8460=CARTESIAN_POINT ( 'NONE',  ( 4.882943008269999509E-15, -73.00000000000000000, -40.00000000000000000 ) ) ;
#8464=CARTESIAN_POINT ( 'NONE',  ( 27.39441059460000361, -70.03171919160000414, 1.011203377119999969 ) ) ;
#8465=B_SPLINE_CURVE_WITH_KNOTS ( 'NONE', 5,
 ( #22040, #8751, #22183, #22325, #11227, #10928, #17669, #19833, #11064 ),
 .UNSPECIFIED., .F., .F.,
 ( 6, 3, 6 ),
 ( 0.000000000000000000, 0.5000000000000000000, 1.000000000000000000 ),
 .UNSPECIFIED. ) ;
#8468=CARTESIAN_POINT ( 'NONE',  ( 8.007693474490000796, -59.01994772509999621, -22.21260941989999793 ) ) ;
#8470=DIRECTION ( 'NONE',  ( 0.000000000000000000, -1.000000000000000000, 0.000000000000000000 ) ) ;
#8473=EDGE_LOOP ( 'NONE', ( #19051, #780, #5207, #23850 ) ) ;
#8478=EDGE_CURVE ( 'NONE', #15872, #25683, #7014, .T. ) ;
#8479=ORIENTED_EDGE ( 'NONE', *, *, #7469, .T. ) ;
#8482=CARTESIAN_POINT ( 'NONE',  ( 7.600472224660162368, -74.00014642295830924, 38.79568063749191253 ) ) ;
#8485=CARTESIAN_POINT ( 'NONE',  ( 19.93464468349999663, -22.49864794700000203, -8.810945045800000486 ) ) ;
#8490=VECTOR ( 'NONE', #2309, 1000.000000000000114 ) ;
#8493=CARTESIAN_POINT ( 'NONE',  ( 8.282596154190001059, -36.62694670249999973, -21.35529100209999953 ) ) ;
#8497=B_SPLINE_CURVE_WITH_KNOTS ( 'NONE', 3,
 ( #5656, #18646, #12206, #16731, #2916, #7431, #27241, #750, #25626, #9733, #27541, #7585, #25052, #11925, #9446, #7279, #27684, #5084, #14534, #890, #23441, #23020, #3478, #22874, #12341, #20976, #20830, #21250, #25483, #5518, #9595, #25353 ),
 .UNSPECIFIED., .F., .F.,
 ( 4, 2, 2, 1, 2, 2, 2, 2, 1, 2, 2, 2, 2, 1, 1, 2, 2, 4 ),
 ( 0.000000000000000000, 0.1249999999997466194, 0.1874999999996319056, 0.2187499999995851374, 0.2343749999995739519, 0.2499999999995627387, 0.3749999999996432853, 0.4374999999996742051, 0.4687499999996861955, 0.4843749999996909139, 0.4999999999996955768, 0.6249999999998518962, 0.6874999999999206191, 0.7187499999999508171, 0.7343749999999712452, 0.7421874999999767963, 0.7499999999999823475, 1.000000000000000000 ),
 .UNSPECIFIED. ) ;
#8498=CARTESIAN_POINT ( 'NONE',  ( 22.55445185059999957, -19.16174980609999778, 0.9703951553680000286 ) ) ;
#8501=VERTEX_POINT ( 'NONE', #7370 ) ;
#8505=B_SPLINE_SURFACE_WITH_KNOTS ( 'NONE', 5, 5, ( 
 ( #7283, #27392, #20385, #2482, #13682, #16009 ),
 ( #2920, #7440, #22589, #24914, #13826, #22731 ),
 ( #2772, #25210, #23025, #27545, #11627, #20537 ),
 ( #11339, #609, #9452, #5243, #11929, #20245 ),
 ( #18358, #26960, #6997, #27246, #11479, #20836 ),
 ( #16454, #894, #18651, #15860, #24770, #18931 ) ),
 .UNSPECIFIED., .F., .F., .F.,
 ( 6, 6 ),
 ( 6, 6 ),
 ( 1.645588054440000114, 2.780179228649999779 ),
 ( 0.000000000000000000, 2.000000000000000000 ),
 .UNSPECIFIED. ) ;
#8506=FACE_OUTER_BOUND ( 'NONE', #3783, .T. ) ;
#8507=ADVANCED_FACE ( 'NONE', ( #3009 ), #12517, .T. ) ;
#8508=CARTESIAN_POINT ( 'NONE',  ( -18.78219790299999659, -19.46510053389999939, 11.52011550950000007 ) ) ;
#8509=CARTESIAN_POINT ( 'NONE',  ( 7.731040106980000104, -34.67919398040000090, -21.19938061109999694 ) ) ;
#8513=CARTESIAN_POINT ( 'NONE',  ( 36.32450514310000500, -74.54297172050000597, -14.86961494949999896 ) ) ;
#8515=CARTESIAN_POINT ( 'NONE',  ( 21.93060288690000093, -36.53320241969999671, -9.504975477409999485 ) ) ;
#8516=EDGE_CURVE ( 'NONE', #11916, #17492, #9420, .T. ) ;
#8517=CARTESIAN_POINT ( 'NONE',  ( -2.587281238340000122, -58.59418302210000462, -25.28476856499999670 ) ) ;
#8519=CARTESIAN_POINT ( 'NONE',  ( -19.59930190490000257, -56.25996389440000200, 12.99169644580000060 ) ) ;
#8521=CARTESIAN_POINT ( 'NONE',  ( 19.73295371884362837, -19.48431472826634092, -8.781177429089979114 ) ) ;
#8522=EDGE_LOOP ( 'NONE', ( #26159, #28330, #10907, #2379 ) ) ;
#8523=AXIS2_PLACEMENT_3D ( 'NONE', #8052, #4643, #11172 ) ;
#8528=CARTESIAN_POINT ( 'NONE',  ( 19.53322478289999964, -19.46563609400000061, 10.20089682329999903 ) ) ;
#8529=AXIS2_PLACEMENT_3D ( 'NONE', #26259, #21730, #14007 ) ;
#8530=CARTESIAN_POINT ( 'NONE',  ( -22.19498675863994563, -74.23482419401921106, -32.69399667229252771 ) ) ;
#8531=CARTESIAN_POINT ( 'NONE',  ( 20.80373709450000064, -18.50000000000000000, 8.362177511490001436 ) ) ;
#8535=LINE ( 'NONE', #1857, #9251 ) ;
#8537=CARTESIAN_POINT ( 'NONE',  ( -22.65726982507337439, -72.31233190808211475, 17.75628222746567175 ) ) ;
#8539=ORIENTED_EDGE ( 'NONE', *, *, #2949, .T. ) ;
#8540=EDGE_CURVE ( 'NONE', #18713, #4316, #21831, .T. ) ;
#8542=AXIS2_PLACEMENT_3D ( 'NONE', #28050, #10106, #16979 ) ;
#8543=EDGE_CURVE ( 'NONE', #10192, #7301, #22323, .T. ) ;
#8544=CARTESIAN_POINT ( 'NONE',  ( 46.25000000000000000, -80.00000000000000000, -13.75000000000000000 ) ) ;
#8545=CARTESIAN_POINT ( 'NONE',  ( -32.51044675360000014, -74.20254482470001278, -21.89358512240000110 ) ) ;
#8550=VECTOR ( 'NONE', #24134, 1000.000000000000000 ) ;
#8551=ORIENTED_EDGE ( 'NONE', *, *, #17672, .T. ) ;
#8553=ORIENTED_EDGE ( 'NONE', *, *, #9238, .F. ) ;
#8558=CARTESIAN_POINT ( 'NONE',  ( -21.71458294140000334, -79.77274805400000446, -32.69645410180000056 ) ) ;
#8559=EDGE_CURVE ( 'NONE', #15352, #27945, #8034, .T. ) ;
#8563=CARTESIAN_POINT ( 'NONE',  ( 18.48933855830000184, -18.50000000000000000, 10.02928721039999971 ) ) ;
#8569=CIRCLE ( 'NONE', #13707, 3.749999999999996447 ) ;
#8570=CARTESIAN_POINT ( 'NONE',  ( 11.03417617331015776, -72.43641487375192867, -26.87308835027350540 ) ) ;
#8571=CARTESIAN_POINT ( 'NONE',  ( -19.47450221869999964, -19.18187901349999791, 14.31430793610000052 ) ) ;
#8572=ORIENTED_EDGE ( 'NONE', *, *, #25638, .T. ) ;
#8575=CARTESIAN_POINT ( 'NONE',  ( 8.928661026786835819, -37.96769807237074446, -22.13892078761991300 ) ) ;
#8578=CYLINDRICAL_SURFACE ( 'NONE', #14101, 39.24999999999998579 ) ;
#8580=AXIS2_PLACEMENT_3D ( 'NONE', #6586, #1785, #17512 ) ;
#8583=ORIENTED_EDGE ( 'NONE', *, *, #17001, .F. ) ;
#8587=CARTESIAN_POINT ( 'NONE',  ( 19.84902281569999971, -35.76462365300000101, -9.046350557000000236 ) ) ;
#8588=CARTESIAN_POINT ( 'NONE',  ( -7.325370793560000315, -19.50000000000000000, -24.94672208400000102 ) ) ;
#8591=ADVANCED_FACE ( 'NONE', ( #2857 ), #20950, .F. ) ;
#8593=AXIS2_PLACEMENT_3D ( 'NONE', #5290, #947, #22931 ) ;
#8596=CARTESIAN_POINT ( 'NONE',  ( 6.931585813929999951, -44.93330283539999925, -21.84994998139999822 ) ) ;
#8597=CARTESIAN_POINT ( 'NONE',  ( -11.41594964319999939, -19.46510059719999930, -18.84569179369999858 ) ) ;
#8601=CARTESIAN_POINT ( 'NONE',  ( 23.90022363910000180, -27.02040600870000020, 1.451709836199999826 ) ) ;
#8602=CARTESIAN_POINT ( 'NONE',  ( 22.40589624629999932, -65.01950563030000296, 11.38001362950000050 ) ) ;
#8603=CARTESIAN_POINT ( 'NONE',  ( 40.00000000000000000, -84.50000000000000000, 3.574918139289999605E-15 ) ) ;
#8604=ORIENTED_EDGE ( 'NONE', *, *, #15265, .T. ) ;
#8605=ADVANCED_FACE ( 'NONE', ( #9237 ), #27479, .T. ) ;
#8606=DIRECTION ( 'NONE',  ( -1.836909530730000236E-16, 0.000000000000000000, 1.000000000000000000 ) ) ;
#8610=CARTESIAN_POINT ( 'NONE',  ( 26.98550733189999917, -69.11937516950000315, 0.7853522802169999872 ) ) ;
#8613=CARTESIAN_POINT ( 'NONE',  ( -12.47069904039999955, -69.15454048580001256, -24.11318545760000021 ) ) ;
#8614=CARTESIAN_POINT ( 'NONE',  ( 22.44118743279999961, -65.00127796780000722, 11.39886732859999974 ) ) ;
#8615=CARTESIAN_POINT ( 'NONE',  ( -11.27790836820000031, -42.20269670389999561, -22.30245189869999933 ) ) ;
#8620=CARTESIAN_POINT ( 'NONE',  ( 23.40015495273278034, -60.60830808328032049, 10.49714536420149180 ) ) ;
#8623=VERTEX_POINT ( 'NONE', #25435 ) ;
#8624=CARTESIAN_POINT ( 'NONE',  ( 7.596414145187134537, -34.80520804250858902, -21.25273119204720018 ) ) ;
#8627=CARTESIAN_POINT ( 'NONE',  ( 8.563236930420002224, -35.95760432990000055, -20.91612140590000024 ) ) ;
#8630=ORIENTED_EDGE ( 'NONE', *, *, #16848, .T. ) ;
#8631=EDGE_CURVE ( 'NONE', #28649, #17366, #1253, .T. ) ;
#8633=DIRECTION ( 'NONE',  ( 0.000000000000000000, 1.000000000000000000, 0.000000000000000000 ) ) ;
#8634=CARTESIAN_POINT ( 'NONE',  ( -40.00000000000000000, -84.50000000000000000, 1.424842520070000199E-16 ) ) ;
#8637=EDGE_CURVE ( 'NONE', #26317, #2654, #27889, .T. ) ;
#8639=CARTESIAN_POINT ( 'NONE',  ( -12.83931898810000050, -18.86159962690000214, 19.25717532500000218 ) ) ;
#8640=CARTESIAN_POINT ( 'NONE',  ( 18.98618457029999718, -18.50000000000000000, -8.015883169030001199 ) ) ;
#8641=EDGE_CURVE ( 'NONE', #14463, #13115, #4151, .T. ) ;
#8644=CARTESIAN_POINT ( 'NONE',  ( -12.76535171569999783, -68.20221627489999605, -23.31268819860000008 ) ) ;
#8645=CARTESIAN_POINT ( 'NONE',  ( 30.97576656850000276, -38.00000000000000000, -19.97576656849999921 ) ) ;
#8646=CARTESIAN_POINT ( 'NONE',  ( 7.429758031459999579, -34.95414986760000176, -21.31951852479999943 ) ) ;
#8647=CIRCLE ( 'NONE', #24471, 7.249999999999999112 ) ;
#8648=CARTESIAN_POINT ( 'NONE',  ( 18.97302707929999599, -20.32897095030000045, -9.021553180059999733 ) ) ;
#8650=CARTESIAN_POINT ( 'NONE',  ( 8.982198732169999644, -19.49132059749999968, -19.39131246359999849 ) ) ;
#8652=CARTESIAN_POINT ( 'NONE',  ( -12.47194051069999965, -65.04696943620000127, 21.82660845869999733 ) ) ;
#8653=CARTESIAN_POINT ( 'NONE',  ( 8.933651848329999368, -37.34495684180000552, -22.03427839560000123 ) ) ;
#8655=CARTESIAN_POINT ( 'NONE',  ( -20.45998242170000125, -52.56313962730000355, 14.78974999389999923 ) ) ;
#8659=CARTESIAN_POINT ( 'NONE',  ( 21.37164028449999975, -35.51902737180000003, -7.548682025549999786 ) ) ;
#8661=EDGE_LOOP ( 'NONE', ( #716, #24278, #27965, #21098 ) ) ;
#8662=FACE_OUTER_BOUND ( 'NONE', #6522, .T. ) ;
#8663=EDGE_CURVE ( 'NONE', #18945, #1175, #17667, .T. ) ;
#8664=CARTESIAN_POINT ( 'NONE',  ( 20.50323656299999797, -45.99732788909999925, 10.49340800629999926 ) ) ;
#8665=DIRECTION ( 'NONE',  ( 0.000000000000000000, 1.000000000000000000, 0.000000000000000000 ) ) ;
#8668=CARTESIAN_POINT ( 'NONE',  ( 8.271554555860001656, -65.04365450350000799, -23.74272563809999781 ) ) ;
#8669=ORIENTED_EDGE ( 'NONE', *, *, #18503, .T. ) ;
#8670=CARTESIAN_POINT ( 'NONE',  ( -12.59478316103309758, -72.72581917438233745, -25.71960458748240086 ) ) ;
#8671=CARTESIAN_POINT ( 'NONE',  ( -22.97965035359588626, -72.72581917439157451, 17.08983009374688322 ) ) ;
#8672=CARTESIAN_POINT ( 'NONE',  ( 22.29407657802536846, -58.30792671702914021, -7.076158844936190739 ) ) ;
#8674=CARTESIAN_POINT ( 'NONE',  ( 32.75000000000000000, -69.50000000000000000, 3.321731688439999685E-15 ) ) ;
#8675=CARTESIAN_POINT ( 'NONE',  ( -32.51340285799999918, -74.11800272920001476, -22.15126936060000062 ) ) ;
#8676=CARTESIAN_POINT ( 'NONE',  ( -22.24051182591864873, -79.62418415837113628, -32.83124725485127726 ) ) ;
#8677=ORIENTED_EDGE ( 'NONE', *, *, #5478, .F. ) ;
#8678=CARTESIAN_POINT ( 'NONE',  ( 19.56129018700000088, -35.88702891199999812, -9.158871637020000733 ) ) ;
#8682=EDGE_LOOP ( 'NONE', ( #7276, #428, #16622, #14130 ) ) ;
#8684=CARTESIAN_POINT ( 'NONE',  ( 46.38121015490000332, -73.57738697389999061, -3.489819008620000051 ) ) ;
#8687=CARTESIAN_POINT ( 'NONE',  ( -22.38372304750000197, -80.07464437650000377, -32.45232253209999840 ) ) ;
#8690=CARTESIAN_POINT ( 'NONE',  ( 8.522642244679998313, -37.33399608140000225, -21.80457156990000200 ) ) ;
#8692=CARTESIAN_POINT ( 'NONE',  ( 27.11492913210000211, -72.00000000000000000, 10.50528373760000100 ) ) ;
#8695=CARTESIAN_POINT ( 'NONE',  ( 36.22844186549999534, -74.00000000000000000, -13.75000000000000000 ) ) ;
#8697=CARTESIAN_POINT ( 'NONE',  ( -24.10762033259999981, -79.50000000000000000, -34.71422205039999653 ) ) ;
#8700=CARTESIAN_POINT ( 'NONE',  ( 21.92880674030000065, -37.95796630489999757, -8.677144366489999427 ) ) ;
#8704=FACE_OUTER_BOUND ( 'NONE', #2054, .T. ) ;
#8709=TOROIDAL_SURFACE ( 'NONE', #15211, 0.5000000000000000000, 0.5000000000000000000 ) ;
#8711=AXIS2_PLACEMENT_3D ( 'NONE', #15364, #12883, #19335 ) ;
#8713=VERTEX_POINT ( 'NONE', #9961 ) ;
#8715=ORIENTED_EDGE ( 'NONE', *, *, #3151, .F. ) ;
#8717=CIRCLE ( 'NONE', #13390, 7.750000000000000000 ) ;
#8719=DIRECTION ( 'NONE',  ( 0.000000000000000000, 1.000000000000000000, 0.000000000000000000 ) ) ;
#8720=ORIENTED_EDGE ( 'NONE', *, *, #243, .F. ) ;
#8722=EDGE_CURVE ( 'NONE', #7826, #26140, #13603, .T. ) ;
#8727=CARTESIAN_POINT ( 'NONE',  ( 22.62080797868468451, -64.93834956056363694, 11.20705156649500367 ) ) ;
#8731=CARTESIAN_POINT ( 'NONE',  ( 27.49607050420000220, -45.73899999920000425, 1.934818144049999855 ) ) ;
#8735=CARTESIAN_POINT ( 'NONE',  ( 22.03613531989999785, -19.46548176030000121, -0.1168477070839999965 ) ) ;
#8736=CARTESIAN_POINT ( 'NONE',  ( -14.48027910668785090, -80.37149491588407102, 36.48148420943337555 ) ) ;
#8742=EDGE_LOOP ( 'NONE', ( #27458, #2529, #17992 ) ) ;
#8743=CARTESIAN_POINT ( 'NONE',  ( 38.62788659690000515, -74.00000000000000000, -7.627568735119999666 ) ) ;
#8746=CARTESIAN_POINT ( 'NONE',  ( 23.33794867324012756, -74.10671401505453559, -31.32117936075259834 ) ) ;
#8748=CARTESIAN_POINT ( 'NONE',  ( -11.31871588699999975, -57.41946978100000365, -22.35641894780000172 ) ) ;
#8749=ORIENTED_EDGE ( 'NONE', *, *, #15481, .T. ) ;
#8751=CARTESIAN_POINT ( 'NONE',  ( 23.23309277570114162, -57.41957472273993801, -9.464544134220355787 ) ) ;
#8752=VECTOR ( 'NONE', #17841, 1000.000000000000000 ) ;
#8753=ORIENTED_EDGE ( 'NONE', *, *, #22668, .F. ) ;
#8754=DIRECTION ( 'NONE',  ( 1.000000000000000000, 0.000000000000000000, 2.220446049250000002E-16 ) ) ;
#8755=DIRECTION ( 'NONE',  ( 0.000000000000000000, -1.000000000000000000, 0.000000000000000000 ) ) ;
#8758=ORIENTED_EDGE ( 'NONE', *, *, #10051, .T. ) ;
#8760=CARTESIAN_POINT ( 'NONE',  ( 2.842170943039999687E-14, -74.00000000000000000, 1.776356839399999804E-15 ) ) ;
#8761=CARTESIAN_POINT ( 'NONE',  ( 18.94592261899999741, -19.50000000009999823, -9.024080787920000901 ) ) ;
#8762=CARTESIAN_POINT ( 'NONE',  ( -40.00000000000000000, -77.00000000000000000, 0.000000000000000000 ) ) ;
#8765=DIRECTION ( 'NONE',  ( -0.3687499999999802047, 0.000000000000000000, 0.9295286103719532234 ) ) ;
#8768=FACE_OUTER_BOUND ( 'NONE', #19182, .T. ) ;
#8771=CARTESIAN_POINT ( 'NONE',  ( 21.71614775840000178, -18.61783141309999934, 0.2114479593869999785 ) ) ;
#8774=CARTESIAN_POINT ( 'NONE',  ( -11.35954001540000036, -74.00000000000000000, 46.75000000000000000 ) ) ;
#8776=CARTESIAN_POINT ( 'NONE',  ( -13.92598445589999834, -18.50000000000000000, 19.64619795940000202 ) ) ;
#8777=DIRECTION ( 'NONE',  ( 0.8479091047340885368, 0.000000000000000000, -0.5301416321220553396 ) ) ;
#8778=AXIS2_PLACEMENT_3D ( 'NONE', #21078, #27645, #1139 ) ;
#8781=VECTOR ( 'NONE', #2072, 1000.000000000000000 ) ;
#8783=CARTESIAN_POINT ( 'NONE',  ( 25.78653733048833274, -61.62289756460010182, 1.407790978842422991 ) ) ;
#8785=CARTESIAN_POINT ( 'NONE',  ( 47.25000000000000000, -82.25000000000000000, 7.327133149349999745E-15 ) ) ;
#8787=ORIENTED_EDGE ( 'NONE', *, *, #27284, .T. ) ;
#8788=CARTESIAN_POINT ( 'NONE',  ( 8.153556109420000197, -19.46889320269999857, -20.47461235829999993 ) ) ;
#8792=CARTESIAN_POINT ( 'NONE',  ( -12.70376715600000139, -58.97497545609999747, 20.32514926010000167 ) ) ;
#8793=CARTESIAN_POINT ( 'NONE',  ( -14.65665288169999947, -79.50000000000000000, 36.94583914790000279 ) ) ;
#8797=CARTESIAN_POINT ( 'NONE',  ( -19.61382872410000289, -55.05312981980000586, 12.65941854959999979 ) ) ;
#8800=AXIS2_PLACEMENT_3D ( 'NONE', #3046, #7115, #27361 ) ;
#8804=CARTESIAN_POINT ( 'NONE',  ( 21.51316767409999997, -36.56981899810000414, -7.049162417470000719 ) ) ;
#8805=DIRECTION ( 'NONE',  ( 0.000000000000000000, 1.000000000000000000, 0.000000000000000000 ) ) ;
#8806=ORIENTED_EDGE ( 'NONE', *, *, #15481, .F. ) ;
#8809=DIRECTION ( 'NONE',  ( 0.7071067811865475727, 0.000000000000000000, 0.7071067811865475727 ) ) ;
#8810=CARTESIAN_POINT ( 'NONE',  ( 20.22207915179999915, -26.09432050500000244, 9.873638696180000451 ) ) ;
#8812=CARTESIAN_POINT ( 'NONE',  ( -13.94259793059999986, -74.00000000000000000, 36.22705481479999889 ) ) ;
#8813=CARTESIAN_POINT ( 'NONE',  ( 9.685027244209999608, -66.27232962659999771, -24.54482743630000030 ) ) ;
#8815=ORIENTED_EDGE ( 'NONE', *, *, #5891, .T. ) ;
#8818=CARTESIAN_POINT ( 'NONE',  ( 21.79177587533808236, -19.48886652631049188, 9.573355507166157352 ) ) ;
#8819=AXIS2_PLACEMENT_3D ( 'NONE', #24429, #6505, #26616 ) ;
#8820=CARTESIAN_POINT ( 'NONE',  ( 22.91500301472982315, -62.03080628915128614, -7.299858054674131402 ) ) ;
#8821=ORIENTED_EDGE ( 'NONE', *, *, #18906, .T. ) ;
#8822=DIRECTION ( 'NONE',  ( 1.000000000000000000, 0.000000000000000000, 0.000000000000000000 ) ) ;
#8823=CARTESIAN_POINT ( 'NONE',  ( -32.17258283129999796, -74.02008960720000630, -21.87546129999999778 ) ) ;
#8824=ORIENTED_EDGE ( 'NONE', *, *, #14651, .T. ) ;
#8825=EDGE_CURVE ( 'NONE', #9115, #5383, #425, .T. ) ;
#8827=DIRECTION ( 'NONE',  ( -0.8687683739962963614, -0.3326668106478661846, 0.3668437070977342285 ) ) ;
#8829=EDGE_CURVE ( 'NONE', #23155, #9669, #3836, .T. ) ;
#8833=CARTESIAN_POINT ( 'NONE',  ( 46.44492052809999905, -73.92805234950000681, -3.607313045449999755 ) ) ;
#8834=APPLICATION_CONTEXT ( 'automotive_design' ) ;
#8835=ORIENTED_EDGE ( 'NONE', *, *, #25678, .F. ) ;
#8837=CARTESIAN_POINT ( 'NONE',  ( 0.000000000000000000, -82.25000000000000000, 0.000000000000000000 ) ) ;
#8838=CARTESIAN_POINT ( 'NONE',  ( 20.84246830319968069, -57.47571038088945983, 10.69856926729981872 ) ) ;
#8841=ORIENTED_EDGE ( 'NONE', *, *, #1923, .T. ) ;
#8842=CARTESIAN_POINT ( 'NONE',  ( -10.61287167059999881, -19.46510050329999686, 19.30934957549999709 ) ) ;
#8846=ORIENTED_EDGE ( 'NONE', *, *, #26245, .T. ) ;
#8849=CARTESIAN_POINT ( 'NONE',  ( -22.09341704730000089, -74.03505044649999434, -32.27636733649999456 ) ) ;
#8850=CARTESIAN_POINT ( 'NONE',  ( -1.984042180019999879, -56.24740423709999249, -23.80057596580000023 ) ) ;
#8852=CARTESIAN_POINT ( 'NONE',  ( 11.81986579350000000, -72.00000321289999761, -27.35691362350000233 ) ) ;
#8853=CARTESIAN_POINT ( 'NONE',  ( 21.34788034980000049, -35.28814072549999281, -7.426815654249999454 ) ) ;
#8854=VERTEX_POINT ( 'NONE', #1667 ) ;
#8856=CARTESIAN_POINT ( 'NONE',  ( 20.30256298825100103, -72.52349576872460091, -31.02298866334802341 ) ) ;
#8858=DIRECTION ( 'NONE',  ( -0.9704142011833033488, 0.000000000000000000, -0.2414462220490755373 ) ) ;
#8862=ADVANCED_FACE ( 'NONE', ( #10504 ), #12063, .F. ) ;
#8866=EDGE_CURVE ( 'NONE', #26695, #10529, #10637, .T. ) ;
#8870=LINE ( 'NONE', #11196, #25174 ) ;
#8872=ORIENTED_EDGE ( 'NONE', *, *, #3030, .T. ) ;
#8873=CARTESIAN_POINT ( 'NONE',  ( 29.82685776330000138, -73.10703858080000828, -25.25856749939999801 ) ) ;
#8875=DIRECTION ( 'NONE',  ( 0.000000000000000000, 0.000000000000000000, -1.000000000000000000 ) ) ;
#8879=CIRCLE ( 'NONE', #1919, 39.25000000000000000 ) ;
#8880=CARTESIAN_POINT ( 'NONE',  ( 21.54175492566420758, -37.57472077364804619, -7.824415534489649993 ) ) ;
#8884=CARTESIAN_POINT ( 'NONE',  ( -21.35786096709999882, -65.07443093669999712, 13.27975207949999970 ) ) ;
#8885=CARTESIAN_POINT ( 'NONE',  ( -14.90808802380093567, -79.75935533160925672, 36.30859255103454331 ) ) ;
#8886=CARTESIAN_POINT ( 'NONE',  ( 40.14660266869234562, -74.07739338297623988, 7.248706349661884651 ) ) ;
#8888=CARTESIAN_POINT ( 'NONE',  ( -2.719187424204038805, -64.35840095536138961, -26.13123326132488344 ) ) ;
#8890=CARTESIAN_POINT ( 'NONE',  ( 7.082639064089999437, -58.88902008639999508, -22.31331248359999719 ) ) ;
#8892=CARTESIAN_POINT ( 'NONE',  ( 26.57206512919999852, -68.20221323439999139, 0.6012600223039999969 ) ) ;
#8894=CARTESIAN_POINT ( 'NONE',  ( 9.464545271429999573, -57.41957453189999683, -23.23309258220000117 ) ) ;
#8895=CARTESIAN_POINT ( 'NONE',  ( -12.79700594729999885, -68.93455661459999817, -23.67518218120000384 ) ) ;
#8896=CARTESIAN_POINT ( 'NONE',  ( -11.10145580579999880, -49.82767789670000269, -21.89191623019999966 ) ) ;
#8897=EDGE_CURVE ( 'NONE', #3127, #8919, #5565, .T. ) ;
#8900=EDGE_CURVE ( 'NONE', #5317, #6780, #478, .T. ) ;
#8901=VECTOR ( 'NONE', #10317, 1000.000000000000000 ) ;
#8905=CARTESIAN_POINT ( 'NONE',  ( -10.20110288159999890, -80.50000000000000000, 41.00000000000000000 ) ) ;
#8910=B_SPLINE_SURFACE_WITH_KNOTS ( 'NONE', 5, 5, ( 
 ( #20824, #1296, #27537, #3066, #886, #23436, #9728, #16444, #10139 ),
 ( #5787, #25347, #9591, #14261, #23154, #19058, #25622, #746, #5513 ),
 ( #7843, #1169, #20972, #3198, #12057, #18788, #14400, #23291, #12199 ),
 ( #21114, #10008, #16726, #3473, #23566, #3604, #12464, #17141, #5918 ),
 ( #28079, #8115, #26030, #1709, #8383, #6057, #26179, #10417, #1577 ),
 ( #10547, #14937, #6502, #17288, #19463, #28352, #21799, #14801, #23841 ) ),
 .UNSPECIFIED., .F., .F., .F.,
 ( 6, 6 ),
 ( 6, 3, 6 ),
 ( 112.4382702900000055, 122.9399824959999989 ),
 ( 0.000000000000000000, 1.000000000000000000, 2.000000000000000000 ),
 .UNSPECIFIED. ) ;
#8911=CARTESIAN_POINT ( 'NONE',  ( 20.74932100510000055, -22.46373488209999891, -7.718703100189999944 ) ) ;
#8912=CARTESIAN_POINT ( 'NONE',  ( 22.50268842703188099, -19.46928078220911473, 0.7888462583312775278 ) ) ;
#8914=ORIENTED_EDGE ( 'NONE', *, *, #18709, .T. ) ;
#8917=CARTESIAN_POINT ( 'NONE',  ( 9.385544185329999678, -35.99604478260000207, -19.82171972309999930 ) ) ;
#8919=VERTEX_POINT ( 'NONE', #13429 ) ;
#8921=CIRCLE ( 'NONE', #25254, 22.03370205219999889 ) ;
#8922=EDGE_CURVE ( 'NONE', #21728, #2654, #17683, .T. ) ;
#8924=CARTESIAN_POINT ( 'NONE',  ( 21.56931447779999900, -36.56979901409999911, -6.850353625240000355 ) ) ;
#8925=CARTESIAN_POINT ( 'NONE',  ( 20.30102379280000235, -72.00000000000000000, -30.97095677779999789 ) ) ;
#8927=CARTESIAN_POINT ( 'NONE',  ( -40.00000000000000000, -73.00000000000000000, 2.464695114669999848E-15 ) ) ;
#8931=DIRECTION ( 'NONE',  ( 0.4478680481951062275, 0.000000000000000000, 0.8940996652532120503 ) ) ;
#8936=ORIENTED_EDGE ( 'NONE', *, *, #13271, .F. ) ;
#8937=CARTESIAN_POINT ( 'NONE',  ( 36.26790001819999532, -74.59539775179999310, -15.00677268220000116 ) ) ;
#8938=EDGE_CURVE ( 'NONE', #4316, #20825, #11384, .T. ) ;
#8941=CARTESIAN_POINT ( 'NONE',  ( -11.18243286969999950, -57.47855569860000458, 20.51090136460000224 ) ) ;
#8942=CARTESIAN_POINT ( 'NONE',  ( 40.00000000000000000, -73.50000000000000000, -9.769962616700000205E-15 ) ) ;
#8945=AXIS2_PLACEMENT_3D ( 'NONE', #254, #9096, #22527 ) ;
#8946=CARTESIAN_POINT ( 'NONE',  ( -19.77751067240000182, -52.59522851940000265, 14.14810317790000127 ) ) ;
#8947=FACE_OUTER_BOUND ( 'NONE', #12800, .T. ) ;
#8948=CARTESIAN_POINT ( 'NONE',  ( -11.67870406894427937, -57.47571038307907543, -20.30949878506913109 ) ) ;
#8951=CARTESIAN_POINT ( 'NONE',  ( 7.260231713129999598, -73.74954830080000079, -39.69297836810000035 ) ) ;
#8954=ORIENTED_EDGE ( 'NONE', *, *, #574, .F. ) ;
#8955=DIRECTION ( 'NONE',  ( -0.3687499999999814260, 0.000000000000000000, 0.9295286103719527793 ) ) ;
#8959=CARTESIAN_POINT ( 'NONE',  ( -9.461931989540000032, -18.50000000000000000, -20.21076900759999972 ) ) ;
#8960=EDGE_CURVE ( 'NONE', #7866, #6381, #10914, .T. ) ;
#8961=DIRECTION ( 'NONE',  ( 1.000000000000000000, 0.000000000000000000, 0.000000000000000000 ) ) ;
#8965=CARTESIAN_POINT ( 'NONE',  ( 8.873743607099997988, -64.92653621079999482, -23.73262392499999862 ) ) ;
#8967=VERTEX_POINT ( 'NONE', #18839 ) ;
#8968=CIRCLE ( 'NONE', #23866, 0.5000000000000027756 ) ;
#8969=CARTESIAN_POINT ( 'NONE',  ( -3.252988965690000178, -72.00000000000000000, -30.32986301179999700 ) ) ;
#8972=EDGE_CURVE ( 'NONE', #1691, #22467, #3660, .T. ) ;
#8973=CARTESIAN_POINT ( 'NONE',  ( 20.77309584335343118, -19.47370675685051111, 9.491263722772981026 ) ) ;
#8974=CARTESIAN_POINT ( 'NONE',  ( -40.28438195539999356, -74.37144044069999893, -7.256982118399999848 ) ) ;
#8980=CARTESIAN_POINT ( 'NONE',  ( 41.47915484300000344, -79.00000000000000000, -14.75000000000000000 ) ) ;
#8982=CARTESIAN_POINT ( 'NONE',  ( -0.5436438173659999817, -58.35721741809999941, -23.39762436370000032 ) ) ;
#8983=ORIENTED_EDGE ( 'NONE', *, *, #13648, .T. ) ;
#8985=CARTESIAN_POINT ( 'NONE',  ( -22.17562918277512907, -67.73307646828385487, 14.25710666000342108 ) ) ;
#8987=DIRECTION ( 'NONE',  ( 0.05918472534689767084, 0.000000000000000000, -0.9982470477219616001 ) ) ;
#8988=ORIENTED_EDGE ( 'NONE', *, *, #3312, .T. ) ;
#8990=CARTESIAN_POINT ( 'NONE',  ( 22.01810471777381650, -19.15810975296247776, -0.4634306781688211641 ) ) ;
#8991=CARTESIAN_POINT ( 'NONE',  ( -22.33048751989999658, -79.95649403670000765, -32.64088387420000004 ) ) ;
#8996=DIRECTION ( 'NONE',  ( 0.3687499999999814260, 0.000000000000000000, -0.9295286103719527793 ) ) ;
#8997=ORIENTED_EDGE ( 'NONE', *, *, #834, .F. ) ;
#9000=CIRCLE ( 'NONE', #204, 7.250000000000000000 ) ;
#9002=CARTESIAN_POINT ( 'NONE',  ( -39.07240670449999698, -73.87254094300001839, 7.323170304809999642 ) ) ;
#9003=FACE_OUTER_BOUND ( 'NONE', #12213, .T. ) ;
#9005=VECTOR ( 'NONE', #7549, 1000.000000000000114 ) ;
#9009=CARTESIAN_POINT ( 'NONE',  ( -17.73225090229999878, -18.50000000000000000, 12.18319217400000021 ) ) ;
#9010=ORIENTED_EDGE ( 'NONE', *, *, #19339, .F. ) ;
#9011=EDGE_CURVE ( 'NONE', #9424, #28497, #20969, .T. ) ;
#9013=CARTESIAN_POINT ( 'NONE',  ( 9.315656985238685905, -37.99004392730040536, -22.70406351595718064 ) ) ;
#9017=CIRCLE ( 'NONE', #25337, 2.000000494510000504 ) ;
#9019=LINE ( 'NONE', #13539, #19589 ) ;
#9020=ORIENTED_EDGE ( 'NONE', *, *, #14726, .T. ) ;
#9022=ORIENTED_EDGE ( 'NONE', *, *, #9610, .F. ) ;
#9024=CARTESIAN_POINT ( 'NONE',  ( -13.40823022979999912, -49.82765297159999562, 20.56009738570000067 ) ) ;
#9025=DIRECTION ( 'NONE',  ( 0.000000000000000000, -1.000000000000000000, 0.000000000000000000 ) ) ;
#9026=ORIENTED_EDGE ( 'NONE', *, *, #3188, .T. ) ;
#9028=CARTESIAN_POINT ( 'NONE',  ( 9.038647564319999717, -35.72724395809999720, -19.55068592700000352 ) ) ;
#9030=EDGE_CURVE ( 'NONE', #1569, #22412, #17220, .T. ) ;
#9033=VECTOR ( 'NONE', #7517, 1000.000000000000000 ) ;
#9034=CARTESIAN_POINT ( 'NONE',  ( -9.443564602020002141, -18.50000000000000000, -19.75225778540000121 ) ) ;
#9035=VERTEX_POINT ( 'NONE', #14179 ) ;
#9037=CARTESIAN_POINT ( 'NONE',  ( -20.56694544386164125, -62.25036960902605898, 12.58271708036219572 ) ) ;
#9038=CARTESIAN_POINT ( 'NONE',  ( 40.28268501200326313, -74.17548517097154104, 7.244487271046783583 ) ) ;
#9043=CARTESIAN_POINT ( 'NONE',  ( 10.20110288159999890, -74.50000000000000000, 41.00000000000000000 ) ) ;
#9044=ORIENTED_EDGE ( 'NONE', *, *, #10755, .T. ) ;
#9046=CARTESIAN_POINT ( 'NONE',  ( 27.85911644260000131, -71.04728284579999809, 0.9189804863380000022 ) ) ;
#9049=CARTESIAN_POINT ( 'NONE',  ( 24.26411138551022262, -74.17203985465638993, -30.69540152489543772 ) ) ;
#9051=CARTESIAN_POINT ( 'NONE',  ( 23.93313133829999728, -65.07443449820000581, -7.727578191800000162 ) ) ;
#9052=CARTESIAN_POINT ( 'NONE',  ( 26.46310910940000127, -64.24504445130001784, 1.532420644259999909 ) ) ;
#9054=EDGE_LOOP ( 'NONE', ( #15220, #8226 ) ) ;
#9055=CARTESIAN_POINT ( 'NONE',  ( -2.741827597428787566, -18.87168151092993895, -24.31677555295371462 ) ) ;
#9057=TOROIDAL_SURFACE ( 'NONE', #12760, 38.75000000000000000, 0.5000000000000000000 ) ;
#9060=CARTESIAN_POINT ( 'NONE',  ( 7.135467526410000261, -73.65707963269998970, 38.71641004229999794 ) ) ;
#9065=CIRCLE ( 'NONE', #27699, 39.25000000000000000 ) ;
#9066=CARTESIAN_POINT ( 'NONE',  ( 27.02630527335654165, -72.25875278531135848, -11.40251575530330008 ) ) ;
#9069=CARTESIAN_POINT ( 'NONE',  ( 8.974207715069999480, -36.02836299580000201, -20.55125170219999831 ) ) ;
#9070=CARTESIAN_POINT ( 'NONE',  ( 8.566533541336891489, -19.47798481066859111, -20.04266833404968651 ) ) ;
#9071=EDGE_CURVE ( 'NONE', #300, #26598, #21165, .T. ) ;
#9074=DIRECTION ( 'NONE',  ( 0.000000000000000000, 1.000000000000000000, 0.000000000000000000 ) ) ;
#9075=CARTESIAN_POINT ( 'NONE',  ( -2.641585765738330593, -19.49371746075303236, -23.93965455194797443 ) ) ;
#9078=CARTESIAN_POINT ( 'NONE',  ( 28.25259359185359642, -69.84715190613960090, 2.434813837803762926 ) ) ;
#9080=DIRECTION ( 'NONE',  ( 0.000000000000000000, -1.000000000000000000, 0.000000000000000000 ) ) ;
#9082=CARTESIAN_POINT ( 'NONE',  ( 20.33566493080000015, -36.00000000000000000, -9.885503730140001721 ) ) ;
#9083=DIRECTION ( 'NONE',  ( 0.2414462220490750377, 0.000000000000000000, -0.9704142011833034598 ) ) ;
#9084=CARTESIAN_POINT ( 'NONE',  ( 5.326862811529999898E-15, -74.50000000000000000, -47.25000000000000000 ) ) ;
#9087=ORIENTED_EDGE ( 'NONE', *, *, #14642, .F. ) ;
#9088=CARTESIAN_POINT ( 'NONE',  ( -32.61798281429999946, -80.00000000000000000, -22.71848787769999944 ) ) ;
#9089=ORIENTED_EDGE ( 'NONE', *, *, #22791, .T. ) ;
#9090=CARTESIAN_POINT ( 'NONE',  ( -14.55866013589999852, -64.24504477300000360, 22.15151183529999912 ) ) ;
#9091=EDGE_CURVE ( 'NONE', #23386, #19780, #6080, .T. ) ;
#9093=DIRECTION ( 'NONE',  ( 0.000000000000000000, -1.000000000000000000, 0.000000000000000000 ) ) ;
#9094=CARTESIAN_POINT ( 'NONE',  ( 26.62370195355942570, -72.37489743482117888, 10.79038948701335698 ) ) ;
#9095=CARTESIAN_POINT ( 'NONE',  ( 21.55953482829999857, -36.72040100929999795, -8.607507078249998500 ) ) ;
#9096=DIRECTION ( 'NONE',  ( 0.000000000000000000, -1.000000000000000000, 0.000000000000000000 ) ) ;
#9098=ORIENTED_EDGE ( 'NONE', *, *, #23782, .T. ) ;
#9099=CARTESIAN_POINT ( 'NONE',  ( -7.260602597430000138, -73.82497517469998627, -39.64142120219999299 ) ) ;
#9101=ORIENTED_EDGE ( 'NONE', *, *, #9011, .T. ) ;
#9104=EDGE_CURVE ( 'NONE', #13461, #28257, #22348, .T. ) ;
#9108=CARTESIAN_POINT ( 'NONE',  ( 20.09790167590000109, -39.36582103100000296, 10.61942201829999988 ) ) ;
#9109=AXIS2_PLACEMENT_3D ( 'NONE', #14442, #22920, #16490 ) ;
#9111=CARTESIAN_POINT ( 'NONE',  ( -7.248796347617021851, -73.89318255918183809, -39.86740956960665727 ) ) ;
#9112=CARTESIAN_POINT ( 'NONE',  ( 19.24535105649999878, -18.85523519099999845, 10.43937572179999940 ) ) ;
#9113=CARTESIAN_POINT ( 'NONE',  ( 9.444162208259999858, -68.01046952510000665, -24.98417836379999812 ) ) ;
#9115=VERTEX_POINT ( 'NONE', #10601 ) ;
#9116=DIRECTION ( 'NONE',  ( 0.000000000000000000, 1.000000000000000000, 0.000000000000000000 ) ) ;
#9119=CARTESIAN_POINT ( 'NONE',  ( 21.70557149514094064, -19.48733830550655100, 9.545844344095677059 ) ) ;
#9120=CARTESIAN_POINT ( 'NONE',  ( -40.37851622809999697, -74.24288085059998821, -7.248115061070000031 ) ) ;
#9125=CARTESIAN_POINT ( 'NONE',  ( -26.69328098980000163, -79.50000000000000000, -35.88566914520000495 ) ) ;
#9127=CARTESIAN_POINT ( 'NONE',  ( 19.55068592539999983, -35.72724453810000256, -9.038647860560001135 ) ) ;
#9130=VERTEX_POINT ( 'NONE', #1908 ) ;
#9131=CARTESIAN_POINT ( 'NONE',  ( -22.99750611650443233, -71.51406819562529904, 16.12010929920209179 ) ) ;
#9133=CARTESIAN_POINT ( 'NONE',  ( 45.84677419350000349, -73.65707963269998970, -4.286925650119999709 ) ) ;
#9134=ADVANCED_FACE ( 'NONE', ( #19947 ), #10750, .F. ) ;
#9135=ORIENTED_EDGE ( 'NONE', *, *, #7942, .F. ) ;
#9141=CARTESIAN_POINT ( 'NONE',  ( -17.94180966909999597, -18.50000000000000000, 18.81731824139999887 ) ) ;
#9142=CARTESIAN_POINT ( 'NONE',  ( -2.788137124389999943, -64.22080823580000697, -26.35245158480000072 ) ) ;
#9143=DIRECTION ( 'NONE',  ( 0.4794255386042040601, 0.000000000000000000, 0.8775825618903720926 ) ) ;
#9144=CARTESIAN_POINT ( 'NONE',  ( -21.99191923020000061, -74.04938808419998963, -32.26547628159999448 ) ) ;
#9146=CARTESIAN_POINT ( 'NONE',  ( 21.71672445440000132, -36.72346566049999694, -8.838003628720001004 ) ) ;
#9147=CARTESIAN_POINT ( 'NONE',  ( 47.25000000000000000, -74.00000000000000000, -14.75000000000000000 ) ) ;
#9148=CARTESIAN_POINT ( 'NONE',  ( -18.77305955369999779, -19.15810970359999743, 11.51451047569999808 ) ) ;
#9150=FACE_OUTER_BOUND ( 'NONE', #2143, .T. ) ;
#9151=CARTESIAN_POINT ( 'NONE',  ( 22.17953390099999922, -65.07443087359999367, 11.85657298630000156 ) ) ;
#9154=CARTESIAN_POINT ( 'NONE',  ( 46.25000000000000000, -80.00000000000000000, -4.582575694960000057 ) ) ;
#9157=CARTESIAN_POINT ( 'NONE',  ( -11.69946357949999971, -63.04983560140001231, -23.02234151810000284 ) ) ;
#9162=CARTESIAN_POINT ( 'NONE',  ( -12.04650752959999949, -69.29982884310000202, -25.46956806489999892 ) ) ;
#9163=VERTEX_POINT ( 'NONE', #10469 ) ;
#9164=CARTESIAN_POINT ( 'NONE',  ( -12.06159284910000018, -57.47122623870000524, 20.23241278190000259 ) ) ;
#9166=EDGE_CURVE ( 'NONE', #24375, #26844, #11614, .T. ) ;
#9168=CIRCLE ( 'NONE', #17082, 38.75000000000000000 ) ;
#9169=DIRECTION ( 'NONE',  ( 1.000000000000000000, 0.000000000000000000, 8.344173797130000142E-16 ) ) ;
#9170=EDGE_CURVE ( 'NONE', #6525, #16368, #16538, .T. ) ;
#9172=DIRECTION ( 'NONE',  ( 0.000000000000000000, -1.000000000000000000, 0.000000000000000000 ) ) ;
#9176=CARTESIAN_POINT ( 'NONE',  ( 23.67408170059999861, -68.20869413019998717, 12.08289283440000084 ) ) ;
#9177=ORIENTED_EDGE ( 'NONE', *, *, #24416, .F. ) ;
#9178=DIRECTION ( 'NONE',  ( 1.000000000000000000, 0.000000000000000000, 0.000000000000000000 ) ) ;
#9179=CARTESIAN_POINT ( 'NONE',  ( -19.97968670135914238, -58.31251141496787938, 12.16213319773063795 ) ) ;
#9181=ORIENTED_EDGE ( 'NONE', *, *, #2237, .T. ) ;
#9182=LINE ( 'NONE', #16040, #17411 ) ;
#9184=CARTESIAN_POINT ( 'NONE',  ( -22.52693219800000080, -70.43934371539999972, 17.54847698860000094 ) ) ;
#9185=ORIENTED_EDGE ( 'NONE', *, *, #14536, .F. ) ;
#9186=AXIS2_PLACEMENT_3D ( 'NONE', #18705, #3396, #21037 ) ;
#9189=CARTESIAN_POINT ( 'NONE',  ( -20.19582590579999959, -52.57401960330000179, 14.62459034920000001 ) ) ;
#9190=CARTESIAN_POINT ( 'NONE',  ( 9.307782790770000148, -57.43039233030000190, -22.95932714879999992 ) ) ;
#9192=CARTESIAN_POINT ( 'NONE',  ( 23.16689931189999641, -60.33770510349999938, -9.368374202520000082 ) ) ;
#9200=VERTEX_POINT ( 'NONE', #12803 ) ;
#9201=CARTESIAN_POINT ( 'NONE',  ( 7.219524535890000649, -73.62955962630000784, 39.18053445169999804 ) ) ;
#9203=ADVANCED_FACE ( 'NONE', ( #21713 ), #15320, .T. ) ;
#9208=CARTESIAN_POINT ( 'NONE',  ( 9.140991624659999815, -36.03656764800000190, -20.50715178119999749 ) ) ;
#9211=LINE ( 'NONE', #26867, #27212 ) ;
#9214=FACE_OUTER_BOUND ( 'NONE', #10125, .T. ) ;
#9216=ORIENTED_EDGE ( 'NONE', *, *, #24144, .F. ) ;
#9218=CARTESIAN_POINT ( 'NONE',  ( -13.32719578240000047, -19.17999174859999911, 20.00777489529999897 ) ) ;
#9222=CARTESIAN_POINT ( 'NONE',  ( 25.67981836682682939, -61.04156242073475624, 1.397343546619608690 ) ) ;
#9224=DIRECTION ( 'NONE',  ( 0.000000000000000000, 1.000000000000000000, 0.000000000000000000 ) ) ;
#9225=CARTESIAN_POINT ( 'NONE',  ( -10.54576762539999990, -18.85523517670000260, 19.18725863699999934 ) ) ;
#9226=ORIENTED_EDGE ( 'NONE', *, *, #565, .F. ) ;
#9227=CARTESIAN_POINT ( 'NONE',  ( 36.37866372090000056, -74.74623938790000466, -14.83127960650000077 ) ) ;
#9234=CARTESIAN_POINT ( 'NONE',  ( -13.94341442410000020, -60.21477618889999661, 21.38633822419999930 ) ) ;
#9235=DIRECTION ( 'NONE',  ( 1.000000000000000000, 0.000000000000000000, 0.000000000000000000 ) ) ;
#9237=FACE_OUTER_BOUND ( 'NONE', #15719, .T. ) ;
#9238=EDGE_CURVE ( 'NONE', #17644, #21056, #26591, .T. ) ;
#9239=CARTESIAN_POINT ( 'NONE',  ( 21.77931243370000303, -37.33301741199999668, -8.479935121490001393 ) ) ;
#9240=CARTESIAN_POINT ( 'NONE',  ( -12.01098287860592428, -65.44960518625730117, -24.07027922927386854 ) ) ;
#9244=CARTESIAN_POINT ( 'NONE',  ( -7.215414233289999757, -74.50000000000000000, -40.70731707320000226 ) ) ;
#9245=CARTESIAN_POINT ( 'NONE',  ( 30.65972643183915736, -74.17589974682529430, -24.31452029874836995 ) ) ;
#9251=VECTOR ( 'NONE', #24279, 1000.000000000000000 ) ;
#9257=CARTESIAN_POINT ( 'NONE',  ( 8.235816542629999560E-15, -69.00000000000000000, -40.00000000000000000 ) ) ;
#9258=CARTESIAN_POINT ( 'NONE',  ( -7.246150394362209646, -73.82038814077014877, -39.74699101873454055 ) ) ;
#9259=CARTESIAN_POINT ( 'NONE',  ( 19.77433184639999908, -18.50000000000000000, 8.671591744060000551 ) ) ;
#9263=CARTESIAN_POINT ( 'NONE',  ( -12.02287215850000024, -69.84851671149999675, -25.68298794020000031 ) ) ;
#9264=DIRECTION ( 'NONE',  ( -1.000000000000000000, 0.000000000000000000, 0.000000000000000000 ) ) ;
#9267=CARTESIAN_POINT ( 'NONE',  ( 23.28519330966129530, -63.31588098632251160, -7.446352683915099746 ) ) ;
#9272=AXIS2_PLACEMENT_3D ( 'NONE', #4115, #7332, #22487 ) ;
#9274=EDGE_CURVE ( 'NONE', #26586, #10144, #14874, .T. ) ;
#9275=DIRECTION ( 'NONE',  ( 0.7071067811865492381, 0.000000000000000000, -0.7071067811865457964 ) ) ;
#9278=VERTEX_POINT ( 'NONE', #18222 ) ;
#9280=CARTESIAN_POINT ( 'NONE',  ( -22.90496460322411565, -70.97967975433614640, 15.82655954324508762 ) ) ;
#9281=DIRECTION ( 'NONE',  ( 0.000000000000000000, -1.000000000000000000, 0.000000000000000000 ) ) ;
#9282=CARTESIAN_POINT ( 'NONE',  ( 47.09727354990000237, -74.46036430799999550, -1.896414880740000086 ) ) ;
#9283=ORIENTED_EDGE ( 'NONE', *, *, #6468, .F. ) ;
#9285=CARTESIAN_POINT ( 'NONE',  ( -11.44396836898854986, -61.24981953521358236, 20.93040142220293731 ) ) ;
#9286=CARTESIAN_POINT ( 'NONE',  ( 8.971065451009998526, -36.23955850699999814, -21.20403844530000015 ) ) ;
#9291=CONICAL_SURFACE ( 'NONE', #11615, 25.14975229270001833, 0.4276056667390000787 ) ;
#9292=CARTESIAN_POINT ( 'NONE',  ( 36.34100412979999817, -74.29447080869999809, -14.83252444919999924 ) ) ;
#9294=CARTESIAN_POINT ( 'NONE',  ( -40.70731707320000226, -74.50000000000000000, 7.215414233289999757 ) ) ;
#9295=CARTESIAN_POINT ( 'NONE',  ( -21.60034937969999902, -74.50000000000000000, -32.77174707999999725 ) ) ;
#9300=CARTESIAN_POINT ( 'NONE',  ( -17.90071848410000399, -18.50000000000000000, 11.63286205439999854 ) ) ;
#9301=EDGE_LOOP ( 'NONE', ( #25213, #20498, #23248, #20666, #25527 ) ) ;
#9303=LINE ( 'NONE', #26402, #26080 ) ;
#9305=CARTESIAN_POINT ( 'NONE',  ( 36.70830950850000107, -75.00000000000000000, -14.75000000000000000 ) ) ;
#9307=CARTESIAN_POINT ( 'NONE',  ( 46.12332287689999788, -80.00000000000000000, -4.489694494070000097 ) ) ;
#9310=CARTESIAN_POINT ( 'NONE',  ( -11.29976941730000028, -60.38561542509999924, -21.91412512930000034 ) ) ;
#9312=CARTESIAN_POINT ( 'NONE',  ( 26.88013656499999726, -70.45756452349999677, -11.38838362379999936 ) ) ;
#9314=VECTOR ( 'NONE', #22785, 1000.000000000000114 ) ;
#9318=CARTESIAN_POINT ( 'NONE',  ( -2.131628207279999844E-14, -80.00000000000000000, 1.776356839399999922E-14 ) ) ;
#9320=VERTEX_POINT ( 'NONE', #323 ) ;
#9323=CARTESIAN_POINT ( 'NONE',  ( 8.677144207910000517, -37.95796631070000160, -21.92880662259999980 ) ) ;
#9326=CARTESIAN_POINT ( 'NONE',  ( 21.51723897743652358, -37.39664231660807303, -7.698370384452410953 ) ) ;
#9330=ADVANCED_FACE ( 'NONE', ( #24482 ), #2338, .T. ) ;
#9331=CARTESIAN_POINT ( 'NONE',  ( 39.97648509715650533, -73.96150430830680023, 7.250349464190967375 ) ) ;
#9334=CARTESIAN_POINT ( 'NONE',  ( 37.60355029590000697, -74.00000000000000000, 9.356041104380000917 ) ) ;
#9335=CARTESIAN_POINT ( 'NONE',  ( -40.00000000000000000, -69.00000000000000000, -8.881784197000000993E-16 ) ) ;
#9336=CARTESIAN_POINT ( 'NONE',  ( -14.34007285459999892, -80.00000123130000418, 37.07570051250000631 ) ) ;
#9337=ORIENTED_EDGE ( 'NONE', *, *, #10958, .T. ) ;
#9341=AXIS2_PLACEMENT_3D ( 'NONE', #19903, #17738, #13049 ) ;
#9344=CARTESIAN_POINT ( 'NONE',  ( 32.65605932329999916, -74.00000011560000246, -20.35087570529999823 ) ) ;
#9345=EDGE_CURVE ( 'NONE', #21714, #5681, #6983, .T. ) ;
#9346=CARTESIAN_POINT ( 'NONE',  ( 22.13628285439999743, -57.47600047049999716, -7.675802460419999917 ) ) ;
#9348=CARTESIAN_POINT ( 'NONE',  ( 27.13958535860000154, -67.66818692689999182, 1.745373480479999850 ) ) ;
#9351=CARTESIAN_POINT ( 'NONE',  ( -38.71640881029999548, -73.50000064450000536, -7.135467304789999687 ) ) ;
#9352=DIRECTION ( 'NONE',  ( 0.000000000000000000, -1.000000000000000000, 0.000000000000000000 ) ) ;
#9354=ORIENTED_EDGE ( 'NONE', *, *, #2125, .F. ) ;
#9356=CARTESIAN_POINT ( 'NONE',  ( 7.332335648789999993, -74.23958658489999607, 39.85912817280000553 ) ) ;
#9360=CARTESIAN_POINT ( 'NONE',  ( 22.02882315030000271, -19.46510050329999686, -0.4636558402470000173 ) ) ;
#9362=CARTESIAN_POINT ( 'NONE',  ( 26.82419938582480512, -72.69597502604865724, -10.30336132714409558 ) ) ;
#9363=CARTESIAN_POINT ( 'NONE',  ( -21.43329341219999762, -64.24504445130001784, 15.59675287610000005 ) ) ;
#9364=CARTESIAN_POINT ( 'NONE',  ( 8.573564494670000258, -37.04357955609999919, -21.61801021650000010 ) ) ;
#9368=CARTESIAN_POINT ( 'NONE',  ( 24.39713799250000292, -19.50000027030000282, 1.459766484860000046 ) ) ;
#9369=CARTESIAN_POINT ( 'NONE',  ( -12.91037659697244599, -19.48298570124567419, 19.57229326679139447 ) ) ;
#9371=CARTESIAN_POINT ( 'NONE',  ( -2.563436409524490589, -19.48585536711892985, -23.48409854323134738 ) ) ;
#9374=EDGE_CURVE ( 'NONE', #27229, #1691, #7157, .T. ) ;
#9375=DIRECTION ( 'NONE',  ( 0.000000000000000000, 1.000000000000000000, 0.000000000000000000 ) ) ;
#9380=AXIS2_PLACEMENT_3D ( 'NONE', #20730, #11817, #5275 ) ;
#9382=CIRCLE ( 'NONE', #19164, 0.5000000000000004441 ) ;
#9383=EDGE_CURVE ( 'NONE', #26844, #27945, #11197, .T. ) ;
#9384=CARTESIAN_POINT ( 'NONE',  ( 36.47623142740000191, -74.84544903709999630, -14.77763247909999933 ) ) ;
#9385=DIRECTION ( 'NONE',  ( 0.000000000000000000, 1.000000000000000000, 0.000000000000000000 ) ) ;
#9388=CARTESIAN_POINT ( 'NONE',  ( 21.29431096540000112, -35.00262504610000036, -7.521543753010000444 ) ) ;
#9389=CARTESIAN_POINT ( 'NONE',  ( -0.8216633941299998911, -65.07442867339999282, -25.13631543320000006 ) ) ;
#9391=CARTESIAN_POINT ( 'NONE',  ( 19.36781163719999910, -19.46510053389999939, 10.50580276810000058 ) ) ;
#9394=CARTESIAN_POINT ( 'NONE',  ( 29.21673098384253109, -74.33752570142104332, -26.16904073697999067 ) ) ;
#9399=CARTESIAN_POINT ( 'NONE',  ( 7.383549334360000493, -18.50000000000000000, -19.69582310909999734 ) ) ;
#9401=EDGE_CURVE ( 'NONE', #16196, #27297, #1572, .T. ) ;
#9403=EDGE_CURVE ( 'NONE', #7043, #10820, #3726, .T. ) ;
#9404=CARTESIAN_POINT ( 'NONE',  ( -13.82310862920000005, -74.00000000000000000, 36.20061004779999791 ) ) ;
#9409=CARTESIAN_POINT ( 'NONE',  ( -13.16183723350000179, -70.12921532840000793, -24.09258144820000069 ) ) ;
#9410=FACE_OUTER_BOUND ( 'NONE', #22118, .T. ) ;
#9417=ORIENTED_EDGE ( 'NONE', *, *, #23715, .T. ) ;
#9418=VECTOR ( 'NONE', #12258, 1000.000000000000000 ) ;
#9420=B_SPLINE_CURVE_WITH_KNOTS ( 'NONE', 5,
 ( #18295, #20472, #5026, #9094, #15942, #13914 ),
 .UNSPECIFIED., .F., .F.,
 ( 6, 6 ),
 ( 0.000000000000000000, 1.000000000000000000 ),
 .UNSPECIFIED. ) ;
#9421=CARTESIAN_POINT ( 'NONE',  ( 10.71318590899999990, -36.06167118559999807, -22.60430443919999988 ) ) ;
#9424=VERTEX_POINT ( 'NONE', #1598 ) ;
#9425=ORIENTED_EDGE ( 'NONE', *, *, #8516, .T. ) ;
#9428=CARTESIAN_POINT ( 'NONE',  ( 47.11398222799999758, -74.48400604130000602, -1.625803566960000168 ) ) ;
#9429=ORIENTED_EDGE ( 'NONE', *, *, #5941, .T. ) ;
#9431=CARTESIAN_POINT ( 'NONE',  ( -11.74876062667526355, -63.11832875707892754, 21.36197986565119677 ) ) ;
#9432=CARTESIAN_POINT ( 'NONE',  ( 23.74633046638808409, -64.47177090206558603, 10.70095004269627914 ) ) ;
#9434=CARTESIAN_POINT ( 'NONE',  ( -3.522003140469999849, -68.93885193580000248, -27.83245572350000074 ) ) ;
#9436=CARTESIAN_POINT ( 'NONE',  ( -15.00767853189999990, -70.93206804260000808, 23.42916186189999905 ) ) ;
#9437=ORIENTED_EDGE ( 'NONE', *, *, #9104, .T. ) ;
#9438=FACE_OUTER_BOUND ( 'NONE', #28177, .T. ) ;
#9441=CARTESIAN_POINT ( 'NONE',  ( 24.90655353600000410, -61.83365245859999959, 1.147770447419999895 ) ) ;
#9442=CARTESIAN_POINT ( 'NONE',  ( -21.99985828019999801, -74.00000000000000000, -31.89935321680000158 ) ) ;
#9445=CARTESIAN_POINT ( 'NONE',  ( -7.367678538425209034, -73.99967062276937213, 39.29948535928571118 ) ) ;
#9446=CARTESIAN_POINT ( 'NONE',  ( 36.63849838837199968, -74.19274952788697419, -14.34036756977614679 ) ) ;
#9450=CIRCLE ( 'NONE', #24815, 1.000000000000000888 ) ;
#9452=CARTESIAN_POINT ( 'NONE',  ( 8.783852041339999417, -35.09305114600000053, -20.45839261020000066 ) ) ;
#9454=FACE_OUTER_BOUND ( 'NONE', #14873, .T. ) ;
#9455=ORIENTED_EDGE ( 'NONE', *, *, #12586, .T. ) ;
#9456=CARTESIAN_POINT ( 'NONE',  ( 46.41171862319999519, -80.37540335289999405, -3.517809264200000285 ) ) ;
#9460=CARTESIAN_POINT ( 'NONE',  ( -12.89905543549999933, -65.07442822920000935, -21.58992615660000070 ) ) ;
#9461=AXIS2_PLACEMENT_3D ( 'NONE', #3668, #10476, #21720 ) ;
#9468=FACE_OUTER_BOUND ( 'NONE', #3708, .T. ) ;
#9469=DIRECTION ( 'NONE',  ( 1.000000000000000000, 0.000000000000000000, 0.000000000000000000 ) ) ;
#9470=ORIENTED_EDGE ( 'NONE', *, *, #1602, .F. ) ;
#9471=FACE_OUTER_BOUND ( 'NONE', #8682, .T. ) ;
#9472=CARTESIAN_POINT ( 'NONE',  ( -31.99658184870000355, -74.50000000000000000, -31.99658184870000355 ) ) ;
#9473=CONICAL_SURFACE ( 'NONE', #24366, 21.99999999999999645, 0.03490658503990158590 ) ;
#9475=CARTESIAN_POINT ( 'NONE',  ( -10.52298218897619186, -19.48483231357551304, -21.08077323561843741 ) ) ;
#9478=CARTESIAN_POINT ( 'NONE',  ( 25.62591688519999877, -71.82672919469999329, 11.84408135179999988 ) ) ;
#9482=CARTESIAN_POINT ( 'NONE',  ( -20.38307042409243408, -61.36262250532579543, 12.44304614358050642 ) ) ;
#9483=CARTESIAN_POINT ( 'NONE',  ( 9.356041104380000917, -74.00000000000000000, -37.60355029590000697 ) ) ;
#9486=DIRECTION ( 'NONE',  ( 0.000000000000000000, -1.000000000000000000, 0.000000000000000000 ) ) ;
#9487=CARTESIAN_POINT ( 'NONE',  ( 7.727581852389999284, -65.07443093669999712, -23.93312597839999967 ) ) ;
#9489=ORIENTED_EDGE ( 'NONE', *, *, #2849, .T. ) ;
#9491=ADVANCED_FACE ( 'NONE', ( #1460 ), #25600, .F. ) ;
#9492=CARTESIAN_POINT ( 'NONE',  ( -19.33917618720000320, -45.99732788909999925, 12.50961972019999990 ) ) ;
#9494=CARTESIAN_POINT ( 'NONE',  ( -11.78425688200000110, -72.00000000000000000, -26.58404760160000180 ) ) ;
#9495=CARTESIAN_POINT ( 'NONE',  ( 22.26662627150000162, -57.47855597999999588, -7.066909368720000195 ) ) ;
#9497=CARTESIAN_POINT ( 'NONE',  ( -10.49977388490000152, -18.50000000000000000, 18.23111608289999808 ) ) ;
#9498=AXIS2_PLACEMENT_3D ( 'NONE', #24917, #7145, #20387 ) ;
#9499=ORIENTED_EDGE ( 'NONE', *, *, #11635, .F. ) ;
#9500=FACE_BOUND ( 'NONE', #17718, .T. ) ;
#9501=ADVANCED_FACE ( 'NONE', ( #6790 ), #20101, .T. ) ;
#9502=CARTESIAN_POINT ( 'NONE',  ( 21.72336075670000000, -37.94103119580000083, -8.348312496720000198 ) ) ;
#9506=CARTESIAN_POINT ( 'NONE',  ( 7.253647055860000137, -74.31845592130000000, 40.32201634399999790 ) ) ;
#9507=CARTESIAN_POINT ( 'NONE',  ( 8.001802476509999096, -18.50000000000000000, -19.02938007170000034 ) ) ;
#9508=CARTESIAN_POINT ( 'NONE',  ( -26.69328098980000163, -74.50000000000000000, -35.88566914520000495 ) ) ;
#9512=CARTESIAN_POINT ( 'NONE',  ( 9.476129726630000860, -36.00000000000000000, -20.06309461859999743 ) ) ;
#9513=ADVANCED_FACE ( 'NONE', ( #14815 ), #17304, .T. ) ;
#9514=CARTESIAN_POINT ( 'NONE',  ( 21.26981850238844984, -34.71690492586082399, -7.540080587919900879 ) ) ;
#9516=CARTESIAN_POINT ( 'NONE',  ( -11.90443957499999961, -64.24504445130001784, -23.68393584109999850 ) ) ;
#9520=AXIS2_PLACEMENT_3D ( 'NONE', #23982, #26463, #28207 ) ;
#9521=CARTESIAN_POINT ( 'NONE',  ( -2.028994704583232167, -19.47131810280622233, -22.58029175209635397 ) ) ;
#9522=CARTESIAN_POINT ( 'NONE',  ( -13.85848666890000125, -57.40875702409999803, 21.24403892489999990 ) ) ;
#9525=CARTESIAN_POINT ( 'NONE',  ( -39.33235237970008313, -73.62392792451801427, 7.219194746715398736 ) ) ;
#9526=CARTESIAN_POINT ( 'NONE',  ( -2.578307999469999778, -52.56313962710000709, -25.11373953509999879 ) ) ;
#9527=CARTESIAN_POINT ( 'NONE',  ( 23.17371582640000227, -44.86350384069999819, -9.449797638930000687 ) ) ;
#9536=CARTESIAN_POINT ( 'NONE',  ( 20.36793975040000149, -34.63244848020000433, -8.805019347009999109 ) ) ;
#9537=CARTESIAN_POINT ( 'NONE',  ( 23.26234223547589153, -59.45680040906446351, 10.43566352099444750 ) ) ;
#9540=ADVANCED_FACE ( 'NONE', ( #21126 ), #7485, .F. ) ;
#9541=CARTESIAN_POINT ( 'NONE',  ( 21.80457179460000106, -37.33399608290000060, -8.522642616350001532 ) ) ;
#9544=B_SPLINE_CURVE_WITH_KNOTS ( 'NONE', 5,
 ( #20580, #644, #20131, #24658, #15605, #200, #14015, #26995, #15901 ),
 .UNSPECIFIED., .F., .F.,
 ( 6, 3, 6 ),
 ( -6.717368912360000444, -6.039642335889999991, -4.007746616509999527 ),
 .UNSPECIFIED. ) ;
#9546=ORIENTED_EDGE ( 'NONE', *, *, #14658, .T. ) ;
#9547=CARTESIAN_POINT ( 'NONE',  ( -3.058911230670000148, -72.82938648530000592, -28.52031834779999997 ) ) ;
#9552=EDGE_CURVE ( 'NONE', #27727, #898, #21619, .T. ) ;
#9555=PLANE ( 'NONE',  #27506 ) ;
#9556=AXIS2_PLACEMENT_3D ( 'NONE', #13705, #19811, #19958 ) ;
#9557=CARTESIAN_POINT ( 'NONE',  ( -37.60355029590000697, -84.00000000000000000, -9.356041104380000917 ) ) ;
#9558=CARTESIAN_POINT ( 'NONE',  ( -7.244146985819436502, -74.18164516872573699, -40.29126735531537662 ) ) ;
#9559=CARTESIAN_POINT ( 'NONE',  ( -14.42755416139999980, -74.19081742459999873, 36.52101890659999839 ) ) ;
#9560=CARTESIAN_POINT ( 'NONE',  ( -21.22624868000000120, -65.72101818089998915, 15.03418113859999927 ) ) ;
#9561=CARTESIAN_POINT ( 'NONE',  ( -36.25000000000000000, -84.50000000000000000, 2.124561919619999789E-15 ) ) ;
#9563=CARTESIAN_POINT ( 'NONE',  ( -11.86976558200000120, -71.47032289400000593, -26.35122234239999983 ) ) ;
#9564=CARTESIAN_POINT ( 'NONE',  ( 8.153551712620000558, -19.43778590579999843, -20.47343976009999977 ) ) ;
#9565=CARTESIAN_POINT ( 'NONE',  ( -6.717799458580000049, -84.50000000000000000, -40.65853658540000026 ) ) ;
#9566=FACE_OUTER_BOUND ( 'NONE', #13048, .T. ) ;
#9569=ORIENTED_EDGE ( 'NONE', *, *, #22344, .T. ) ;
#9570=AXIS2_PLACEMENT_3D ( 'NONE', #6720, #20260, #22607 ) ;
#9571=CARTESIAN_POINT ( 'NONE',  ( -14.09870646349260603, -80.05388654820464467, 36.88642194476569358 ) ) ;
#9575=EDGE_CURVE ( 'NONE', #9035, #25958, #19314, .T. ) ;
#9577=DIRECTION ( 'NONE',  ( 0.9295286103719527793, 0.000000000000000000, 0.3687499999999814260 ) ) ;
#9578=CARTESIAN_POINT ( 'NONE',  ( 47.08605683180000057, -74.34014987910001082, -1.561105320619999848 ) ) ;
#9581=CARTESIAN_POINT ( 'NONE',  ( 7.247933038816999129, -73.86845561477531419, -39.82679900489436164 ) ) ;
#9582=CARTESIAN_POINT ( 'NONE',  ( -11.45610569668674295, -61.34399254273181867, 20.94869055166078908 ) ) ;
#9583=EDGE_CURVE ( 'NONE', #9687, #3916, #26516, .T. ) ;
#9585=CARTESIAN_POINT ( 'NONE',  ( -2.842096223940000055, -64.76590626960000918, -26.52558581780000324 ) ) ;
#9586=CARTESIAN_POINT ( 'NONE',  ( -16.42252987980000256, -71.30682482819999279, 23.34985130180000112 ) ) ;
#9588=CARTESIAN_POINT ( 'NONE',  ( 36.46839126729999947, -74.19089203260000431, -14.49828573059999925 ) ) ;
#9590=CARTESIAN_POINT ( 'NONE',  ( 24.49108460629999939, -63.62177041899999352, -0.2391711755510000093 ) ) ;
#9591=CARTESIAN_POINT ( 'NONE',  ( -20.62138254979999985, -63.58944626250000454, 13.29929482439999866 ) ) ;
#9593=CARTESIAN_POINT ( 'NONE',  ( 28.91458899939999938, -72.00000000000000000, 3.086557976320000396 ) ) ;
#9595=CARTESIAN_POINT ( 'NONE',  ( 36.31482215109925704, -74.00000000000000000, -13.86667273340584039 ) ) ;
#9596=VERTEX_POINT ( 'NONE', #21901 ) ;
#9598=CARTESIAN_POINT ( 'NONE',  ( 22.65540084869999760, -61.59774147150000090, 10.37602781989999912 ) ) ;
#9599=DIRECTION ( 'NONE',  ( 1.000000000000000000, 0.000000000000000000, 0.000000000000000000 ) ) ;
#9602=ORIENTED_EDGE ( 'NONE', *, *, #7098, .T. ) ;
#9603=CARTESIAN_POINT ( 'NONE',  ( 46.85006010219999695, -80.10037130149999030, -2.646644417630000135 ) ) ;
#9605=CARTESIAN_POINT ( 'NONE',  ( -13.35146630740000084, -18.50000000000000000, 18.52320307730000337 ) ) ;
#9606=CARTESIAN_POINT ( 'NONE',  ( -11.31871641740000101, -57.41946977210000114, -22.35641880389999869 ) ) ;
#9607=CARTESIAN_POINT ( 'NONE',  ( -7.135467304789999687, -73.50000064450000536, 38.71640881029999548 ) ) ;
#9609=EDGE_LOOP ( 'NONE', ( #10098, #12531, #4780, #28448 ) ) ;
#9610=EDGE_CURVE ( 'NONE', #12917, #23425, #10508, .T. ) ;
#9613=CARTESIAN_POINT ( 'NONE',  ( 22.45957212879999787, -52.58489974430000302, 10.08523539449999973 ) ) ;
#9616=CARTESIAN_POINT ( 'NONE',  ( 46.25000000000000000, -80.00000000000000000, -4.582575694960000057 ) ) ;
#9618=CARTESIAN_POINT ( 'NONE',  ( 40.35968420270000223, -74.26794181920000426, 7.250122995559999950 ) ) ;
#9620=CARTESIAN_POINT ( 'NONE',  ( 25.52419697193059278, -69.00255572341212940, -8.618219423246786803 ) ) ;
#9622=ORIENTED_EDGE ( 'NONE', *, *, #3758, .F. ) ;
#9623=CARTESIAN_POINT ( 'NONE',  ( -32.69645379630000548, -79.77277768780000144, -21.71458329359999695 ) ) ;
#9624=CARTESIAN_POINT ( 'NONE',  ( -19.95527577780000072, -57.47855601759999900, 12.14622656770000120 ) ) ;
#9625=CYLINDRICAL_SURFACE ( 'NONE', #27523, 34.89999999999999858 ) ;
#9627=CARTESIAN_POINT ( 'NONE',  ( 40.00000000000000000, -69.50000000000000000, 2.433892081919999696E-15 ) ) ;
#9628=CARTESIAN_POINT ( 'NONE',  ( 9.356041104380000917, -84.50000000000000000, -37.60355029590000697 ) ) ;
#9631=CARTESIAN_POINT ( 'NONE',  ( -19.03577102200000226, -32.73235193859999725, 11.99443138589999869 ) ) ;
#9635=CARTESIAN_POINT ( 'NONE',  ( 25.71060173579999741, -66.29767256830000122, 0.2782536591429999318 ) ) ;
#9638=CARTESIAN_POINT ( 'NONE',  ( 9.014522480169999241, -36.52810941340000284, -21.48399575520000226 ) ) ;
#9639=CARTESIAN_POINT ( 'NONE',  ( -39.13694367224998416, -73.55869875170414218, -7.198781032002129265 ) ) ;
#9641=CARTESIAN_POINT ( 'NONE',  ( 21.75704398650000115, -37.63585108239999499, -8.427448657780001184 ) ) ;
#9644=CARTESIAN_POINT ( 'NONE',  ( 21.91842625758061303, -37.33819205718435796, -8.685017703894253316 ) ) ;
#9645=CARTESIAN_POINT ( 'NONE',  ( 46.77849477899999897, -74.12949171449999142, -3.288587074160000068 ) ) ;
#9647=B_SPLINE_SURFACE_WITH_KNOTS ( 'NONE', 5, 5, ( 
 ( #17190, #4812, #11346, #16016, #2638, #24922, #5392, #13691, #9460 ),
 ( #16159, #9157, #7148, #5099, #18215, #13980, #22889, #7448, #7291 ),
 ( #25219, #14273, #18365, #20393, #11485, #615, #4952, #26966, #25067 ),
 ( #27252, #11789, #466, #9310, #27110, #11634, #13835, #22738, #5248 ),
 ( #11933, #18506, #2777, #23031, #20548, #2927, #20701, #904, #760 ),
 ( #9746, #9606, #14133, #3081, #17630, #26818, #4658, #12937, #22445 ) ),
 .UNSPECIFIED., .F., .F., .F.,
 ( 6, 6 ),
 ( 6, 3, 6 ),
 ( 8.242378609270000211, 18.74558921099999864 ),
 ( 0.000000000000000000, 1.000000000000000000, 2.000000000000000000 ),
 .UNSPECIFIED. ) ;
#9648=CARTESIAN_POINT ( 'NONE',  ( 7.010390260919999428E-15, -84.50000000000000000, 36.25000000000000000 ) ) ;
#9650=CARTESIAN_POINT ( 'NONE',  ( -7.325370793560000315, -19.50000000000000000, -24.94672208400000102 ) ) ;
#9652=DIRECTION ( 'NONE',  ( 0.9704142011833034598, 0.000000000000000000, -0.2414462220490750377 ) ) ;
#9654=ORIENTED_EDGE ( 'NONE', *, *, #15229, .F. ) ;
#9656=CARTESIAN_POINT ( 'NONE',  ( -39.35783505871010846, -73.63371395844393419, 7.221517031003334530 ) ) ;
#9659=ORIENTED_EDGE ( 'NONE', *, *, #20031, .T. ) ;
#9660=CARTESIAN_POINT ( 'NONE',  ( -2.139909113419224074, -19.47322495657797248, -22.70449621793245498 ) ) ;
#9661=CARTESIAN_POINT ( 'NONE',  ( 1.421085471519999883E-15, -89.50000000000000000, 3.042011087470000117E-15 ) ) ;
#9662=CARTESIAN_POINT ( 'NONE',  ( -2.572067239809999961, -45.94038128989999592, -24.63225655530000324 ) ) ;
#9666=CARTESIAN_POINT ( 'NONE',  ( 21.61801161032304819, -37.04357994246159080, -8.573564458946657751 ) ) ;
#9667=DIRECTION ( 'NONE',  ( 0.000000000000000000, -1.000000000000000000, 0.000000000000000000 ) ) ;
#9668=LINE ( 'NONE', #27472, #1118 ) ;
#9669=VERTEX_POINT ( 'NONE', #8208 ) ;
#9670=CARTESIAN_POINT ( 'NONE',  ( 0.000000000000000000, -86.00000000000000000, 0.000000000000000000 ) ) ;
#9673=CARTESIAN_POINT ( 'NONE',  ( -12.68142862450000052, -66.36586770009999725, 22.39764779240000081 ) ) ;
#9674=CARTESIAN_POINT ( 'NONE',  ( 19.46718696450000152, -35.19368270689999889, -8.987515577199999939 ) ) ;
#9675=CARTESIAN_POINT ( 'NONE',  ( 23.15717220300345147, -57.99960184875410363, 10.38505609836370702 ) ) ;
#9677=FACE_OUTER_BOUND ( 'NONE', #26334, .T. ) ;
#9680=CARTESIAN_POINT ( 'NONE',  ( -8.569349526716633747, -80.50000000000000000, 38.48258446242443398 ) ) ;
#9685=EDGE_LOOP ( 'NONE', ( #1703, #27680, #20023, #14541, #9752 ) ) ;
#9687=VERTEX_POINT ( 'NONE', #10936 ) ;
#9689=CARTESIAN_POINT ( 'NONE',  ( -11.08158641716409498, -19.46474590321556875, 19.12288009785157428 ) ) ;
#9690=CARTESIAN_POINT ( 'NONE',  ( -7.241237543289999579, -73.80576217300000508, 39.53368540329999803 ) ) ;
#9692=CARTESIAN_POINT ( 'NONE',  ( -7.244026535083167850, -74.18384006180646395, -40.29424782656837323 ) ) ;
#9697=DIRECTION ( 'NONE',  ( 0.000000000000000000, -1.000000000000000000, 0.000000000000000000 ) ) ;
#9698=CARTESIAN_POINT ( 'NONE',  ( 8.810945591680001243, -22.49864585750000145, -19.93464393029999826 ) ) ;
#9699=CARTESIAN_POINT ( 'NONE',  ( -1.450349733947329467, -57.47122607689037466, -23.51019145097244234 ) ) ;
#9700=CARTESIAN_POINT ( 'NONE',  ( 20.04647669423046352, -19.46665351427041202, 9.775544613538123428 ) ) ;
#9702=ORIENTED_EDGE ( 'NONE', *, *, #18840, .F. ) ;
#9703=EDGE_CURVE ( 'NONE', #4968, #20017, #12562, .T. ) ;
#9707=CARTESIAN_POINT ( 'NONE',  ( -2.565528333990000132, -57.82174915179999886, -24.93709123049999832 ) ) ;
#9712=CIRCLE ( 'NONE', #18580, 7.249999999999999112 ) ;
#9715=CARTESIAN_POINT ( 'NONE',  ( 9.445827302050000540, -44.46958577849999728, -23.16276489379999859 ) ) ;
#9716=PLANE ( 'NONE',  #25104 ) ;
#9717=ORIENTED_EDGE ( 'NONE', *, *, #27972, .T. ) ;
#9718=CARTESIAN_POINT ( 'NONE',  ( 7.215414233289999757, -74.50000000000000000, -40.70731707320000226 ) ) ;
#9720=CARTESIAN_POINT ( 'NONE',  ( -14.65665268890000128, -79.65629807879999191, 36.94583904750000158 ) ) ;
#9721=DIRECTION ( 'NONE',  ( -0.2588190451029840911, 0.000000000000000000, -0.9659258262889440783 ) ) ;
#9722=CARTESIAN_POINT ( 'NONE',  ( -1.973996428270000214, -65.91612967349999508, -25.65258536809999868 ) ) ;
#9723=CARTESIAN_POINT ( 'NONE',  ( -16.72250540970000188, -71.11599492770000097, 23.42677820880000183 ) ) ;
#9724=ORIENTED_EDGE ( 'NONE', *, *, #12380, .T. ) ;
#9725=CYLINDRICAL_SURFACE ( 'NONE', #27904, 7.250000000000004441 ) ;
#9728=CARTESIAN_POINT ( 'NONE',  ( -21.14045977570000190, -64.47177096180000433, 15.21445029600000076 ) ) ;
#9729=ORIENTED_EDGE ( 'NONE', *, *, #10056, .T. ) ;
#9732=CARTESIAN_POINT ( 'NONE',  ( -1.179391805059999854, -18.50000000000000000, -21.01038717779999843 ) ) ;
#9733=CARTESIAN_POINT ( 'NONE',  ( 36.73205512257106875, -74.36687860487361945, -14.52407699815695352 ) ) ;
#9734=ORIENTED_EDGE ( 'NONE', *, *, #6133, .F. ) ;
#9737=AXIS2_PLACEMENT_3D ( 'NONE', #13162, #26302, #2253 ) ;
#9743=ORIENTED_EDGE ( 'NONE', *, *, #14240, .F. ) ;
#9744=EDGE_CURVE ( 'NONE', #22934, #14668, #25911, .T. ) ;
#9745=CARTESIAN_POINT ( 'NONE',  ( -11.32770615259999936, -18.50000000000000000, 18.02817438119999949 ) ) ;
#9746=CARTESIAN_POINT ( 'NONE',  ( -11.46863496399999960, -57.40875702469999453, -22.62382260229999886 ) ) ;
#9747=CARTESIAN_POINT ( 'NONE',  ( 37.22630421854149319, -79.99409917514977053, -13.87589282898977849 ) ) ;
#9748=CARTESIAN_POINT ( 'NONE',  ( 24.38889592600000000, -66.59094944230000124, -8.558251894909998825 ) ) ;
#9752=ORIENTED_EDGE ( 'NONE', *, *, #23047, .T. ) ;
#9753=CYLINDRICAL_SURFACE ( 'NONE', #19561, 4.750000000000000888 ) ;
#9755=ORIENTED_EDGE ( 'NONE', *, *, #11371, .T. ) ;
#9759=CARTESIAN_POINT ( 'NONE',  ( 38.71640869449999656, -73.50000064450000536, 7.135466578850000019 ) ) ;
#9760=CARTESIAN_POINT ( 'NONE',  ( -10.52559454271665729, -19.48499002900891952, -21.09029437625177650 ) ) ;
#9761=CARTESIAN_POINT ( 'NONE',  ( 41.00000000000000000, -80.50000000000000000, -10.20110288159999890 ) ) ;
#9762=CARTESIAN_POINT ( 'NONE',  ( -11.85777263121401859, -63.71742432004833034, -23.51471264972168385 ) ) ;
#9763=CARTESIAN_POINT ( 'NONE',  ( 47.01511379249026135, -79.64389730943054246, -2.310193425807324896 ) ) ;
#9765=DIRECTION ( 'NONE',  ( 1.000000000000000000, 0.000000000000000000, 0.000000000000000000 ) ) ;
#9772=DIRECTION ( 'NONE',  ( -0.9704142011833032377, 0.000000000000000000, -0.2414462220490753985 ) ) ;
#9773=ORIENTED_EDGE ( 'NONE', *, *, #16561, .F. ) ;
#9776=CARTESIAN_POINT ( 'NONE',  ( -20.32174609979999858, -45.92926717529999792, 14.70331994040000012 ) ) ;
#9778=CARTESIAN_POINT ( 'NONE',  ( 31.14753128929999804, -73.95999340959998847, -23.57268455550000041 ) ) ;
#9779=CARTESIAN_POINT ( 'NONE',  ( 22.51510749560000235, -60.60190586809999758, -7.150863154439999647 ) ) ;
#9782=EDGE_CURVE ( 'NONE', #11938, #6398, #28677, .T. ) ;
#9783=CARTESIAN_POINT ( 'NONE',  ( 25.83227502339999759, -65.33654462470001079, 1.152172478150000012 ) ) ;
#9787=FACE_OUTER_BOUND ( 'NONE', #3590, .T. ) ;
#9788=CARTESIAN_POINT ( 'NONE',  ( 21.54641223700000197, -36.98696877929999260, -8.488506496170000304 ) ) ;
#9790=ORIENTED_EDGE ( 'NONE', *, *, #28443, .F. ) ;
#9791=LINE ( 'NONE', #6230, #12928 ) ;
#9795=CARTESIAN_POINT ( 'NONE',  ( 9.295214654649997854, -36.51121532460000196, -22.62696043789999933 ) ) ;
#9798=ORIENTED_EDGE ( 'NONE', *, *, #16973, .T. ) ;
#9799=CARTESIAN_POINT ( 'NONE',  ( -40.20585889361907306, -74.11886065923714284, 7.247546674747338713 ) ) ;
#9801=CARTESIAN_POINT ( 'NONE',  ( -13.31718154921655817, -19.49371677639106792, 20.06828757285913056 ) ) ;
#9804=CARTESIAN_POINT ( 'NONE',  ( 19.39131233670000043, -19.49132065570000094, -8.982198477279998983 ) ) ;
#9806=CARTESIAN_POINT ( 'NONE',  ( -1.560217637240000066, -26.09432050500000244, -22.44965361090000044 ) ) ;
#9808=EDGE_CURVE ( 'NONE', #8240, #16034, #20444, .T. ) ;
#9809=ADVANCED_FACE ( 'NONE', ( #7337 ), #25618, .T. ) ;
#9810=CARTESIAN_POINT ( 'NONE',  ( 40.70731707320000226, -84.00000000000000000, -7.215414233289999757 ) ) ;
#9811=DIRECTION ( 'NONE',  ( 1.000000000000000000, 0.000000000000000000, 0.000000000000000000 ) ) ;
#9816=CARTESIAN_POINT ( 'NONE',  ( -32.66023292530000077, -74.50000000430000568, -21.85457041679999790 ) ) ;
#9818=AXIS2_PLACEMENT_3D ( 'NONE', #26292, #8351, #17687 ) ;
#9820=CIRCLE ( 'NONE', #1022, 3.000000000000002665 ) ;
#9823=CARTESIAN_POINT ( 'NONE',  ( 21.05852219120000157, -34.60505771119999707, -8.113043137870000976 ) ) ;
#9824=CARTESIAN_POINT ( 'NONE',  ( 7.230541818635105145, -73.67850591074257238, 39.46631086800589827 ) ) ;
#9825=TOROIDAL_SURFACE ( 'NONE', #12149, 3.500000000000000000, 0.5000000000000000000 ) ;
#9833=DIRECTION ( 'NONE',  ( -1.203338504109999799E-16, -0.000000000000000000, -1.000000000000000000 ) ) ;
#9835=LINE ( 'NONE', #18743, #22944 ) ;
#9837=CARTESIAN_POINT ( 'NONE',  ( -7.448397597250000501, -73.97429387040000393, 38.88881331079999626 ) ) ;
#9843=EDGE_CURVE ( 'NONE', #5725, #23453, #14109, .T. ) ;
#9844=AXIS2_PLACEMENT_3D ( 'NONE', #25594, #566, #16111 ) ;
#9845=CARTESIAN_POINT ( 'NONE',  ( 11.52668943299999960, -72.21526968880000652, -27.03296487709999951 ) ) ;
#9847=FACE_OUTER_BOUND ( 'NONE', #26862, .T. ) ;
#9848=CARTESIAN_POINT ( 'NONE',  ( -5.679770007689999289, -80.00000000000000000, 46.75000000000000000 ) ) ;
#9850=DIRECTION ( 'NONE',  ( 0.000000000000000000, -1.000000000000000000, 0.000000000000000000 ) ) ;
#9852=CARTESIAN_POINT ( 'NONE',  ( 9.469927264672032052, -36.00000000000000000, -20.04523765350436904 ) ) ;
#9855=CARTESIAN_POINT ( 'NONE',  ( -2.351527211430000097, -58.27079767440000069, -24.37373320010000199 ) ) ;
#9861=LINE ( 'NONE', #5063, #4703 ) ;
#9867=FACE_OUTER_BOUND ( 'NONE', #17380, .T. ) ;
#9869=CARTESIAN_POINT ( 'NONE',  ( -14.22861760630000028, -68.06112540870000771, 22.55404134810000016 ) ) ;
#9873=CARTESIAN_POINT ( 'NONE',  ( 24.53756381369999673, -63.58862135099999335, 0.03861512792729999977 ) ) ;
#9876=CARTESIAN_POINT ( 'NONE',  ( -18.78219790299999659, -19.46510053389999939, 11.52011550950000007 ) ) ;
#9877=CIRCLE ( 'NONE', #26626, 7.249999999999999112 ) ;
#9878=CARTESIAN_POINT ( 'NONE',  ( 18.88171271891879854, -18.49999999999998224, -8.341252403918135272 ) ) ;
#9881=FACE_OUTER_BOUND ( 'NONE', #860, .T. ) ;
#9883=CARTESIAN_POINT ( 'NONE',  ( -12.24789267329999909, -65.07443093669999712, 21.96586363990000024 ) ) ;
#9884=ORIENTED_EDGE ( 'NONE', *, *, #22784, .F. ) ;
#9885=B_SPLINE_SURFACE_WITH_KNOTS ( 'NONE', 5, 5, ( 
 ( #8422, #26220, #4057, #12923, #1615, #24024 ),
 ( #8156, #21840, #1893, #10731, #8571, #10879 ),
 ( #17475, #28669, #19231, #14711, #28119, #25933 ),
 ( #23743, #13821, #26808, #11475, #20381, #11018 ),
 ( #6543, #19932, #4940, #17915, #6840, #15705 ),
 ( #20092, #17617, #15406, #6992, #4359, #451 ),
 ( #16005, #9009, #24611, #22727, #6, #15856 ),
 ( #7138, #9300, #18201, #22583, #24766, #4648 ),
 ( #22435, #13374, #155, #603, #9148, #4499 ) ),
 .UNSPECIFIED., .F., .F., .F.,
 ( 6, 3, 6 ),
 ( 6, 6 ),
 ( 1.594447291550000054E-15, 2.252774941530000241, 5.576981603840000190 ),
 ( 0.000000000000000000, 1.000000000000000000 ),
 .UNSPECIFIED. ) ;
#9886=FACE_OUTER_BOUND ( 'NONE', #14794, .T. ) ;
#9887=CYLINDRICAL_SURFACE ( 'NONE', #5935, 0.5000000000000004441 ) ;
#9888=ORIENTED_EDGE ( 'NONE', *, *, #2963, .F. ) ;
#9889=CARTESIAN_POINT ( 'NONE',  ( 47.25006817639999923, -74.77883526400000846, -0.5535757861789999401 ) ) ;
#9894=VERTEX_POINT ( 'NONE', #9648 ) ;
#9895=EDGE_CURVE ( 'NONE', #19383, #10333, #1225, .T. ) ;
#9899=B_SPLINE_CURVE_WITH_KNOTS ( 'NONE', 5,
 ( #11369, #9336, #24499, #4532, #20273, #25094 ),
 .UNSPECIFIED., .F., .F.,
 ( 6, 6 ),
 ( 0.000000000000000000, 1.000000000000000000 ),
 .UNSPECIFIED. ) ;
#9900=CARTESIAN_POINT ( 'NONE',  ( 39.96405812750000308, -74.08838618730000292, 7.268564243930000224 ) ) ;
#9908=CARTESIAN_POINT ( 'NONE',  ( -32.64087606319999679, -79.95649630820000198, -22.33050332599999876 ) ) ;
#9913=CARTESIAN_POINT ( 'NONE',  ( -0.7591504320660000804, -79.66564775870000403, 47.25050659409999554 ) ) ;
#9915=ORIENTED_EDGE ( 'NONE', *, *, #10325, .F. ) ;
#9916=DIRECTION ( 'NONE',  ( 0.000000000000000000, -1.000000000000000000, 0.000000000000000000 ) ) ;
#9917=CARTESIAN_POINT ( 'NONE',  ( 0.000000000000000000, -56.78056608349999834, 0.000000000000000000 ) ) ;
#9919=CARTESIAN_POINT ( 'NONE',  ( 27.75394116159999669, -74.50000000000000000, -27.75394116159999669 ) ) ;
#9920=CARTESIAN_POINT ( 'NONE',  ( -14.49490684773424931, -74.10099149224471660, 36.26165015395787350 ) ) ;
#9925=CIRCLE ( 'NONE', #18794, 39.25000000000000000 ) ;
#9926=CARTESIAN_POINT ( 'NONE',  ( 20.58520128069999799, -36.04995792020000067, -8.980828480690000504 ) ) ;
#9927=DIRECTION ( 'NONE',  ( 0.9387128607161809857, 0.000000000000000000, 0.3447001089730665768 ) ) ;
#9930=ADVANCED_FACE ( 'NONE', ( #3395 ), #8379, .F. ) ;
#9931=CARTESIAN_POINT ( 'NONE',  ( -21.10814673583525902, -64.47177029419442817, 15.24425173043963966 ) ) ;
#9935=FACE_OUTER_BOUND ( 'NONE', #1468, .T. ) ;
#9937=EDGE_CURVE ( 'NONE', #12917, #2214, #7817, .T. ) ;
#9939=CARTESIAN_POINT ( 'NONE',  ( 24.05376935019999962, -19.40595403639999716, 1.523939926209999962 ) ) ;
#9940=CARTESIAN_POINT ( 'NONE',  ( -12.99499290521388595, -19.48483198002087491, 19.65355774919085263 ) ) ;
#9941=CARTESIAN_POINT ( 'NONE',  ( 23.19910953469999981, -45.76350410940000302, -9.457696755039998848 ) ) ;
#9942=ORIENTED_EDGE ( 'NONE', *, *, #16399, .T. ) ;
#9943=CARTESIAN_POINT ( 'NONE',  ( 19.61724684530000218, -18.50000000000000000, -7.593153726179999730 ) ) ;
#9945=CARTESIAN_POINT ( 'NONE',  ( -0.8962089411180000909, -26.09894693429999890, -22.24995341260000359 ) ) ;
#9948=FACE_OUTER_BOUND ( 'NONE', #18726, .T. ) ;
#9950=CARTESIAN_POINT ( 'NONE',  ( 20.06309763089999620, -36.00000000000000000, -9.476129751679998492 ) ) ;
#9953=ORIENTED_EDGE ( 'NONE', *, *, #23090, .T. ) ;
#9954=B_SPLINE_CURVE_WITH_KNOTS ( 'NONE', 5,
 ( #13261, #4678, #13857, #24352, #22312, #24649, #22762, #18085, #24798, #24495, #20417, #2509 ),
 .UNSPECIFIED., .F., .F.,
 ( 6, 3, 3, 6 ),
 ( 0.000000000000000000, 0.2674763062605450825, 0.5735529784659251229, 1.000000000000000000 ),
 .UNSPECIFIED. ) ;
#9956=CARTESIAN_POINT ( 'NONE',  ( -21.71458329359999695, -74.50000000000000000, -32.69645379630000548 ) ) ;
#9958=CARTESIAN_POINT ( 'NONE',  ( 7.882323183639998732, -36.30033153219999775, -21.44286902610000212 ) ) ;
#9961=CARTESIAN_POINT ( 'NONE',  ( 23.52622212079999997, -57.40875702419999982, -9.564509902230000193 ) ) ;
#9962=CARTESIAN_POINT ( 'NONE',  ( -13.66168260340000096, -74.00000000000000000, -27.27344781959999764 ) ) ;
#9963=DIRECTION ( 'NONE',  ( -0.1038897333389494221, 0.000000000000000000, -0.9945888212255162841 ) ) ;
#9966=ORIENTED_EDGE ( 'NONE', *, *, #21108, .F. ) ;
#9968=DIRECTION ( 'NONE',  ( 0.1166882174331227151, -0.3326668106479456766, -0.9357973354341229122 ) ) ;
#9971=CARTESIAN_POINT ( 'NONE',  ( 26.38214758550000028, -68.90972672860000614, -11.00107854260000018 ) ) ;
#9972=EDGE_CURVE ( 'NONE', #10466, #321, #16310, .T. ) ;
#9974=CARTESIAN_POINT ( 'NONE',  ( -7.263337524479998919, -73.89694774980000602, 39.48646518750000212 ) ) ;
#9978=CARTESIAN_POINT ( 'NONE',  ( 21.93491260069999882, -72.48668981500000541, -30.95810316469999890 ) ) ;
#9979=CARTESIAN_POINT ( 'NONE',  ( -22.80702985319999954, -71.67701549839999586, 16.52030771659999786 ) ) ;
#9981=CIRCLE ( 'NONE', #7217, 23.36116116979999902 ) ;
#9983=CARTESIAN_POINT ( 'NONE',  ( 8.815774981519998832, -19.46527873000000142, -19.82451640119999681 ) ) ;
#9993=EDGE_CURVE ( 'NONE', #25766, #23252, #5977, .T. ) ;
#9995=CARTESIAN_POINT ( 'NONE',  ( -7.135467304789999687, -73.50000064450000536, 38.71640881029999548 ) ) ;
#9996=CARTESIAN_POINT ( 'NONE',  ( -7.315286554515622264, -74.28332971673216889, -40.00438978215803587 ) ) ;
#9997=VERTEX_POINT ( 'NONE', #6407 ) ;
#9999=CARTESIAN_POINT ( 'NONE',  ( 7.954809540590000339, -36.56645929769999981, -21.41760928989999968 ) ) ;
#10003=CARTESIAN_POINT ( 'NONE',  ( -13.80673663610000013, -68.20222181140000828, 22.71145995190000377 ) ) ;
#10005=DIRECTION ( 'NONE',  ( 1.000000000000000000, 0.000000000000000000, 0.000000000000000000 ) ) ;
#10007=CARTESIAN_POINT ( 'NONE',  ( 23.80217619240000104, -60.55397095009999475, 0.3124424936219999949 ) ) ;
#10008=CARTESIAN_POINT ( 'NONE',  ( -20.01779683490000039, -60.59309307459999872, 12.54531749399999896 ) ) ;
#10010=CARTESIAN_POINT ( 'NONE',  ( 24.31832408829999892, -64.48635707210000589, -9.855635234570000236 ) ) ;
#10011=CARTESIAN_POINT ( 'NONE',  ( 18.94592261899999741, -19.50000000000000000, -9.024080787800000891 ) ) ;
#10013=ORIENTED_EDGE ( 'NONE', *, *, #10404, .F. ) ;
#10014=EDGE_CURVE ( 'NONE', #10287, #3233, #5020, .T. ) ;
#10018=CARTESIAN_POINT ( 'NONE',  ( 36.62206425559999445, -80.26271606740000664, -14.12235947189999941 ) ) ;
#10019=FACE_OUTER_BOUND ( 'NONE', #4471, .T. ) ;
#10021=ADVANCED_FACE ( 'NONE', ( #23256 ), #18260, .T. ) ;
#10023=CARTESIAN_POINT ( 'NONE',  ( 10.00000000000000000, -19.00000000000000000, 0.000000000000000000 ) ) ;
#10024=ORIENTED_EDGE ( 'NONE', *, *, #25799, .T. ) ;
#10025=CARTESIAN_POINT ( 'NONE',  ( 46.37168807673121762, -73.60877760474707543, -3.458991447863533963 ) ) ;
#10027=CARTESIAN_POINT ( 'NONE',  ( -13.26444742760000040, -34.62271398969999581, 20.17275320750000134 ) ) ;
#10029=EDGE_LOOP ( 'NONE', ( #15675, #3901, #3803, #11032 ) ) ;
#10031=EDGE_LOOP ( 'NONE', ( #18784, #13387, #22150, #4178, #16109, #4119, #7280 ) ) ;
#10032=CARTESIAN_POINT ( 'NONE',  ( 38.65569830309999588, -74.00000023179998720, 7.472969336320000266 ) ) ;
#10034=CARTESIAN_POINT ( 'NONE',  ( -11.80701538218819913, -63.17441371568864383, -23.36682876523914842 ) ) ;
#10035=CARTESIAN_POINT ( 'NONE',  ( 46.83762086372372124, -79.80981178139894894, -3.035625116143169322 ) ) ;
#10036=ORIENTED_EDGE ( 'NONE', *, *, #28003, .F. ) ;
#10037=CARTESIAN_POINT ( 'NONE',  ( -32.35914374060000398, -80.34842067969999846, -22.21527698039999876 ) ) ;
#10040=ORIENTED_EDGE ( 'NONE', *, *, #19423, .F. ) ;
#10042=FACE_OUTER_BOUND ( 'NONE', #24546, .T. ) ;
#10044=ORIENTED_EDGE ( 'NONE', *, *, #7964, .T. ) ;
#10048=CARTESIAN_POINT ( 'NONE',  ( 30.92226875830000310, -72.24519481100000462, -21.98812938469999878 ) ) ;
#10050=CARTESIAN_POINT ( 'NONE',  ( -15.34661535209604644, -72.13193952715772639, 23.85822615002545888 ) ) ;
#10051=EDGE_CURVE ( 'NONE', #4550, #14431, #4192, .T. ) ;
#10052=B_SPLINE_CURVE_WITH_KNOTS ( 'NONE', 5,
 ( #10186, #10324, #8163, #17049, #23750, #1622 ),
 .UNSPECIFIED., .F., .F.,
 ( 6, 6 ),
 ( 0.000000000000000000, 1.000000000000000000 ),
 .UNSPECIFIED. ) ;
#10053=B_SPLINE_SURFACE_WITH_KNOTS ( 'NONE', 5, 5, ( 
 ( #654, #9060, #11072, #26856, #15762, #2821 ),
 ( #19990, #9201, #7193, #510, #11531, #22489 ),
 ( #6897, #24668, #4701, #11386, #20288, #18114 ),
 ( #27006, #7045, #15912, #24818, #4857, #9356 ),
 ( #18257, #27153, #11681, #9506, #25114, #5144 ),
 ( #14026, #5939, #25403, #16355, #17162, #8140 ) ),
 .UNSPECIFIED., .F., .F., .F.,
 ( 6, 6 ),
 ( 6, 6 ),
 ( 2.788355763089999773, 6.107000906319999700 ),
 ( 0.000000000000000000, 0.5000000000000000000 ),
 .UNSPECIFIED. ) ;
#10054=EDGE_CURVE ( 'NONE', #16224, #12521, #8870, .T. ) ;
#10055=B_SPLINE_CURVE_WITH_KNOTS ( 'NONE', 5,
 ( #7425, #5378, #5651, #5232, #23016, #18641, #18922, #3335, #21245 ),
 .UNSPECIFIED., .F., .F.,
 ( 6, 3, 6 ),
 ( -1.134864905219999942, -0.9962660581400000215, 0.000000000000000000 ),
 .UNSPECIFIED. ) ;
#10056=EDGE_CURVE ( 'NONE', #25273, #6167, #18237, .T. ) ;
#10058=CARTESIAN_POINT ( 'NONE',  ( 8.883150714079999233, -37.96517267130000306, -22.08524768410000050 ) ) ;
#10059=CARTESIAN_POINT ( 'NONE',  ( 20.01429411540000203, -35.44265700830000299, -8.963580768409999067 ) ) ;
#10060=CARTESIAN_POINT ( 'NONE',  ( 21.16092811309999888, -36.40219747150000273, -8.702541777570001358 ) ) ;
#10062=ORIENTED_EDGE ( 'NONE', *, *, #17974, .T. ) ;
#10068=ORIENTED_EDGE ( 'NONE', *, *, #17432, .T. ) ;
#10071=CARTESIAN_POINT ( 'NONE',  ( -10.20110288159999890, -84.00000000000000000, -41.00000000000000000 ) ) ;
#10072=ORIENTED_EDGE ( 'NONE', *, *, #4415, .T. ) ;
#10074=B_SPLINE_CURVE_WITH_KNOTS ( 'NONE', 5,
 ( #10011, #7722, #27805, #16877, #9878, #7847 ),
 .UNSPECIFIED., .F., .F.,
 ( 6, 6 ),
 ( 0.000000000000000000, 1.000000000000000000 ),
 .UNSPECIFIED. ) ;
#10075=CARTESIAN_POINT ( 'NONE',  ( -14.51516215540000054, -74.22762369209999633, 36.44028598479999914 ) ) ;
#10076=CARTESIAN_POINT ( 'NONE',  ( -14.94461375770000089, -74.50000000000000000, 45.97940633559999668 ) ) ;
#10077=CARTESIAN_POINT ( 'NONE',  ( -16.86265888959999870, -74.50000000000000000, 45.21850545039999503 ) ) ;
#10078=B_SPLINE_CURVE_WITH_KNOTS ( 'NONE', 5,
 ( #23156, #600, #27385, #20379, #3068, #9876 ),
 .UNSPECIFIED., .F., .F.,
 ( 6, 6 ),
 ( 0.000000000000000000, 46.92787229080000344 ),
 .UNSPECIFIED. ) ;
#10079=DIRECTION ( 'NONE',  ( 0.000000000000000000, -1.000000000000000000, 0.000000000000000000 ) ) ;
#10082=CARTESIAN_POINT ( 'NONE',  ( -10.97670906379999956, -34.61119146809999592, -21.88132632449999804 ) ) ;
#10084=EDGE_CURVE ( 'NONE', #19884, #13409, #27277, .T. ) ;
#10088=EDGE_CURVE ( 'NONE', #6300, #2641, #24099, .T. ) ;
#10089=CARTESIAN_POINT ( 'NONE',  ( 10.00000000000000000, -42.50000000000000000, -2.449212707639999657E-15 ) ) ;
#10090=CARTESIAN_POINT ( 'NONE',  ( 8.408940298639999256, -35.33620340770000468, -20.95510887249999854 ) ) ;
#10091=CARTESIAN_POINT ( 'NONE',  ( 7.221517031000784570, -73.63371395842501954, 39.35783505868155174 ) ) ;
#10093=DIRECTION ( 'NONE',  ( 0.000000000000000000, -1.000000000000000000, 0.000000000000000000 ) ) ;
#10096=CARTESIAN_POINT ( 'NONE',  ( 10.33698150750000089, -74.00000000000000000, -28.69894320070000049 ) ) ;
#10097=CYLINDRICAL_SURFACE ( 'NONE', #23673, 11.00000000000000000 ) ;
#10098=ORIENTED_EDGE ( 'NONE', *, *, #8897, .T. ) ;
#10102=DIRECTION ( 'NONE',  ( 1.000000000000000000, 0.000000000000000000, 0.000000000000000000 ) ) ;
#10103=FACE_OUTER_BOUND ( 'NONE', #21192, .T. ) ;
#10104=CARTESIAN_POINT ( 'NONE',  ( 10.50000000000000000, -89.50000000000000000, 0.000000000000000000 ) ) ;
#10105=CARTESIAN_POINT ( 'NONE',  ( 26.50110885399999816, -74.25067683309998756, -29.00949035939999732 ) ) ;
#10106=DIRECTION ( 'NONE',  ( 0.000000000000000000, -1.000000000000000000, 0.000000000000000000 ) ) ;
#10107=B_SPLINE_SURFACE_WITH_KNOTS ( 'NONE', 5, 5, ( 
 ( #27661, #22698, #9421, #16566, #18328, #16123, #13947, #16850, #12732 ),
 ( #25743, #15061, #16702, #14923, #3453, #1419, #12320, #14784, #23685 ),
 ( #28196, #23970, #1560, #12180, #10403, #8229, #1153, #17125, #4985 ),
 ( #4147, #18404, #7040, #20436, #22083, #10964, #1835, #28755, #28481 ),
 ( #18108, #22630, #6333, #24113, #1982, #10825, #8653, #6483, #10058 ),
 ( #7487, #14583, #7899, #3524, #9638, #27593, #21027, #5426, #10193 ) ),
 .UNSPECIFIED., .F., .F., .F.,
 ( 6, 6 ),
 ( 6, 3, 6 ),
 ( 0.000000000000000000, 2.709627183969999908 ),
 ( 0.000000000000000000, 1.000000000000000000, 2.000000000000000000 ),
 .UNSPECIFIED. ) ;
#10111=CARTESIAN_POINT ( 'NONE',  ( -2.565530488236128726, -57.41946962537819843, -24.92670969134982073 ) ) ;
#10113=ORIENTED_EDGE ( 'NONE', *, *, #18813, .F. ) ;
#10115=DIRECTION ( 'NONE',  ( 0.000000000000000000, -1.000000000000000000, 0.000000000000000000 ) ) ;
#10119=CARTESIAN_POINT ( 'NONE',  ( -33.25000000000000000, -69.00000000000000000, 2.267215112510000273E-15 ) ) ;
#10121=DIRECTION ( 'NONE',  ( 0.4794255386042036715, 0.000000000000000000, 0.8775825618903724257 ) ) ;
#10122=AXIS2_PLACEMENT_3D ( 'NONE', #8125, #3482, #23164 ) ;
#10125=EDGE_LOOP ( 'NONE', ( #22521, #13197 ) ) ;
#10127=ORIENTED_EDGE ( 'NONE', *, *, #9166, .F. ) ;
#10129=CARTESIAN_POINT ( 'NONE',  ( 9.079731074819999748, -35.79879667440000190, -19.54912311329999852 ) ) ;
#10131=CARTESIAN_POINT ( 'NONE',  ( -14.93121042630000161, -79.81259640750000983, 36.29905572410000048 ) ) ;
#10134=CARTESIAN_POINT ( 'NONE',  ( -22.19162232541316726, -74.22311029766915169, -32.68008730919952853 ) ) ;
#10135=ORIENTED_EDGE ( 'NONE', *, *, #27228, .T. ) ;
#10138=CARTESIAN_POINT ( 'NONE',  ( -32.38119801256480201, -74.06990842591031310, -22.11895758288902769 ) ) ;
#10139=CARTESIAN_POINT ( 'NONE',  ( -21.43329106970000453, -64.24504445130001784, 15.59675033660000132 ) ) ;
#10141=CARTESIAN_POINT ( 'NONE',  ( -40.00000000000000000, -79.00000000000000000, 0.000000000000000000 ) ) ;
#10142=CARTESIAN_POINT ( 'NONE',  ( -2.433604254030000025, -18.85965710059999978, -22.72529456070000009 ) ) ;
#10144=VERTEX_POINT ( 'NONE', #4821 ) ;
#10146=EDGE_CURVE ( 'NONE', #21742, #10192, #27938, .T. ) ;
#10149=CARTESIAN_POINT ( 'NONE',  ( 36.70830968599999977, -79.18133521899999039, -14.75000000000000000 ) ) ;
#10150=EDGE_LOOP ( 'NONE', ( #1130, #15266, #17117 ) ) ;
#10151=EDGE_CURVE ( 'NONE', #14119, #3822, #28397, .T. ) ;
#10155=CARTESIAN_POINT ( 'NONE',  ( -1.962472190547156492, -80.20444909203943951, 46.98144082036905900 ) ) ;
#10157=CARTESIAN_POINT ( 'NONE',  ( 46.35917536702522312, -73.60349922462170014, -3.481876491973060705 ) ) ;
#10158=EDGE_LOOP ( 'NONE', ( #11623, #13094, #17011, #5035, #1607 ) ) ;
#10159=CARTESIAN_POINT ( 'NONE',  ( 23.14416696800000040, -57.40875702389999446, 10.37855829579999778 ) ) ;
#10163=CARTESIAN_POINT ( 'NONE',  ( 22.97877291159999658, -37.99999999279999230, -9.393614097370001303 ) ) ;
#10164=ADVANCED_FACE ( 'NONE', ( #19946 ), #14081, .T. ) ;
#10165=AXIS2_PLACEMENT_3D ( 'NONE', #8404, #17025, #11832 ) ;
#10166=CARTESIAN_POINT ( 'NONE',  ( 40.32207487400000190, -74.31847293620000983, 7.253641904880000268 ) ) ;
#10167=CARTESIAN_POINT ( 'NONE',  ( 8.748807886850000770, -36.72219091139999847, -21.64960688639999731 ) ) ;
#10168=CARTESIAN_POINT ( 'NONE',  ( 19.36781163719999910, -19.46510053389999939, 10.50580276810000058 ) ) ;
#10169=CARTESIAN_POINT ( 'NONE',  ( 9.719900652158303345, -61.18767182266058313, -23.95297974322888024 ) ) ;
#10171=VECTOR ( 'NONE', #6723, 1000.000000000000114 ) ;
#10172=AXIS2_PLACEMENT_3D ( 'NONE', #26983, #2507, #11210 ) ;
#10173=DIRECTION ( 'NONE',  ( 1.000000000000000000, 0.000000000000000000, 0.000000000000000000 ) ) ;
#10176=CARTESIAN_POINT ( 'NONE',  ( -2.566493094860000213, -53.78538132969999452, -24.83346198079999922 ) ) ;
#10177=CIRCLE ( 'NONE', #20916, 0.4999999999999982236 ) ;
#10183=DIRECTION ( 'NONE',  ( 1.000000000000000000, 0.000000000000000000, 0.000000000000000000 ) ) ;
#10184=B_SPLINE_CURVE_WITH_KNOTS ( 'NONE', 3,
 ( #5265, #1327, #20861, #920, #5120, #3367, #2945, #10169, #27271, #7308, #22907, #21001 ),
 .UNSPECIFIED., .F., .F.,
 ( 4, 2, 2, 2, 2, 4 ),
 ( 0.000000000000000000, 0.2500000000000004996, 0.3750000000000007772, 0.4375000000000008882, 0.5000000000000009992, 1.000000000000000000 ),
 .UNSPECIFIED. ) ;
#10185=CARTESIAN_POINT ( 'NONE',  ( 31.74621573099999949, -73.74045749030000252, -21.89553964419999943 ) ) ;
#10186=CARTESIAN_POINT ( 'NONE',  ( 20.30102379280000235, -72.00000000000000000, -30.97095677779999789 ) ) ;
#10187=B_SPLINE_CURVE_WITH_KNOTS ( 'NONE', 3,
 ( #17708, #20026, #26594, #94, #17852, #26750, #4589, #13464, #11269, #249, #17995, #6930, #15793, #18876, #11715, #3424, #12289, #20777, #21062, #18440, #25144, #14623, #7671, #23243, #9824, #21198, #10091, #7368, #5741, #16670, #11866, #25434, #1121 ),
 .UNSPECIFIED., .F., .F.,
 ( 4, 2, 2, 1, 1, 1, 2, 2, 2, 1, 1, 1, 2, 2, 2, 1, 1, 1, 2, 2, 4 ),
 ( 0.000000000000000000, 0.1250000000005699607, 0.1875000000008528733, 0.2187500000009991175, 0.2343750000010775270, 0.2421875000011083912, 0.2460937500011094736, 0.2500000000011105561, 0.3750000000008985035, 0.4375000000007871481, 0.4687500000007259193, 0.4843750000006953327, 0.4921875000006845635, 0.5000000000006737944, 0.6250000000004710676, 0.6875000000003697043, 0.7187500000003232969, 0.7343750000002956524, 0.7421875000002818856, 0.7500000000002680078, 1.000000000000000000 ),
 .UNSPECIFIED. ) ;
#10189=DIRECTION ( 'NONE',  ( 0.000000000000000000, -1.000000000000000000, 0.000000000000000000 ) ) ;
#10192=VERTEX_POINT ( 'NONE', #13842 ) ;
#10193=CARTESIAN_POINT ( 'NONE',  ( 8.677144177649999790, -37.95796631159999635, -21.92880660069999976 ) ) ;
#10194=CARTESIAN_POINT ( 'NONE',  ( 21.23424077079999961, -35.30313508829999591, -7.936588796080000563 ) ) ;
#10195=CARTESIAN_POINT ( 'NONE',  ( 21.41729796960000343, -36.56372031789999966, -7.953963089449999302 ) ) ;
#10196=CARTESIAN_POINT ( 'NONE',  ( -21.60034894820000062, -79.50000026560000776, -32.77174736439999947 ) ) ;
#10197=EDGE_LOOP ( 'NONE', ( #4455, #14921, #14855, #19599 ) ) ;
#10199=ADVANCED_FACE ( 'NONE', ( #3220 ), #9753, .T. ) ;
#10210=ORIENTED_EDGE ( 'NONE', *, *, #27116, .T. ) ;
#10211=CARTESIAN_POINT ( 'NONE',  ( -13.82310862920000005, -74.00000000000000000, 36.20061004769999613 ) ) ;
#10212=ADVANCED_FACE ( 'NONE', ( #9468 ), #24774, .F. ) ;
#10214=CARTESIAN_POINT ( 'NONE',  ( -14.65665286289999969, -74.50000000000000000, 36.94583910070000599 ) ) ;
#10216=DIRECTION ( 'NONE',  ( 0.000000000000000000, 1.000000000000000000, 0.000000000000000000 ) ) ;
#10219=VECTOR ( 'NONE', #12990, 1000.000000000000000 ) ;
#10220=DIRECTION ( 'NONE',  ( -1.000000000000000000, 0.000000000000000000, -7.486357007659997978E-17 ) ) ;
#10222=CARTESIAN_POINT ( 'NONE',  ( 9.613588401009998563, -61.68639133699999633, -23.70244304940000291 ) ) ;
#10224=CARTESIAN_POINT ( 'NONE',  ( 22.56940943720000092, -57.43018231299999599, 10.15711860900000119 ) ) ;
#10225=DIRECTION ( 'NONE',  ( -1.000000000000000000, 0.000000000000000000, 0.000000000000000000 ) ) ;
#10230=DIRECTION ( 'NONE',  ( 0.000000000000000000, -1.000000000000000000, 0.000000000000000000 ) ) ;
#10237=CARTESIAN_POINT ( 'NONE',  ( 21.05852160050000066, -34.60505674910000096, -8.113043604739999637 ) ) ;
#10239=LINE ( 'NONE', #24083, #2686 ) ;
#10243=CARTESIAN_POINT ( 'NONE',  ( 7.215414233289999757, -74.50000000000000000, -40.70731707320000226 ) ) ;
#10244=EDGE_CURVE ( 'NONE', #24813, #4093, #25868, .T. ) ;
#10248=DIRECTION ( 'NONE',  ( 1.000000000000000000, 0.000000000000000000, 0.000000000000000000 ) ) ;
#10249=ADVANCED_FACE ( 'NONE', ( #20362 ), #13508, .T. ) ;
#10250=CARTESIAN_POINT ( 'NONE',  ( 26.48637309549999941, -74.30622060240000337, -29.02318743760000075 ) ) ;
#10251=ADVANCED_FACE ( 'NONE', ( #18181 ), #27669, .T. ) ;
#10253=DIRECTION ( 'NONE',  ( 0.000000000000000000, -1.000000000000000000, 0.000000000000000000 ) ) ;
#10254=FACE_OUTER_BOUND ( 'NONE', #20944, .T. ) ;
#10257=VERTEX_POINT ( 'NONE', #24890 ) ;
#10258=AXIS2_PLACEMENT_3D ( 'NONE', #26369, #17628, #21999 ) ;
#10260=CIRCLE ( 'NONE', #4704, 34.89999999999999858 ) ;
#10262=EDGE_LOOP ( 'NONE', ( #11078, #11466, #12908, #2782 ) ) ;
#10263=CARTESIAN_POINT ( 'NONE',  ( -0.9108550417630000284, -62.96338283689998860, -24.26276433549999823 ) ) ;
#10265=CARTESIAN_POINT ( 'NONE',  ( 20.95510892579999762, -35.33620225780000368, -8.408939989400000314 ) ) ;
#10267=CARTESIAN_POINT ( 'NONE',  ( 21.43354447929999651, -35.82074273779999629, -7.316573576590000627 ) ) ;
#10269=AXIS2_PLACEMENT_3D ( 'NONE', #11990, #16946, #7783 ) ;
#10270=CARTESIAN_POINT ( 'NONE',  ( 7.635730262653531497, -37.29149436589506195, -21.50724729230068988 ) ) ;
#10271=CIRCLE ( 'NONE', #6574, 2.500000000000000444 ) ;
#10274=AXIS2_PLACEMENT_3D ( 'NONE', #11347, #13091, #22288 ) ;
#10275=CARTESIAN_POINT ( 'NONE',  ( -14.66608889819999995, -79.71516998469999749, 36.47374630150000030 ) ) ;
#10276=CARTESIAN_POINT ( 'NONE',  ( 10.20110288159999890, -84.00000000000000000, 41.00000000000000000 ) ) ;
#10277=EDGE_CURVE ( 'NONE', #14992, #14960, #9861, .T. ) ;
#10280=CARTESIAN_POINT ( 'NONE',  ( -32.82503636037260719, -74.41293640438078683, -22.22642620204530672 ) ) ;
#10283=CARTESIAN_POINT ( 'NONE',  ( -47.25000000000000000, -69.50000000000000000, 3.352534721190000231E-15 ) ) ;
#10285=CARTESIAN_POINT ( 'NONE',  ( -2.591557398349999985, -19.17414499179999865, -23.45736093650000242 ) ) ;
#10287=VERTEX_POINT ( 'NONE', #25187 ) ;
#10289=CARTESIAN_POINT ( 'NONE',  ( -31.99425276130000384, -74.00000000020000357, -21.99785695679999975 ) ) ;
#10290=CARTESIAN_POINT ( 'NONE',  ( 7.196178079599999222, -73.81415926540000783, 38.70548889989999708 ) ) ;
#10291=ORIENTED_EDGE ( 'NONE', *, *, #25646, .T. ) ;
#10294=CARTESIAN_POINT ( 'NONE',  ( 40.00000000000000000, -73.50000000000000000, 2.065014825799999939E-15 ) ) ;
#10295=CARTESIAN_POINT ( 'NONE',  ( -2.570879204283450736, -80.36838817132422719, 46.77903939411709189 ) ) ;
#10298=VERTEX_POINT ( 'NONE', #582 ) ;
#10301=CARTESIAN_POINT ( 'NONE',  ( -7.260205543919999727, -73.74944613220000633, -39.69269201139999836 ) ) ;
#10304=DIRECTION ( 'NONE',  ( 0.000000000000000000, -1.000000000000000000, 0.000000000000000000 ) ) ;
#10312=CARTESIAN_POINT ( 'NONE',  ( 19.97576656849999921, -35.50000000000000000, -19.97576656849999921 ) ) ;
#10315=CARTESIAN_POINT ( 'NONE',  ( -0.5367793161509999411, -55.05574748869999979, -23.27036471170000098 ) ) ;
#10317=DIRECTION ( 'NONE',  ( 0.000000000000000000, 1.000000000000000000, 0.000000000000000000 ) ) ;
#10318=ORIENTED_EDGE ( 'NONE', *, *, #2888, .F. ) ;
#10320=CARTESIAN_POINT ( 'NONE',  ( -18.51518804340000202, -19.44981017040000282, 13.21263506969999924 ) ) ;
#10322=CARTESIAN_POINT ( 'NONE',  ( 8.125022609680000230, -36.17810633829999745, -21.26282345639999605 ) ) ;
#10324=CARTESIAN_POINT ( 'NONE',  ( 22.05228288849999885, -72.00360875399999827, -30.91980140109999553 ) ) ;
#10325=EDGE_CURVE ( 'NONE', #16095, #14660, #24841, .T. ) ;
#10327=CIRCLE ( 'NONE', #21109, 4.750000000000000888 ) ;
#10329=CARTESIAN_POINT ( 'NONE',  ( 21.45633488809999889, -36.07487150869999937, -7.289748192099999358 ) ) ;
#10331=CARTESIAN_POINT ( 'NONE',  ( 21.29631346280000059, -36.39568407349999291, -8.188957909990000061 ) ) ;
#10332=CARTESIAN_POINT ( 'NONE',  ( -9.708956880459998828, -80.00000000000000000, 43.08928339610000791 ) ) ;
#10333=VERTEX_POINT ( 'NONE', #7120 ) ;
#10339=ORIENTED_EDGE ( 'NONE', *, *, #9401, .T. ) ;
#10341=AXIS2_PLACEMENT_3D ( 'NONE', #21847, #11182, #4505 ) ;
#10342=CARTESIAN_POINT ( 'NONE',  ( 9.099149309629998683, -57.44066854489999940, -22.71963733680000175 ) ) ;
#10345=CYLINDRICAL_SURFACE ( 'NONE', #16734, 7.250000000000004441 ) ;
#10347=CARTESIAN_POINT ( 'NONE',  ( -13.00193227667292639, -19.48498969582177409, 19.66058068040372575 ) ) ;
#10348=CARTESIAN_POINT ( 'NONE',  ( 39.29494613547247894, -73.61009970497249810, 7.215638845165015525 ) ) ;
#10349=ORIENTED_EDGE ( 'NONE', *, *, #22654, .T. ) ;
#10350=CARTESIAN_POINT ( 'NONE',  ( 20.19515389160000396, -19.16582656490000147, -8.522375633559999386 ) ) ;
#10353=CARTESIAN_POINT ( 'NONE',  ( -14.12253468279999957, -74.03309514170000227, 36.41043208560000011 ) ) ;
#10354=DIRECTION ( 'NONE',  ( 0.9295286103719527793, 0.000000000000000000, 0.3687499999999814260 ) ) ;
#10357=CARTESIAN_POINT ( 'NONE',  ( 40.00000000000000000, -73.50000000000000000, 2.065014825799999939E-15 ) ) ;
#10359=CARTESIAN_POINT ( 'NONE',  ( 8.286111488879999598, -65.02206714839999790, -23.78780924429999999 ) ) ;
#10360=CARTESIAN_POINT ( 'NONE',  ( 7.370697001239634005, -73.94611239985914608, -38.67409491847346459 ) ) ;
#10361=CARTESIAN_POINT ( 'NONE',  ( 7.670973119660000172, -34.59820496239999699, -21.21808926809999818 ) ) ;
#10362=CARTESIAN_POINT ( 'NONE',  ( 5.326862811529999898E-15, -77.00000000000000000, -47.25000000000000000 ) ) ;
#10364=EDGE_CURVE ( 'NONE', #10257, #2641, #3051, .T. ) ;
#10367=AXIS2_PLACEMENT_3D ( 'NONE', #10662, #11252, #17833 ) ;
#10375=CARTESIAN_POINT ( 'NONE',  ( -7.135467526410000261, -73.50000000000000000, -38.71641004229999794 ) ) ;
#10379=CARTESIAN_POINT ( 'NONE',  ( 19.97576656849999921, -55.50000000000000000, -19.97576656849999921 ) ) ;
#10385=CIRCLE ( 'NONE', #26677, 2.000000000000000888 ) ;
#10387=DIRECTION ( 'NONE',  ( 0.000000000000000000, 1.000000000000000000, 0.000000000000000000 ) ) ;
#10388=FACE_OUTER_BOUND ( 'NONE', #17932, .T. ) ;
#10389=CARTESIAN_POINT ( 'NONE',  ( -23.11870653469999937, -72.31449597569999810, 16.58129546599999671 ) ) ;
#10393=CARTESIAN_POINT ( 'NONE',  ( 6.929578963970000061, -35.67530021650000549, -21.51138254459999999 ) ) ;
#10397=CARTESIAN_POINT ( 'NONE',  ( 22.60430443959999991, -36.06167118559999807, -10.71318590909999990 ) ) ;
#10398=ADVANCED_FACE ( 'NONE', ( #16427 ), #13832, .F. ) ;
#10399=EDGE_CURVE ( 'NONE', #212, #23252, #2851, .T. ) ;
#10401=CARTESIAN_POINT ( 'NONE',  ( -0.5436438173659999817, -58.35721741809999941, -23.39762436370000032 ) ) ;
#10402=CIRCLE ( 'NONE', #26729, 0.5000000000000004441 ) ;
#10403=CARTESIAN_POINT ( 'NONE',  ( 9.691266666139998875, -36.53611442790000297, -22.20987735279999953 ) ) ;
#10404=EDGE_CURVE ( 'NONE', #12727, #27727, #8398, .T. ) ;
#10409=CARTESIAN_POINT ( 'NONE',  ( 21.30237673919999608, -35.02344231349999859, -7.506539989010000191 ) ) ;
#10411=ORIENTED_EDGE ( 'NONE', *, *, #2988, .F. ) ;
#10412=AXIS2_PLACEMENT_3D ( 'NONE', #678, #2999, #23098 ) ;
#10413=DIRECTION ( 'NONE',  ( 0.2730005759809499555, 0.000000000000000000, -0.9620138697098237213 ) ) ;
#10414=CARTESIAN_POINT ( 'NONE',  ( -22.13750278361801449, -74.09775395658994057, -32.45700471235915785 ) ) ;
#10415=CARTESIAN_POINT ( 'NONE',  ( 21.77543175429999778, -18.50000000000000000, 8.809926792680000673 ) ) ;
#10416=CARTESIAN_POINT ( 'NONE',  ( -32.50515439522262540, -74.11794838461926815, -22.14922053471763164 ) ) ;
#10417=CARTESIAN_POINT ( 'NONE',  ( -20.33633474980000244, -58.84825201809999839, 14.70359657240000040 ) ) ;
#10418=ORIENTED_EDGE ( 'NONE', *, *, #20815, .T. ) ;
#10422=CARTESIAN_POINT ( 'NONE',  ( -0.5856137342820000313, -19.46510053389999939, -22.02591827759999887 ) ) ;
#10425=CARTESIAN_POINT ( 'NONE',  ( 10.08508256729999886, -64.24504434620000382, -24.78974309399999854 ) ) ;
#10426=DIRECTION ( 'NONE',  ( 1.000000000000000000, 0.000000000000000000, 0.000000000000000000 ) ) ;
#10427=VERTEX_POINT ( 'NONE', #17269 ) ;
#10429=AXIS2_PLACEMENT_3D ( 'NONE', #505, #13874, #5140 ) ;
#10431=EDGE_CURVE ( 'NONE', #15079, #7826, #19607, .T. ) ;
#10433=CARTESIAN_POINT ( 'NONE',  ( -12.79457676069784178, -70.02558174159734961, -24.23940011715129472 ) ) ;
#10434=FACE_OUTER_BOUND ( 'NONE', #13555, .T. ) ;
#10435=ORIENTED_EDGE ( 'NONE', *, *, #1951, .F. ) ;
#10436=VECTOR ( 'NONE', #674, 1000.000000000000000 ) ;
#10439=CARTESIAN_POINT ( 'NONE',  ( -7.283536107469999799, -74.14144860030000928, -39.92836808239999868 ) ) ;
#10440=ORIENTED_EDGE ( 'NONE', *, *, #24381, .F. ) ;
#10442=CARTESIAN_POINT ( 'NONE',  ( 19.53732555980000285, -35.60472305269999538, -8.991793591719998702 ) ) ;
#10450=ORIENTED_EDGE ( 'NONE', *, *, #3412, .F. ) ;
#10451=CIRCLE ( 'NONE', #27730, 4.750000000000000000 ) ;
#10452=CARTESIAN_POINT ( 'NONE',  ( 10.66842981584318295, -72.57936627267046958, -26.81288472990357263 ) ) ;
#10453=FACE_BOUND ( 'NONE', #11195, .T. ) ;
#10455=CARTESIAN_POINT ( 'NONE',  ( 21.83355004490000084, -37.95349900880000149, -8.543356255189999970 ) ) ;
#10458=CARTESIAN_POINT ( 'NONE',  ( 19.97576656849999921, -38.00000000000000000, -19.97576656849999921 ) ) ;
#10459=CARTESIAN_POINT ( 'NONE',  ( -14.42431928191101953, -74.07810314560701670, 36.25543878699895828 ) ) ;
#10460=DIRECTION ( 'NONE',  ( 0.000000000000000000, -1.000000000000000000, 0.000000000000000000 ) ) ;
#10465=CARTESIAN_POINT ( 'NONE',  ( -40.27753662873140428, -74.17170883818889138, -7.244686332484143065 ) ) ;
#10466=VERTEX_POINT ( 'NONE', #21610 ) ;
#10467=B_SPLINE_CURVE_WITH_KNOTS ( 'NONE', 3,
 ( #23316, #7303, #25079, #20715 ),
 .UNSPECIFIED., .F., .F.,
 ( 4, 4 ),
 ( 0.000000000000000000, 1.000000000000000000 ),
 .UNSPECIFIED. ) ;
#10468=CARTESIAN_POINT ( 'NONE',  ( 19.54920062769999944, -35.79804965070000122, -9.079275989799999280 ) ) ;
#10469=CARTESIAN_POINT ( 'NONE',  ( -8.467380000549999508, -74.00000000000000000, 37.95957158089999695 ) ) ;
#10474=VERTEX_POINT ( 'NONE', #28296 ) ;
#10476=DIRECTION ( 'NONE',  ( 0.000000000000000000, -1.000000000000000000, 0.000000000000000000 ) ) ;
#10479=VERTEX_POINT ( 'NONE', #16051 ) ;
#10482=CARTESIAN_POINT ( 'NONE',  ( 25.14017297600000234, -49.80573906499999737, 1.377424475129999992 ) ) ;
#10483=CARTESIAN_POINT ( 'NONE',  ( 23.93286062550000182, -64.98911155900000836, 10.71582475930000022 ) ) ;
#10485=ORIENTED_EDGE ( 'NONE', *, *, #12273, .T. ) ;
#10486=DIRECTION ( 'NONE',  ( 1.000000000000000000, 0.000000000000000000, 0.000000000000000000 ) ) ;
#10487=CARTESIAN_POINT ( 'NONE',  ( -14.20005211740000028, -74.02367878169998505, 36.23549608150000267 ) ) ;
#10490=ORIENTED_EDGE ( 'NONE', *, *, #962, .F. ) ;
#10491=CARTESIAN_POINT ( 'NONE',  ( -0.8996493333321277097, -74.26935822088371708, 47.19463505169927231 ) ) ;
#10494=CARTESIAN_POINT ( 'NONE',  ( -13.18221367349999973, -68.65989719860000662, -23.31533323539999714 ) ) ;
#10495=CARTESIAN_POINT ( 'NONE',  ( 20.84247163680000270, -57.47571004099999925, 10.69856784059999910 ) ) ;
#10496=DIRECTION ( 'NONE',  ( -0.3687499999999814260, 0.000000000000000000, 0.9295286103719527793 ) ) ;
#10497=ORIENTED_EDGE ( 'NONE', *, *, #19239, .F. ) ;
#10502=CARTESIAN_POINT ( 'NONE',  ( -32.70900267797851058, -74.50000000069999828, -21.69554430468080142 ) ) ;
#10503=CYLINDRICAL_SURFACE ( 'NONE', #12204, 3.749999999999996447 ) ;
#10504=FACE_OUTER_BOUND ( 'NONE', #7458, .T. ) ;
#10505=VERTEX_POINT ( 'NONE', #20431 ) ;
#10508=LINE ( 'NONE', #1952, #1879 ) ;
#10510=ORIENTED_EDGE ( 'NONE', *, *, #2045, .F. ) ;
#10511=CARTESIAN_POINT ( 'NONE',  ( -11.90026993885546602, -42.27314267039926676, -19.48333362464491003 ) ) ;
#10513=VERTEX_POINT ( 'NONE', #6595 ) ;
#10514=EDGE_LOOP ( 'NONE', ( #26525, #5552, #28646, #17454 ) ) ;
#10516=ADVANCED_FACE ( 'NONE', ( #15455 ), #208, .T. ) ;
#10522=CARTESIAN_POINT ( 'NONE',  ( -22.53552307149999834, -71.00576155849999793, 16.55302470919999536 ) ) ;
#10523=CARTESIAN_POINT ( 'NONE',  ( 0.000000000000000000, -82.25000000000000000, 0.000000000000000000 ) ) ;
#10524=CARTESIAN_POINT ( 'NONE',  ( -12.53135398279999890, -65.65894985500000303, -22.11805201909999852 ) ) ;
#10527=ORIENTED_EDGE ( 'NONE', *, *, #25638, .F. ) ;
#10528=CARTESIAN_POINT ( 'NONE',  ( 7.685455694319999864, -18.85523520590000146, -20.50116753240000023 ) ) ;
#10529=VERTEX_POINT ( 'NONE', #16497 ) ;
#10530=CARTESIAN_POINT ( 'NONE',  ( 22.30282385709999815, -36.18404282190000743, -10.32053919999999891 ) ) ;
#10531=CARTESIAN_POINT ( 'NONE',  ( 7.356933064080000584, -36.56811125840000187, -21.47791245320000186 ) ) ;
#10537=FACE_OUTER_BOUND ( 'NONE', #2008, .T. ) ;
#10542=CARTESIAN_POINT ( 'NONE',  ( -18.04504154990000231, -18.50000000000000000, 14.32575856849999951 ) ) ;
#10543=EDGE_CURVE ( 'NONE', #10981, #5413, #27958, .T. ) ;
#10547=CARTESIAN_POINT ( 'NONE',  ( -19.95528134719999969, -57.47855581339999986, 12.14623028109999936 ) ) ;
#10548=ORIENTED_EDGE ( 'NONE', *, *, #4331, .T. ) ;
#10552=LINE ( 'NONE', #12753, #8550 ) ;
#10555=EDGE_CURVE ( 'NONE', #19768, #27517, #9820, .T. ) ;
#10556=CARTESIAN_POINT ( 'NONE',  ( -10.89815191770000169, -18.50000000000000000, -17.99090140869999743 ) ) ;
#10558=CARTESIAN_POINT ( 'NONE',  ( -32.60214282289999943, -74.28456446479999897, -21.99410253310000130 ) ) ;
#10559=CARTESIAN_POINT ( 'NONE',  ( 36.66437779740000025, -79.55211029950000068, -14.61455063210000205 ) ) ;
#10562=CARTESIAN_POINT ( 'NONE',  ( -1.776356839399999804E-15, -79.50000000000000000, 47.25000000000000000 ) ) ;
#10564=VECTOR ( 'NONE', #3870, 1000.000000000000000 ) ;
#10565=CARTESIAN_POINT ( 'NONE',  ( -12.04650752959999949, -69.29982884310000202, -25.46956806489999892 ) ) ;
#10567=CIRCLE ( 'NONE', #14349, 7.249999999999999112 ) ;
#10568=ORIENTED_EDGE ( 'NONE', *, *, #4169, .F. ) ;
#10569=CARTESIAN_POINT ( 'NONE',  ( 20.49657866069999912, -57.47855601730000075, 11.20866246219999951 ) ) ;
#10570=DIRECTION ( 'NONE',  ( 0.000000000000000000, -1.000000000000000000, 0.000000000000000000 ) ) ;
#10573=CARTESIAN_POINT ( 'NONE',  ( 22.83075791639760510, -36.54217832149996781, -9.915197167589349547 ) ) ;
#10574=CARTESIAN_POINT ( 'NONE',  ( 22.13892079547798630, -37.96769806959605376, -8.928661031997458863 ) ) ;
#10576=DIRECTION ( 'NONE',  ( 0.000000000000000000, 1.000000000000000000, 0.000000000000000000 ) ) ;
#10578=ADVANCED_FACE ( 'NONE', ( #25256 ), #10692, .T. ) ;
#10581=DIRECTION ( 'NONE',  ( -0.8391385125251890065, -0.000000000000000000, -0.5439177849611219751 ) ) ;
#10583=CARTESIAN_POINT ( 'NONE',  ( 10.26571866753450735, -72.70657137122177005, -26.82921983142418654 ) ) ;
#10584=CARTESIAN_POINT ( 'NONE',  ( -12.09704001540000107, -74.00000000000000000, 47.10905722069999513 ) ) ;
#10585=VERTEX_POINT ( 'NONE', #17191 ) ;
#10589=AXIS2_PLACEMENT_3D ( 'NONE', #18707, #16935, #23217 ) ;
#10590=CARTESIAN_POINT ( 'NONE',  ( 8.600016245220459155, -57.45905972565284259, -22.33353789330169903 ) ) ;
#10591=CARTESIAN_POINT ( 'NONE',  ( 2.798556025240000070E-15, -74.00000000000000000, 3.175502518160000051E-15 ) ) ;
#10596=VERTEX_POINT ( 'NONE', #12795 ) ;
#10597=CARTESIAN_POINT ( 'NONE',  ( -39.75929607736751592, -73.82871504812071350, -7.246063797182709543 ) ) ;
#10600=CARTESIAN_POINT ( 'NONE',  ( 21.59259415360000034, -37.41349446709999427, -8.074292674670001446 ) ) ;
#10601=CARTESIAN_POINT ( 'NONE',  ( 7.215414233289999757, -74.50000000000000000, 40.70731707320000226 ) ) ;
#10602=ORIENTED_EDGE ( 'NONE', *, *, #17001, .T. ) ;
#10604=CIRCLE ( 'NONE', #18105, 0.5000000000000027756 ) ;
#10606=CARTESIAN_POINT ( 'NONE',  ( -40.70731707320000226, -82.25000000000000000, 7.215414233289999757 ) ) ;
#10612=EDGE_CURVE ( 'NONE', #24581, #14960, #22861, .T. ) ;
#10613=DIRECTION ( 'NONE',  ( 0.000000000000000000, 0.000000000000000000, 1.000000000000000000 ) ) ;
#10616=EDGE_CURVE ( 'NONE', #11515, #27229, #21898, .T. ) ;
#10618=CARTESIAN_POINT ( 'NONE',  ( 24.58067739159999832, -26.99662418180000145, 1.425465004250000112 ) ) ;
#10619=CARTESIAN_POINT ( 'NONE',  ( 23.63993607689999976, -65.72572872239999242, 10.85718295470000072 ) ) ;
#10621=ORIENTED_EDGE ( 'NONE', *, *, #21014, .F. ) ;
#10624=DIRECTION ( 'NONE',  ( 1.000000000000000000, 0.000000000000000000, 0.000000000000000000 ) ) ;
#10625=DIRECTION ( 'NONE',  ( 1.000000000000000000, 0.000000000000000000, 0.000000000000000000 ) ) ;
#10628=EDGE_CURVE ( 'NONE', #21742, #2030, #25636, .T. ) ;
#10629=CARTESIAN_POINT ( 'NONE',  ( 28.73411594649999756, -72.18745077389999665, 2.870220308499999984 ) ) ;
#10632=CARTESIAN_POINT ( 'NONE',  ( 8.575410935299998982, -64.96415972239999803, -23.78692408539999903 ) ) ;
#10633=CARTESIAN_POINT ( 'NONE',  ( -12.07243755420000042, -67.46050599719998786, -24.77969519869999715 ) ) ;
#10634=CARTESIAN_POINT ( 'NONE',  ( -16.78865735879999832, -72.00000000000000000, 25.46808810279999946 ) ) ;
#10635=DIRECTION ( 'NONE',  ( 1.000000000000000000, 0.000000000000000000, 0.000000000000000000 ) ) ;
#10636=EDGE_LOOP ( 'NONE', ( #28464, #26396, #18355, #19045 ) ) ;
#10637=CIRCLE ( 'NONE', #26976, 0.5000000000000027756 ) ;
#10643=CARTESIAN_POINT ( 'NONE',  ( 23.36120711399192018, -60.32159801849539349, 10.48029063133665950 ) ) ;
#10645=ORIENTED_EDGE ( 'NONE', *, *, #1571, .T. ) ;
#10650=FACE_OUTER_BOUND ( 'NONE', #23455, .T. ) ;
#10653=CARTESIAN_POINT ( 'NONE',  ( 8.586027522829999370, -36.03056633890000171, -20.93209955569999892 ) ) ;
#10656=AXIS2_PLACEMENT_3D ( 'NONE', #25373, #14142, #14421 ) ;
#10657=AXIS2_PLACEMENT_3D ( 'NONE', #12400, #23225, #27744 ) ;
#10658=EDGE_CURVE ( 'NONE', #24310, #4593, #25515, .T. ) ;
#10660=CARTESIAN_POINT ( 'NONE',  ( 22.05393571419999788, -18.50000000000000000, 1.471539986210000039 ) ) ;
#10662=CARTESIAN_POINT ( 'NONE',  ( -40.00000000000000000, -84.50000000000000000, -1.998401444329999950E-16 ) ) ;
#10666=CARTESIAN_POINT ( 'NONE',  ( 37.60355029590000697, -74.50000000000000000, 9.356041104380000917 ) ) ;
#10667=CARTESIAN_POINT ( 'NONE',  ( 9.444187806723459033, -35.99901531098080909, -19.97576011151723563 ) ) ;
#10669=CARTESIAN_POINT ( 'NONE',  ( -18.48779199151693220, -19.46686856770285345, 12.50825135346812012 ) ) ;
#10670=CARTESIAN_POINT ( 'NONE',  ( 7.253824032229999830, -36.56890884879999959, -21.48302425329999821 ) ) ;
#10672=ORIENTED_EDGE ( 'NONE', *, *, #22372, .F. ) ;
#10673=CARTESIAN_POINT ( 'NONE',  ( 36.40080305970000296, -74.58594344089999595, -14.77956079149999979 ) ) ;
#10674=CARTESIAN_POINT ( 'NONE',  ( 22.20987792570000252, -36.53611441549999483, -9.691267042979999857 ) ) ;
#10675=AXIS2_PLACEMENT_3D ( 'NONE', #7728, #25359, #11931 ) ;
#10677=EDGE_CURVE ( 'NONE', #2951, #19383, #10890, .T. ) ;
#10678=CARTESIAN_POINT ( 'NONE',  ( -1.453418026390000062, -61.82150526550000080, -24.08281248540000163 ) ) ;
#10680=CARTESIAN_POINT ( 'NONE',  ( -19.95527576509999790, -57.47855601730000075, 12.14622657969999864 ) ) ;
#10682=ORIENTED_EDGE ( 'NONE', *, *, #243, .T. ) ;
#10683=CARTESIAN_POINT ( 'NONE',  ( -19.95527577780000072, -57.47855601759999900, 12.14622656770000120 ) ) ;
#10684=CARTESIAN_POINT ( 'NONE',  ( 7.252014196660000245, -74.29300278830000082, -40.34091732179999923 ) ) ;
#10686=FACE_OUTER_BOUND ( 'NONE', #5080, .T. ) ;
#10689=CARTESIAN_POINT ( 'NONE',  ( 21.83467201959999926, -39.32886505740000160, 9.827746952760001875 ) ) ;
#10690=AXIS2_PLACEMENT_3D ( 'NONE', #5551, #14565, #21006 ) ;
#10691=CARTESIAN_POINT ( 'NONE',  ( -22.13657418456727299, -74.09627300783152748, -32.45321636354270822 ) ) ;
#10692=TOROIDAL_SURFACE ( 'NONE', #26099, 6.750000000000000000, 0.5000000000000000000 ) ;
#10693=CIRCLE ( 'NONE', #28398, 1.999999999999998890 ) ;
#10695=CARTESIAN_POINT ( 'NONE',  ( -32.23078363019764225, -74.03198227414637245, -22.08206013869884643 ) ) ;
#10699=CARTESIAN_POINT ( 'NONE',  ( -22.65530694619999963, -72.00000000000000000, 18.22957389299999775 ) ) ;
#10701=ORIENTED_EDGE ( 'NONE', *, *, #28663, .T. ) ;
#10704=ORIENTED_EDGE ( 'NONE', *, *, #18873, .F. ) ;
#10705=ADVANCED_FACE ( 'NONE', ( #9886 ), #12144, .F. ) ;
#10706=CARTESIAN_POINT ( 'NONE',  ( 19.99313163150000250, -36.00000036840000206, -9.451827061030000365 ) ) ;
#10707=AXIS2_PLACEMENT_3D ( 'NONE', #4871, #13752, #527 ) ;
#10711=CIRCLE ( 'NONE', #10274, 3.749999999999996447 ) ;
#10712=CARTESIAN_POINT ( 'NONE',  ( -19.86057790159999925, -54.24814459719999604, 12.08483967110000101 ) ) ;
#10714=ORIENTED_EDGE ( 'NONE', *, *, #23998, .T. ) ;
#10715=CARTESIAN_POINT ( 'NONE',  ( 23.09098980150000102, -54.98594849529999351, 10.35171084059999913 ) ) ;
#10716=CARTESIAN_POINT ( 'NONE',  ( 45.89652018349999452, -73.81415926540000783, -4.323400012419999605 ) ) ;
#10717=EDGE_CURVE ( 'NONE', #3822, #25360, #25160, .T. ) ;
#10718=ORIENTED_EDGE ( 'NONE', *, *, #19062, .T. ) ;
#10721=CARTESIAN_POINT ( 'NONE',  ( 9.807088892109998568, -36.00000000000000000, -20.27618918270000137 ) ) ;
#10725=DIRECTION ( 'NONE',  ( -0.8775825618903722036, 0.000000000000000000, 0.4794255386042041156 ) ) ;
#10727=DIRECTION ( 'NONE',  ( 0.000000000000000000, 1.000000000000000000, 0.000000000000000000 ) ) ;
#10728=CARTESIAN_POINT ( 'NONE',  ( -1.990166961069999907, -53.82492386869999734, -23.72420749220000147 ) ) ;
#10731=CARTESIAN_POINT ( 'NONE',  ( -19.41166767530000214, -18.86932112550000085, 14.42276170449999917 ) ) ;
#10734=SHAPE_REPRESENTATION ( 'Water Pump Main Cast Housing', ( #26433 ), #911 ) ;
#10738=CARTESIAN_POINT ( 'NONE',  ( 18.58445413780000166, -18.50000000000000000, 9.853938316409998066 ) ) ;
#10745=ORIENTED_EDGE ( 'NONE', *, *, #6844, .F. ) ;
#10746=AXIS2_PLACEMENT_3D ( 'NONE', #1570, #10413, #16997 ) ;
#10748=ORIENTED_EDGE ( 'NONE', *, *, #1884, .T. ) ;
#10749=CARTESIAN_POINT ( 'NONE',  ( 19.86198292329999759, -35.82855941500000085, -9.092038893569998947 ) ) ;
#10750=CYLINDRICAL_SURFACE ( 'NONE', #4174, 3.000000000000001332 ) ;
#10753=CIRCLE ( 'NONE', #12182, 3.000000000000002665 ) ;
#10755=EDGE_CURVE ( 'NONE', #23918, #25360, #6815, .T. ) ;
#10756=FACE_OUTER_BOUND ( 'NONE', #8742, .T. ) ;
#10757=DIRECTION ( 'NONE',  ( 1.000000000000000000, 0.000000000000000000, 0.000000000000000000 ) ) ;
#10760=CARTESIAN_POINT ( 'NONE',  ( 9.238026508649999968, -49.06719615769999621, -22.71123055929999879 ) ) ;
#10765=DIRECTION ( 'NONE',  ( -0.9704142011833030157, 0.000000000000000000, 0.2414462220490760924 ) ) ;
#10766=CARTESIAN_POINT ( 'NONE',  ( 25.86461527650000036, -68.93885193590000426, 10.86608366989999830 ) ) ;
#10768=EDGE_LOOP ( 'NONE', ( #15539, #1014, #23530, #4913, #16866, #7576, #24130 ) ) ;
#10769=FACE_OUTER_BOUND ( 'NONE', #7128, .T. ) ;
#10773=DIRECTION ( 'NONE',  ( 1.000000000000000000, 0.000000000000000000, -1.203338504109999799E-16 ) ) ;
#10774=AXIS2_PLACEMENT_3D ( 'NONE', #15805, #16397, #5187 ) ;
#10776=CARTESIAN_POINT ( 'NONE',  ( 25.67840951673019134, -74.29132473649202950, -29.62461545363389703 ) ) ;
#10778=CARTESIAN_POINT ( 'NONE',  ( 22.28403574200000037, -58.27079767440000069, 10.15038429719999868 ) ) ;
#10779=CARTESIAN_POINT ( 'NONE',  ( -11.21295062929999986, -49.81670839429999376, -22.19244673080000041 ) ) ;
#10780=AXIS2_PLACEMENT_3D ( 'NONE', #5327, #23106, #3146 ) ;
#10785=EDGE_CURVE ( 'NONE', #11872, #24375, #7957, .T. ) ;
#10790=ORIENTED_EDGE ( 'NONE', *, *, #14200, .F. ) ;
#10792=EDGE_CURVE ( 'NONE', #23252, #10529, #63, .T. ) ;
#10793=CARTESIAN_POINT ( 'NONE',  ( 20.59195074500000189, -22.47117435080000192, -8.142470642490000188 ) ) ;
#10798=CARTESIAN_POINT ( 'NONE',  ( 32.25000000000000000, -73.50000000000000000, 1.484822157706350179E-15 ) ) ;
#10802=DIRECTION ( 'NONE',  ( 0.000000000000000000, -1.000000000000000000, 0.000000000000000000 ) ) ;
#10804=DIRECTION ( 'NONE',  ( -0.7414446217286150276, 0.000000000000000000, -0.6710140631236509723 ) ) ;
#10805=EDGE_LOOP ( 'NONE', ( #22674, #27558, #11818, #11495 ) ) ;
#10808=CARTESIAN_POINT ( 'NONE',  ( -12.27251325432490781, -19.47282290365338397, 19.18777339616194055 ) ) ;
#10812=CARTESIAN_POINT ( 'NONE',  ( -13.84192735959999965, -18.50000000000000000, 18.94933192010000056 ) ) ;
#10813=CARTESIAN_POINT ( 'NONE',  ( 19.69582338720000081, -18.50000000000000000, -7.383548592259999488 ) ) ;
#10815=AXIS2_PLACEMENT_3D ( 'NONE', #11555, #20464, #11859 ) ;
#10817=LINE ( 'NONE', #24535, #20356 ) ;
#10819=CARTESIAN_POINT ( 'NONE',  ( 18.98656275410000305, -20.74345739960000401, -9.020322599649999162 ) ) ;
#10820=VERTEX_POINT ( 'NONE', #2014 ) ;
#10822=EDGE_CURVE ( 'NONE', #17492, #13409, #24230, .T. ) ;
#10824=CARTESIAN_POINT ( 'NONE',  ( -2.646733530900000186, -62.35648592489999942, -25.81438035669999564 ) ) ;
#10825=CARTESIAN_POINT ( 'NONE',  ( 9.022692971490000602, -37.05206027789999723, -21.94388125080000052 ) ) ;
#10827=CARTESIAN_POINT ( 'NONE',  ( -19.72357768420000212, -55.05548131559999803, 12.36420953449999871 ) ) ;
#10830=AXIS2_PLACEMENT_3D ( 'NONE', #1779, #16291, #14399 ) ;
#10831=CARTESIAN_POINT ( 'NONE',  ( 21.39448334389999928, -35.36119160450000010, -7.275524378479999221 ) ) ;
#10832=CARTESIAN_POINT ( 'NONE',  ( 7.367357169079999935, -74.05258142279998879, -39.49501612619999946 ) ) ;
#10833=VERTEX_POINT ( 'NONE', #13205 ) ;
#10837=CARTESIAN_POINT ( 'NONE',  ( -10.09856422800000075, -18.50000000000000000, -18.66762288940000403 ) ) ;
#10844=DIRECTION ( 'NONE',  ( 1.000000000000000000, 0.000000000000000000, 0.000000000000000000 ) ) ;
#10846=CARTESIAN_POINT ( 'NONE',  ( 22.85380330025371265, -61.78215645786973909, -7.276638066883097444 ) ) ;
#10848=CIRCLE ( 'NONE', #2525, 0.5000000000000004441 ) ;
#10849=CARTESIAN_POINT ( 'NONE',  ( 8.472395020760000506, -37.95144078679999922, -21.79230213740000011 ) ) ;
#10850=CARTESIAN_POINT ( 'NONE',  ( 36.75955791450000021, -80.34763096870000254, -13.75991944210000106 ) ) ;
#10852=EDGE_CURVE ( 'NONE', #16224, #22982, #17726, .T. ) ;
#10854=CARTESIAN_POINT ( 'NONE',  ( 25.26718046270000073, -72.00000000000000000, 6.129403842640000377 ) ) ;
#10855=CARTESIAN_POINT ( 'NONE',  ( -22.71848792900000191, -80.00000000000000000, -32.61798286559999838 ) ) ;
#10856=CARTESIAN_POINT ( 'NONE',  ( -0.5421338679160000451, -57.91805294160000273, -23.37022173519999768 ) ) ;
#10859=ORIENTED_EDGE ( 'NONE', *, *, #4859, .T. ) ;
#10861=CARTESIAN_POINT ( 'NONE',  ( 0.000000000000000000, -19.46510050329999686, 0.000000000000000000 ) ) ;
#10864=CARTESIAN_POINT ( 'NONE',  ( -22.62871153299999705, -80.00000000000000000, -32.48908674569999988 ) ) ;
#10870=ORIENTED_EDGE ( 'NONE', *, *, #2988, .T. ) ;
#10871=DIRECTION ( 'NONE',  ( 1.000000000000000000, 0.000000000000000000, 0.000000000000000000 ) ) ;
#10875=CARTESIAN_POINT ( 'NONE',  ( -0.5413028955969999556, -57.47855601730000075, -23.35488904190000170 ) ) ;
#10877=AXIS2_PLACEMENT_3D ( 'NONE', #19865, #4435, #11261 ) ;
#10878=CARTESIAN_POINT ( 'NONE',  ( 10.38182607682433378, -72.67376041724993740, -26.81396579421036463 ) ) ;
#10879=CARTESIAN_POINT ( 'NONE',  ( -19.47508940490000029, -19.49504784870000051, 14.31286723660000071 ) ) ;
#10880=ORIENTED_EDGE ( 'NONE', *, *, #28443, .T. ) ;
#10882=AXIS2_PLACEMENT_3D ( 'NONE', #131, #13496, #24880 ) ;
#10890=LINE ( 'NONE', #22148, #20518 ) ;
#10892=EDGE_LOOP ( 'NONE', ( #262, #5160, #9798, #24558, #4223 ) ) ;
#10893=B_SPLINE_CURVE_WITH_KNOTS ( 'NONE', 5,
 ( #19376, #24323, #4063, #10322, #28124, #17481, #17048, #22714, #27232 ),
 .UNSPECIFIED., .F., .F.,
 ( 6, 3, 6 ),
 ( 0.000000000000000000, 0.5000000000000000000, 1.000000000000000000 ),
 .UNSPECIFIED. ) ;
#10895=ORIENTED_EDGE ( 'NONE', *, *, #25330, .F. ) ;
#10896=CARTESIAN_POINT ( 'NONE',  ( -11.62935565859999798, -49.87337825049999651, 20.03543646159999980 ) ) ;
#10897=CARTESIAN_POINT ( 'NONE',  ( 7.383549334360000493, -18.50000000000000000, -19.69582310909999734 ) ) ;
#10900=CARTESIAN_POINT ( 'NONE',  ( -3.240188565246664432, -67.45413847081940162, -27.37092558598135028 ) ) ;
#10903=CARTESIAN_POINT ( 'NONE',  ( 9.332951828819998852, -36.18018306619999436, -21.06416784469999826 ) ) ;
#10907=ORIENTED_EDGE ( 'NONE', *, *, #7254, .F. ) ;
#10910=CARTESIAN_POINT ( 'NONE',  ( 23.35417710990000373, -57.47855602609999437, -0.5711871778539999722 ) ) ;
#10912=CARTESIAN_POINT ( 'NONE',  ( 39.30828467216858968, -73.61493928630405037, 7.216929735073121854 ) ) ;
#10914=B_SPLINE_CURVE_WITH_KNOTS ( 'NONE', 3,
 ( #10196, #14454, #7768, #5840, #21435, #25401 ),
 .UNSPECIFIED., .F., .F.,
 ( 4, 2, 4 ),
 ( 0.000000000000000000, 0.5000000000000000000, 1.000000000000000000 ),
 .UNSPECIFIED. ) ;
#10915=CARTESIAN_POINT ( 'NONE',  ( -38.70548889989999708, -73.81415926540000783, 7.196178079599999222 ) ) ;
#10917=DIRECTION ( 'NONE',  ( 1.000000000000000000, 0.000000000000000000, 0.000000000000000000 ) ) ;
#10919=ADVANCED_FACE ( 'NONE', ( #11896 ), #10107, .F. ) ;
#10920=CARTESIAN_POINT ( 'NONE',  ( 28.19138828400000207, -71.67693266270001118, 1.948646730969999963 ) ) ;
#10922=CARTESIAN_POINT ( 'NONE',  ( 22.44846404289852515, -74.05540946579084505, -31.87117065944173433 ) ) ;
#10924=EDGE_CURVE ( 'NONE', #5668, #10427, #1086, .T. ) ;
#10925=CARTESIAN_POINT ( 'NONE',  ( -10.92535406200000025, -42.25468912499999874, -20.74622789749999896 ) ) ;
#10926=ORIENTED_EDGE ( 'NONE', *, *, #6640, .T. ) ;
#10927=EDGE_CURVE ( 'NONE', #2868, #14159, #14709, .T. ) ;
#10928=CARTESIAN_POINT ( 'NONE',  ( 22.16163108380142432, -57.47158985094319661, -7.992697376200416315 ) ) ;
#10930=ORIENTED_EDGE ( 'NONE', *, *, #13277, .T. ) ;
#10933=CARTESIAN_POINT ( 'NONE',  ( 7.435983481019023955, -74.13941005068963364, 39.48497135292184623 ) ) ;
#10936=CARTESIAN_POINT ( 'NONE',  ( 36.25000000000000000, -69.00000000000000000, 2.314797894279999601E-15 ) ) ;
#10938=CARTESIAN_POINT ( 'NONE',  ( 27.04769748009325880, -72.23842146203566017, -11.44023399195399371 ) ) ;
#10939=DIRECTION ( 'NONE',  ( 1.000000000000000000, 0.000000000000000000, 0.000000000000000000 ) ) ;
#10944=CARTESIAN_POINT ( 'NONE',  ( 23.15198552840000090, -19.16887642500000055, 1.371920395479999888 ) ) ;
#10948=CARTESIAN_POINT ( 'NONE',  ( 28.44483739272424216, -70.46285482980914594, 2.597167156265934640 ) ) ;
#10950=EDGE_CURVE ( 'NONE', #5438, #1018, #13055, .T. ) ;
#10951=CARTESIAN_POINT ( 'NONE',  ( 6.931585813929999951, -44.93330283539999925, -21.84994998139999822 ) ) ;
#10953=CARTESIAN_POINT ( 'NONE',  ( -12.73274366210000075, -67.57003242140000054, -23.00245288660000043 ) ) ;
#10956=CARTESIAN_POINT ( 'NONE',  ( -10.27945668490000131, -18.50000000000000000, 18.70272521329999904 ) ) ;
#10957=ORIENTED_EDGE ( 'NONE', *, *, #15825, .F. ) ;
#10958=EDGE_CURVE ( 'NONE', #17392, #15244, #12659, .T. ) ;
#10959=CARTESIAN_POINT ( 'NONE',  ( 8.857880004760000148, -18.86754460619999918, -19.35192615410000272 ) ) ;
#10960=CARTESIAN_POINT ( 'NONE',  ( 22.49242817279999684, -37.98196143189999674, -9.212282262639998720 ) ) ;
#10961=EDGE_LOOP ( 'NONE', ( #8758, #18202, #12679, #338 ) ) ;
#10962=CARTESIAN_POINT ( 'NONE',  ( -12.71547034009999955, -65.00127802399998700, 21.72228991030000245 ) ) ;
#10964=CARTESIAN_POINT ( 'NONE',  ( 9.219197186969998015, -37.05706108660000098, -22.15413563950000153 ) ) ;
#10966=CARTESIAN_POINT ( 'NONE',  ( -19.63524818169999975, -57.47122622290000749, 13.01113544189999871 ) ) ;
#10967=CARTESIAN_POINT ( 'NONE',  ( -20.19582590579999959, -52.57401960350014036, 14.62459034920000001 ) ) ;
#10968=ORIENTED_EDGE ( 'NONE', *, *, #6337, .F. ) ;
#10971=EDGE_LOOP ( 'NONE', ( #23666, #17065, #21811, #1921 ) ) ;
#10972=CYLINDRICAL_SURFACE ( 'NONE', #6614, 0.9999999999999988898 ) ;
#10973=EDGE_LOOP ( 'NONE', ( #26541, #27363, #13744, #16126 ) ) ;
#10974=CARTESIAN_POINT ( 'NONE',  ( -9.927741060089999792, -18.50000000000000000, -22.19465444469999937 ) ) ;
#10977=CARTESIAN_POINT ( 'NONE',  ( 20.49657866619999780, -57.47855601759999900, 11.20866246179999948 ) ) ;
#10978=CARTESIAN_POINT ( 'NONE',  ( 8.782859991099998709, -69.73939502419999314, -25.82418225190000172 ) ) ;
#10980=B_SPLINE_SURFACE_WITH_KNOTS ( 'NONE', 5, 5, ( 
 ( #5853, #21179, #16515, #21450, #18854, #18985 ),
 ( #25690, #14599, #23503, #1361, #8049, #16940 ),
 ( #22024, #19678, #1927, #1646, #24351, #12959 ),
 ( #10766, #11051, #6578, #21588, #28423, #6129 ),
 ( #3953, #15002, #15143, #28277, #15283, #23916 ),
 ( #24051, #12816, #15439, #26390, #17359, #21726 ),
 ( #1776, #19966, #10619, #4091, #19535, #8456 ),
 ( #28567, #10483, #19395, #12677, #26254, #17211 ),
 ( #4241, #26103, #6277, #21873, #8602, #17505 ) ),
 .UNSPECIFIED., .F., .F., .F.,
 ( 6, 3, 6 ),
 ( 6, 6 ),
 ( 41.71218049779999859, 49.83411874859999813, 53.81665561530000019 ),
 ( 0.000000000000000000, 2.000000000000000000 ),
 .UNSPECIFIED. ) ;
#10981=VERTEX_POINT ( 'NONE', #14987 ) ;
#10983=CARTESIAN_POINT ( 'NONE',  ( 26.79207366509999844, -72.75494331939999881, -10.16049586859999998 ) ) ;
#10990=EDGE_LOOP ( 'NONE', ( #18172, #13350, #3566, #9966 ) ) ;
#10994=CARTESIAN_POINT ( 'NONE',  ( -22.62871152338947311, -80.00000000056968474, -32.48908675062602924 ) ) ;
#10997=CYLINDRICAL_SURFACE ( 'NONE', #5802, 3.000000000000001332 ) ;
#11000=CARTESIAN_POINT ( 'NONE',  ( 46.22668039279999874, -73.89966597549998539, -4.016967337520000569 ) ) ;
#11001=ORIENTED_EDGE ( 'NONE', *, *, #25951, .T. ) ;
#11012=DIRECTION ( 'NONE',  ( 0.3687499999999813705, 0.000000000000000000, -0.9295286103719528903 ) ) ;
#11014=CARTESIAN_POINT ( 'NONE',  ( -2.489779910060000212, -56.21886023140000077, -24.59145677380000095 ) ) ;
#11015=DIRECTION ( 'NONE',  ( 1.000000000000000000, 0.000000000000000000, 0.000000000000000000 ) ) ;
#11018=CARTESIAN_POINT ( 'NONE',  ( -19.02205191440000220, -19.48534420260000033, 13.96959728589999905 ) ) ;
#11020=CARTESIAN_POINT ( 'NONE',  ( -15.95377854864229050, -18.50000000000000000, 21.99697738415282799 ) ) ;
#11022=DIRECTION ( 'NONE',  ( -0.5715342875219319163, 0.000000000000000000, -0.8205781852979018298 ) ) ;
#11025=AXIS2_PLACEMENT_3D ( 'NONE', #617, #16161, #5101 ) ;
#11032=ORIENTED_EDGE ( 'NONE', *, *, #14361, .F. ) ;
#11035=DIRECTION ( 'NONE',  ( 0.4794255386042040601, 0.000000000000000000, 0.8775825618903720926 ) ) ;
#11036=ORIENTED_EDGE ( 'NONE', *, *, #24810, .T. ) ;
#11040=ORIENTED_EDGE ( 'NONE', *, *, #565, .T. ) ;
#11045=CARTESIAN_POINT ( 'NONE',  ( 22.17953377930000158, -65.07443093669999712, 11.85657293289999892 ) ) ;
#11048=CARTESIAN_POINT ( 'NONE',  ( 6.717799458580000049, -84.50000000000000000, 40.65853658540000026 ) ) ;
#11049=EDGE_CURVE ( 'NONE', #7605, #9894, #18213, .T. ) ;
#11050=CARTESIAN_POINT ( 'NONE',  ( 24.20832872070000263, -49.83808240369999254, 1.215820334740000064 ) ) ;
#11051=CARTESIAN_POINT ( 'NONE',  ( 25.49852039510000168, -69.13896873969999035, 10.91553851559999977 ) ) ;
#11054=CARTESIAN_POINT ( 'NONE',  ( -12.84659744679999882, -72.82938648530000592, -25.64625568420000334 ) ) ;
#11061=DIRECTION ( 'NONE',  ( 1.291895883199999965E-15, -0.000000000000000000, 1.000000000000000000 ) ) ;
#11063=CARTESIAN_POINT ( 'NONE',  ( -11.67870342830000041, -57.47571039179999985, -20.30949892389999789 ) ) ;
#11064=CARTESIAN_POINT ( 'NONE',  ( 22.26662627820000040, -57.47855601759999900, -7.066909182079999852 ) ) ;
#11065=CIRCLE ( 'NONE', #11558, 25.14975229270000057 ) ;
#11066=EDGE_LOOP ( 'NONE', ( #12483, #3043, #23489, #7004 ) ) ;
#11069=CIRCLE ( 'NONE', #11578, 7.249999999999999112 ) ;
#11071=ORIENTED_EDGE ( 'NONE', *, *, #21964, .F. ) ;
#11072=CARTESIAN_POINT ( 'NONE',  ( 7.196178079599999222, -73.81415926540000783, 38.70548889989999708 ) ) ;
#11074=ADVANCED_FACE ( 'NONE', ( #24478 ), #24627, .F. ) ;
#11075=CARTESIAN_POINT ( 'NONE',  ( -10.20110288159999890, -80.00000000000000000, 41.00000000000000000 ) ) ;
#11076=CARTESIAN_POINT ( 'NONE',  ( 22.29295329801293235, -19.46656432701744777, 0.4976463741603174284 ) ) ;
#11078=ORIENTED_EDGE ( 'NONE', *, *, #22231, .T. ) ;
#11079=CARTESIAN_POINT ( 'NONE',  ( 0.000000000000000000, -84.00000000000000000, 0.000000000000000000 ) ) ;
#11082=CARTESIAN_POINT ( 'NONE',  ( 9.203357703080000007, -35.92863931600000171, -19.97610107710000094 ) ) ;
#11083=EDGE_CURVE ( 'NONE', #16955, #19768, #18702, .T. ) ;
#11084=CARTESIAN_POINT ( 'NONE',  ( 21.43169449828233653, -35.31509369946678589, -7.132046020603563186 ) ) ;
#11086=CARTESIAN_POINT ( 'NONE',  ( -12.16664950528991440, -19.47159289567763096, 19.15110637680422201 ) ) ;
#11090=VERTEX_POINT ( 'NONE', #2642 ) ;
#11092=CARTESIAN_POINT ( 'NONE',  ( -14.40572000550000098, -18.50000000000000000, 20.06574520719999910 ) ) ;
#11095=CONICAL_SURFACE ( 'NONE', #9737, 25.14975229270001833, 0.4276056667390000787 ) ;
#11096=AXIS2_PLACEMENT_3D ( 'NONE', #24149, #8827, #11310 ) ;
#11097=FACE_OUTER_BOUND ( 'NONE', #4343, .T. ) ;
#11100=CARTESIAN_POINT ( 'NONE',  ( 26.13951773519340094, -63.17363326945925195, 1.458190918673929248 ) ) ;
#11104=ORIENTED_EDGE ( 'NONE', *, *, #28406, .T. ) ;
#11105=CARTESIAN_POINT ( 'NONE',  ( 8.076031017920000110, -18.85700242990000319, -20.35668352559999761 ) ) ;
#11106=ORIENTED_EDGE ( 'NONE', *, *, #18170, .F. ) ;
#11107=CARTESIAN_POINT ( 'NONE',  ( -11.79670204130000144, -63.63842289929999652, 21.46815698109999815 ) ) ;
#11110=EDGE_CURVE ( 'NONE', #25354, #26232, #4287, .T. ) ;
#11111=CARTESIAN_POINT ( 'NONE',  ( -19.79577514300000018, -57.47815920199999340, 12.40824665329999910 ) ) ;
#11112=DIRECTION ( 'NONE',  ( 0.000000000000000000, 1.000000000000000000, 0.000000000000000000 ) ) ;
#11116=CARTESIAN_POINT ( 'NONE',  ( -11.90992159604306622, -57.47815920418752711, -20.09952900877129878 ) ) ;
#11117=ORIENTED_EDGE ( 'NONE', *, *, #23244, .F. ) ;
#11119=CARTESIAN_POINT ( 'NONE',  ( 0.000000000000000000, -65.07443093669999712, 0.000000000000000000 ) ) ;
#11121=ORIENTED_EDGE ( 'NONE', *, *, #806, .F. ) ;
#11122=EDGE_CURVE ( 'NONE', #20659, #22866, #14138, .T. ) ;
#11124=B_SPLINE_CURVE_WITH_KNOTS ( 'NONE', 5,
 ( #27638, #25578, #8080, #7679, #16545, #5610 ),
 .UNSPECIFIED., .F., .F.,
 ( 6, 6 ),
 ( 0.000000000000000000, 1.000000000000000000 ),
 .UNSPECIFIED. ) ;
#11125=EDGE_CURVE ( 'NONE', #19131, #24445, #14028, .T. ) ;
#11128=CARTESIAN_POINT ( 'NONE',  ( 20.12528277150000022, -32.73099401700000044, 10.22949540999999840 ) ) ;
#11131=CARTESIAN_POINT ( 'NONE',  ( 18.75935060549999989, -18.50000000000000000, 10.17575150659999927 ) ) ;
#11132=CARTESIAN_POINT ( 'NONE',  ( -32.64751318483137510, -80.00000000000000000, -22.65605297795088191 ) ) ;
#11136=CARTESIAN_POINT ( 'NONE',  ( 9.008529550149999565, -24.55588640339999884, -19.11129932280000077 ) ) ;
#11138=CARTESIAN_POINT ( 'NONE',  ( 21.61954412840861295, -19.48585536712340271, 9.522048220035644661 ) ) ;
#11141=ORIENTED_EDGE ( 'NONE', *, *, #12445, .T. ) ;
#11142=AXIS2_PLACEMENT_3D ( 'NONE', #10294, #7858, #8257 ) ;
#11145=ORIENTED_EDGE ( 'NONE', *, *, #20622, .T. ) ;
#11146=B_SPLINE_CURVE_WITH_KNOTS ( 'NONE', 5,
 ( #6225, #4182, #2159, #15228, #10994, #19907 ),
 .UNSPECIFIED., .F., .F.,
 ( 6, 6 ),
 ( 0.000000000000000000, 1.000000000000000000 ),
 .UNSPECIFIED. ) ;
#11147=FACE_OUTER_BOUND ( 'NONE', #23037, .T. ) ;
#11151=ORIENTED_EDGE ( 'NONE', *, *, #10151, .T. ) ;
#11157=CARTESIAN_POINT ( 'NONE',  ( 46.57616008939999830, -73.79912698820000116, -3.102537739159999752 ) ) ;
#11158=ORIENTED_EDGE ( 'NONE', *, *, #27939, .T. ) ;
#11165=ORIENTED_EDGE ( 'NONE', *, *, #6343, .F. ) ;
#11166=CARTESIAN_POINT ( 'NONE',  ( 8.556786983500000332, -37.95394734039999918, -21.84310845219999919 ) ) ;
#11168=DIRECTION ( 'NONE',  ( 1.000000000000000000, 0.000000000000000000, 0.000000000000000000 ) ) ;
#11172=DIRECTION ( 'NONE',  ( 0.2414462220490750377, 0.000000000000000000, 0.9704142011833034598 ) ) ;
#11176=CARTESIAN_POINT ( 'NONE',  ( -13.46276276179999876, -19.49999999970000175, 20.39865906480000035 ) ) ;
#11177=CARTESIAN_POINT ( 'NONE',  ( 7.600490370247736216, -74.00013394018854740, -38.79561088320171791 ) ) ;
#11180=CARTESIAN_POINT ( 'NONE',  ( 7.675802467110550253, -57.47600031385420039, -22.13628273390180468 ) ) ;
#11182=DIRECTION ( 'NONE',  ( 0.000000000000000000, 1.000000000000000000, 0.000000000000000000 ) ) ;
#11183=CIRCLE ( 'NONE', #21009, 3.749999999999996447 ) ;
#11189=CARTESIAN_POINT ( 'NONE',  ( 24.71478484869999903, -57.43018266680000039, 1.313252026010000018 ) ) ;
#11192=ORIENTED_EDGE ( 'NONE', *, *, #22711, .F. ) ;
#11195=EDGE_LOOP ( 'NONE', ( #14789, #12062 ) ) ;
#11196=CARTESIAN_POINT ( 'NONE',  ( 34.89999999999999858, -86.00000000000000000, 4.273876174839999917E-15 ) ) ;
#11197=LINE ( 'NONE', #22898, #6511 ) ;
#11199=CARTESIAN_POINT ( 'NONE',  ( -40.00000000000000000, -69.50000000000000000, -8.881784197000000993E-16 ) ) ;
#11200=EDGE_CURVE ( 'NONE', #12661, #9424, #20068, .T. ) ;
#11207=CARTESIAN_POINT ( 'NONE',  ( 12.05743353869999979, -65.07443093669999712, 22.07098404789999790 ) ) ;
#11208=ORIENTED_EDGE ( 'NONE', *, *, #4036, .T. ) ;
#11210=DIRECTION ( 'NONE',  ( -0.5301416321220548955, 0.000000000000000000, -0.8479091047340887588 ) ) ;
#11212=CARTESIAN_POINT ( 'NONE',  ( -20.50880539726380292, -61.98877831146614170, 12.53749828487332252 ) ) ;
#11213=CARTESIAN_POINT ( 'NONE',  ( 40.52471374997017506, -74.35734738321731641, 7.233314584394662461 ) ) ;
#11214=ORIENTED_EDGE ( 'NONE', *, *, #7754, .F. ) ;
#11219=CARTESIAN_POINT ( 'NONE',  ( 27.45110624719999848, -70.13570072960000346, 0.6191059290799999504 ) ) ;
#11220=B_SPLINE_CURVE_WITH_KNOTS ( 'NONE', 5,
 ( #28339, #10967, #15199, #13174, #21649, #22085, #12735, #1698, #19451 ),
 .UNSPECIFIED., .F., .F.,
 ( 6, 3, 6 ),
 ( 0.000000000000000000, 0.5000000000000000000, 1.000000000000000000 ),
 .UNSPECIFIED. ) ;
#11222=EDGE_CURVE ( 'NONE', #15463, #5258, #19553, .T. ) ;
#11226=CARTESIAN_POINT ( 'NONE',  ( -11.34636246480000032, -49.86909869750000013, -20.35003598449999984 ) ) ;
#11227=CARTESIAN_POINT ( 'NONE',  ( 22.33353861310135358, -57.45905989834243144, -8.600015579560372103 ) ) ;
#11230=CIRCLE ( 'NONE', #19623, 0.5000000000000027756 ) ;
#11231=ORIENTED_EDGE ( 'NONE', *, *, #17942, .T. ) ;
#11232=EDGE_CURVE ( 'NONE', #4093, #22777, #23045, .T. ) ;
#11237=ORIENTED_EDGE ( 'NONE', *, *, #8370, .T. ) ;
#11240=B_SPLINE_SURFACE_WITH_KNOTS ( 'NONE', 5, 5, ( 
 ( #28163, #8196, #17083, #26117, #25976, #6000, #12282, #23931, #14881 ),
 ( #1660, #23790, #16662, #5595, #7926, #3828, #1243, #25557, #12691 ),
 ( #14476, #10082, #27879, #22479, #24659, #28709, #6433, #26849, #4692 ),
 ( #8615, #6290, #26701, #22038, #10925, #19549, #2086, #19831, #21888 ),
 ( #13570, #10779, #8896, #15606, #15296, #11226, #13272, #20132, #22181 ),
 ( #15156, #8748, #17665, #2521, #17810, #202, #11063, #26549, #28437 ) ),
 .UNSPECIFIED., .F., .F., .F.,
 ( 6, 6 ),
 ( 6, 3, 6 ),
 ( 15.94303934740000095, 69.72897805050000386 ),
 ( 0.000000000000000000, 1.000000000000000000, 2.000000000000000000 ),
 .UNSPECIFIED. ) ;
#11241=CARTESIAN_POINT ( 'NONE',  ( 23.51796030652247893, -19.48482983503955168, 1.427212532244023668 ) ) ;
#11244=CARTESIAN_POINT ( 'NONE',  ( 27.09220507755102858, -72.19826629891751679, -11.51208668783220013 ) ) ;
#11246=CARTESIAN_POINT ( 'NONE',  ( 8.435862578959998359, -36.92586548770000121, -21.49743428369999521 ) ) ;
#11249=CARTESIAN_POINT ( 'NONE',  ( 19.69582338720000081, -18.50000000000000000, -7.383548592259999488 ) ) ;
#11250=LINE ( 'NONE', #5001, #559 ) ;
#11252=DIRECTION ( 'NONE',  ( 0.000000000000000000, 1.000000000000000000, 0.000000000000000000 ) ) ;
#11254=CIRCLE ( 'NONE', #22927, 13.00000000000000178 ) ;
#11255=CARTESIAN_POINT ( 'NONE',  ( -14.10948125060000002, -18.50000000000000000, 20.17033318009999832 ) ) ;
#11258=ADVANCED_FACE ( 'NONE', ( #24744 ), #15833, .T. ) ;
#11259=CARTESIAN_POINT ( 'NONE',  ( 36.61022179955299549, -75.00000020938335865, -14.75000000000000178 ) ) ;
#11261=DIRECTION ( 'NONE',  ( 1.000000000000000000, 0.000000000000000000, 0.000000000000000000 ) ) ;
#11262=CARTESIAN_POINT ( 'NONE',  ( -10.42741367090000004, -18.61794786490000320, 18.97192220850000055 ) ) ;
#11264=CARTESIAN_POINT ( 'NONE',  ( -32.20769383860636026, -80.36910031991209280, -22.43272069095936416 ) ) ;
#11267=CARTESIAN_POINT ( 'NONE',  ( -13.76017623309999927, -64.69849637139999743, 21.59184277249999795 ) ) ;
#11268=CARTESIAN_POINT ( 'NONE',  ( -12.30235599149999892, -63.58904326009999153, 21.23101024950000237 ) ) ;
#11269=CARTESIAN_POINT ( 'NONE',  ( 7.243843118859103924, -74.18716007600167472, 40.29875214202166944 ) ) ;
#11271=VECTOR ( 'NONE', #14284, 1000.000000000000000 ) ;
#11272=B_SPLINE_CURVE_WITH_KNOTS ( 'NONE', 3,
 ( #5322, #16813, #7664, #27624 ),
 .UNSPECIFIED., .F., .F.,
 ( 4, 4 ),
 ( 0.000000000000000000, 1.000000000000000000 ),
 .UNSPECIFIED. ) ;
#11276=CARTESIAN_POINT ( 'NONE',  ( 19.96273463004390081, -19.47964434323706939, -8.629719000944380269 ) ) ;
#11277=CARTESIAN_POINT ( 'NONE',  ( -11.46863496920000003, -57.40875702469999453, -22.62382260909999943 ) ) ;
#11279=CARTESIAN_POINT ( 'NONE',  ( -7.250133233359999707, -73.75841684550000821, -39.12193274490000050 ) ) ;
#11282=ORIENTED_EDGE ( 'NONE', *, *, #18136, .F. ) ;
#11285=CARTESIAN_POINT ( 'NONE',  ( 7.215414233289999757, -84.00000000000000000, -40.70731707320000226 ) ) ;
#11287=CARTESIAN_POINT ( 'NONE',  ( 20.29473261270000251, -45.99930305829999355, 10.74246239310000028 ) ) ;
#11290=CARTESIAN_POINT ( 'NONE',  ( -13.93619502189999970, -74.00000000010000178, 36.24163866030000491 ) ) ;
#11291=CARTESIAN_POINT ( 'NONE',  ( 10.39238870299999995, -67.58693996879999588, -25.45267030080000126 ) ) ;
#11295=DIRECTION ( 'NONE',  ( 0.000000000000000000, 1.000000000000000000, 0.000000000000000000 ) ) ;
#11296=CARTESIAN_POINT ( 'NONE',  ( 38.08875739639999836, -84.00000000000000000, 9.476764215410000247 ) ) ;
#11299=CIRCLE ( 'NONE', #28061, 4.750000000000000888 ) ;
#11301=CARTESIAN_POINT ( 'NONE',  ( 22.76002593507040928, -61.37679267133752603, -7.241526953473480965 ) ) ;
#11302=EDGE_LOOP ( 'NONE', ( #8630, #17375 ) ) ;
#11303=EDGE_CURVE ( 'NONE', #18665, #26232, #24443, .T. ) ;
#11310=DIRECTION ( 'NONE',  ( 0.3064653112860303286, -0.9430444279530931784, -0.1294071863730131000 ) ) ;
#11313=ORIENTED_EDGE ( 'NONE', *, *, #27972, .F. ) ;
#11317=ORIENTED_EDGE ( 'NONE', *, *, #2949, .F. ) ;
#11318=CIRCLE ( 'NONE', #20656, 1.499999999999999556 ) ;
#11320=CARTESIAN_POINT ( 'NONE',  ( -21.99312410279999952, -80.25114227570000480, -32.51123870579999675 ) ) ;
#11321=CARTESIAN_POINT ( 'NONE',  ( 8.655529603599999788, -36.72098037409999449, -21.58808908319999986 ) ) ;
#11328=CARTESIAN_POINT ( 'NONE',  ( -40.30304758909999663, -74.34471143260000758, 7.255215663249999558 ) ) ;
#11330=CARTESIAN_POINT ( 'NONE',  ( -1.981473163410000016, -57.45864773929999814, -23.83876219520000106 ) ) ;
#11331=AXIS2_PLACEMENT_3D ( 'NONE', #14501, #23960, #7950 ) ;
#11333=CARTESIAN_POINT ( 'NONE',  ( -7.489111472456650098, -73.99989317614092954, 38.95197877120744323 ) ) ;
#11334=CARTESIAN_POINT ( 'NONE',  ( 25.26718046270000073, -19.50000000000000000, 6.129403842640000377 ) ) ;
#11335=ORIENTED_EDGE ( 'NONE', *, *, #18906, .F. ) ;
#11338=CARTESIAN_POINT ( 'NONE',  ( 22.29272167939999960, -65.04696937989999128, 11.61829170020000035 ) ) ;
#11339=CARTESIAN_POINT ( 'NONE',  ( 8.987515397540001061, -35.19375992660000207, -19.46719241160000280 ) ) ;
#11342=CARTESIAN_POINT ( 'NONE',  ( 46.47110230210000026, -80.14094940709999548, -3.615576172169999936 ) ) ;
#11346=CARTESIAN_POINT ( 'NONE',  ( -11.81933340930000043, -64.47176828549999072, -23.20996066840000083 ) ) ;
#11347=CARTESIAN_POINT ( 'NONE',  ( -40.00000000000000000, -69.00000000000000000, -9.436895709309999441E-17 ) ) ;
#11348=ORIENTED_EDGE ( 'NONE', *, *, #7699, .F. ) ;
#11350=ORIENTED_EDGE ( 'NONE', *, *, #15006, .T. ) ;
#11351=CARTESIAN_POINT ( 'NONE',  ( -11.85013948020000107, -42.26697439500000542, 19.76414738429999929 ) ) ;
#11353=ORIENTED_EDGE ( 'NONE', *, *, #2410, .F. ) ;
#11354=CARTESIAN_POINT ( 'NONE',  ( 9.165580245683250027, -36.00000000019999646, -20.59810122320078918 ) ) ;
#11357=CARTESIAN_POINT ( 'NONE',  ( 25.94817478915412323, -70.08538442660875489, -8.904232401822897103 ) ) ;
#11358=CIRCLE ( 'NONE', #10877, 7.250000000000000000 ) ;
#11359=CARTESIAN_POINT ( 'NONE',  ( -10.17458377400000025, -18.50000000000000000, -22.50859265919999785 ) ) ;
#11360=CARTESIAN_POINT ( 'NONE',  ( 21.52064452127972416, -37.42737532315320692, -7.718013524113811918 ) ) ;
#11361=ORIENTED_EDGE ( 'NONE', *, *, #9170, .F. ) ;
#11365=ORIENTED_EDGE ( 'NONE', *, *, #19241, .T. ) ;
#11366=AXIS2_PLACEMENT_3D ( 'NONE', #21226, #25602, #14513 ) ;
#11367=CARTESIAN_POINT ( 'NONE',  ( 19.69582338720000081, -18.50000000000000000, -7.383548592259999488 ) ) ;
#11369=CARTESIAN_POINT ( 'NONE',  ( -14.19188855770000046, -80.00000000000000000, 37.13021410070000883 ) ) ;
#11371=EDGE_CURVE ( 'NONE', #5907, #17770, #16778, .T. ) ;
#11375=CARTESIAN_POINT ( 'NONE',  ( 23.94732912799409164, -74.14839568665851743, -30.91612537757790946 ) ) ;
#11379=DIRECTION ( 'NONE',  ( 0.000000000000000000, 1.000000000000000000, 0.000000000000000000 ) ) ;
#11380=ORIENTED_EDGE ( 'NONE', *, *, #23181, .F. ) ;
#11384=LINE ( 'NONE', #6895, #5136 ) ;
#11385=ORIENTED_EDGE ( 'NONE', *, *, #24381, .T. ) ;
#11386=CARTESIAN_POINT ( 'NONE',  ( 7.314390784529999578, -73.97626148509999666, 39.54176628510000313 ) ) ;
#11392=AXIS2_PLACEMENT_3D ( 'NONE', #21496, #21637, #23965 ) ;
#11393=CARTESIAN_POINT ( 'NONE',  ( 27.02127222293052711, -72.26362179314627099, -11.39336057284735659 ) ) ;
#11394=CARTESIAN_POINT ( 'NONE',  ( 8.981104793960000165, -36.05511643379999498, -20.59303662420000336 ) ) ;
#11395=CARTESIAN_POINT ( 'NONE',  ( 45.84677420395677672, -73.65707963207451314, -4.286925635858382932 ) ) ;
#11399=CARTESIAN_POINT ( 'NONE',  ( -2.552536252342168410, -19.48522775728675072, -23.44697642559193085 ) ) ;
#11403=EDGE_CURVE ( 'NONE', #7122, #24982, #23351, .T. ) ;
#11407=CARTESIAN_POINT ( 'NONE',  ( -12.37736070569999924, -67.43115654220000010, -23.30866868589999896 ) ) ;
#11410=ORIENTED_EDGE ( 'NONE', *, *, #18709, .F. ) ;
#11411=CARTESIAN_POINT ( 'NONE',  ( -32.25191193603353668, -80.23900669782145201, -22.46351872105675440 ) ) ;
#11413=AXIS2_PLACEMENT_3D ( 'NONE', #23124, #23405, #3445 ) ;
#11415=CARTESIAN_POINT ( 'NONE',  ( -12.32689411409999991, -62.06831188909999497, 20.76176652019999835 ) ) ;
#11416=DIRECTION ( 'NONE',  ( 0.000000000000000000, 1.000000000000000000, 0.000000000000000000 ) ) ;
#11417=CARTESIAN_POINT ( 'NONE',  ( 20.06309763089999620, -36.00000000000000000, -9.476129751679998492 ) ) ;
#11418=CARTESIAN_POINT ( 'NONE',  ( 21.20403895319999776, -36.23955850830000003, -8.971066259000000542 ) ) ;
#11419=CARTESIAN_POINT ( 'NONE',  ( 6.015370493379999656E-15, -69.50000000000000000, -40.00000000000000000 ) ) ;
#11420=EDGE_CURVE ( 'NONE', #3267, #452, #1176, .T. ) ;
#11421=CARTESIAN_POINT ( 'NONE',  ( 46.25000000000000000, -75.00000000000000000, -7.375000000000000000 ) ) ;
#11422=VERTEX_POINT ( 'NONE', #6338 ) ;
#11423=CARTESIAN_POINT ( 'NONE',  ( -7.252015964940000003, -74.29298176469998793, -40.34085930499999506 ) ) ;
#11424=CARTESIAN_POINT ( 'NONE',  ( 29.28445555986126791, -74.32986215128055107, -26.08911349325367723 ) ) ;
#11426=ORIENTED_EDGE ( 'NONE', *, *, #6622, .F. ) ;
#11431=TOROIDAL_SURFACE ( 'NONE', #25431, 3.750000000000000000, 1.000000000000000000 ) ;
#11434=CARTESIAN_POINT ( 'NONE',  ( 19.84950935299999841, -19.15770089200000115, 9.820435146359999479 ) ) ;
#11435=CARTESIAN_POINT ( 'NONE',  ( 10.35051949290000017, -65.80242602599999202, -25.33509568779999910 ) ) ;
#11438=DIRECTION ( 'NONE',  ( 0.000000000000000000, 1.000000000000000000, 0.000000000000000000 ) ) ;
#11440=APPLICATION_CONTEXT ( 'automotive_design' ) ;
#11442=CARTESIAN_POINT ( 'NONE',  ( 23.30839594958685268, -63.38792371584848695, -7.455862079869596926 ) ) ;
#11445=ORIENTED_EDGE ( 'NONE', *, *, #23047, .F. ) ;
#11446=B_SPLINE_CURVE_WITH_KNOTS ( 'NONE', 3,
 ( #19818, #28696, #22167, #8736, #2207, #26534, #17653, #8885, #26688, #6729 ),
 .UNSPECIFIED., .F., .F.,
 ( 4, 2, 2, 2, 4 ),
 ( 0.000000000000000000, 0.2500000000000000000, 0.5000000000000000000, 0.7500000000000000000, 1.000000000000000000 ),
 .UNSPECIFIED. ) ;
#11447=CARTESIAN_POINT ( 'NONE',  ( -10.80933341492661448, -19.49660160594845948, -21.71230118854520796 ) ) ;
#11448=CARTESIAN_POINT ( 'NONE',  ( -41.00000000000000000, -74.50000000000000000, 10.20110288159999890 ) ) ;
#11452=EDGE_CURVE ( 'NONE', #3127, #27117, #2407, .T. ) ;
#11453=ORIENTED_EDGE ( 'NONE', *, *, #26379, .F. ) ;
#11455=CARTESIAN_POINT ( 'NONE',  ( -13.02626867543477829, -71.94658701398387279, -25.10627575233144171 ) ) ;
#11456=CARTESIAN_POINT ( 'NONE',  ( 10.55611696420000101, -36.00000000000000000, -20.94239052940000079 ) ) ;
#11457=VERTEX_POINT ( 'NONE', #4447 ) ;
#11458=CARTESIAN_POINT ( 'NONE',  ( 7.239953483535906287, -73.75061506092028196, -39.61603006814522843 ) ) ;
#11459=CARTESIAN_POINT ( 'NONE',  ( -22.13232311830000043, -79.50000004279999644, -32.73892520679999762 ) ) ;
#11466=ORIENTED_EDGE ( 'NONE', *, *, #8004, .T. ) ;
#11468=CARTESIAN_POINT ( 'NONE',  ( 36.32677412860000032, -74.12275851199999011, -14.57143996970000011 ) ) ;
#11469=CARTESIAN_POINT ( 'NONE',  ( -2.595652345209999989, -59.96629798200000039, -25.39846653560000078 ) ) ;
#11470=CARTESIAN_POINT ( 'NONE',  ( -40.35962647450000418, -74.26791556530000094, 7.250123090889999844 ) ) ;
#11471=CARTESIAN_POINT ( 'NONE',  ( -21.74262969930000011, -74.09723562380000317, -32.46276855370000192 ) ) ;
#11473=CARTESIAN_POINT ( 'NONE',  ( 27.19594722837873491, -66.52176723538890712, 1.775342338193904856 ) ) ;
#11474=CARTESIAN_POINT ( 'NONE',  ( -7.371519361690793026, -73.99966369223987783, 39.28661307825520055 ) ) ;
#11475=CARTESIAN_POINT ( 'NONE',  ( -18.92688961970000250, -18.86472494539999900, 14.06132894319999949 ) ) ;
#11478=CARTESIAN_POINT ( 'NONE',  ( 23.92242908059999706, -63.31646347429999366, 10.69554000200000132 ) ) ;
#11479=CARTESIAN_POINT ( 'NONE',  ( 7.969906462720000029, -35.15970427070000426, -21.19871012420000156 ) ) ;
#11483=CARTESIAN_POINT ( 'NONE',  ( 45.84677419350000349, -80.34292036729999609, -4.286925650119999709 ) ) ;
#11484=B_SPLINE_SURFACE_WITH_KNOTS ( 'NONE', 5, 5, ( 
 ( #19013, #28303, #3702, #28174, #10237, #12564 ),
 ( #19151, #8337, #1670, #17097, #17242, #26134 ),
 ( #6157, #21203, #1126, #7801, #27892, #16826 ),
 ( #14629, #23528, #19992, #21900, #4265, #28723 ),
 ( #26714, #65, #8485, #13286, #10793, #8911 ),
 ( #8761, #26417, #15311, #6303, #26563, #13138 ) ),
 .UNSPECIFIED., .F., .F., .F.,
 ( 6, 6 ),
 ( 6, 6 ),
 ( 43.40831274110000493, 64.87293781390000902 ),
 ( 0.000000000000000000, 2.000000000000000000 ),
 .UNSPECIFIED. ) ;
#11485=CARTESIAN_POINT ( 'NONE',  ( -11.53845963589999890, -61.97075362790000241, -21.57078944089999695 ) ) ;
#11486=CARTESIAN_POINT ( 'NONE',  ( 26.27227914920000273, -70.89666188759998988, -10.69275250369999952 ) ) ;
#11489=AXIS2_PLACEMENT_3D ( 'NONE', #22193, #20149, #13289 ) ;
#11490=CARTESIAN_POINT ( 'NONE',  ( -14.65665286289999969, -74.50000000000000000, 36.94583910070000599 ) ) ;
#11493=CARTESIAN_POINT ( 'NONE',  ( -13.91350890449018962, -18.60777309624396381, 20.23952179938335050 ) ) ;
#11495=ORIENTED_EDGE ( 'NONE', *, *, #28319, .F. ) ;
#11497=CARTESIAN_POINT ( 'NONE',  ( 41.00000000000000000, -84.50000000000000000, 10.20110288159999890 ) ) ;
#11499=AXIS2_PLACEMENT_3D ( 'NONE', #22070, #2119, #529 ) ;
#11504=CARTESIAN_POINT ( 'NONE',  ( -10.65197422049999965, -18.62337009750000050, -22.10007990119999732 ) ) ;
#11505=DIRECTION ( 'NONE',  ( 0.000000000000000000, 1.000000000000000000, 0.000000000000000000 ) ) ;
#11506=ORIENTED_EDGE ( 'NONE', *, *, #22626, .T. ) ;
#11508=CYLINDRICAL_SURFACE ( 'NONE', #10172, 4.750000000000000888 ) ;
#11512=CARTESIAN_POINT ( 'NONE',  ( 19.93551599202017499, -18.49999999997239186, -7.473404292298043039 ) ) ;
#11514=DIRECTION ( 'NONE',  ( 0.000000000000000000, 1.000000000000000000, 0.000000000000000000 ) ) ;
#11515=VERTEX_POINT ( 'NONE', #5465 ) ;
#11517=CARTESIAN_POINT ( 'NONE',  ( -19.41484581850000168, -39.36519097789999933, 11.81754271080000152 ) ) ;
#11518=CARTESIAN_POINT ( 'NONE',  ( 7.279266295386986663, -36.17014819251620850, -21.46816513959021222 ) ) ;
#11519=CARTESIAN_POINT ( 'NONE',  ( -13.16184031329999904, -70.12921433920000425, -24.09257711200000074 ) ) ;
#11521=CARTESIAN_POINT ( 'NONE',  ( 27.08636525929999905, -66.18149755910000920, 1.733009796709999994 ) ) ;
#11526=CARTESIAN_POINT ( 'NONE',  ( -37.60355029590000697, -84.50000000000000000, 9.356041104380000917 ) ) ;
#11527=DIRECTION ( 'NONE',  ( 0.5439177849611214199, 0.000000000000000000, -0.8391385125251892285 ) ) ;
#11530=ORIENTED_EDGE ( 'NONE', *, *, #26572, .T. ) ;
#11531=CARTESIAN_POINT ( 'NONE',  ( 7.432602092569998931, -73.95640471630001400, 39.04179453189999549 ) ) ;
#11533=ADVANCED_FACE ( 'NONE', ( #21068 ), #11484, .T. ) ;
#11535=CARTESIAN_POINT ( 'NONE',  ( 21.19011208810000113, -36.03998686679999963, -8.396978594420000164 ) ) ;
#11536=AXIS2_PLACEMENT_3D ( 'NONE', #3919, #2, #12784 ) ;
#11538=CARTESIAN_POINT ( 'NONE',  ( 8.753883147839999879, -36.52594017789999725, -21.30736199240000062 ) ) ;
#11539=EDGE_CURVE ( 'NONE', #10505, #22467, #10271, .T. ) ;
#11540=CARTESIAN_POINT ( 'NONE',  ( 46.12332288492410015, -73.99999999901751835, -4.489694478895246199 ) ) ;
#11545=CARTESIAN_POINT ( 'NONE',  ( -12.77867724610393552, -19.48040540344112870, 19.46310901654912584 ) ) ;
#11547=CARTESIAN_POINT ( 'NONE',  ( -2.645789240093490591, -19.49660179754663858, -24.10947003643325814 ) ) ;
#11549=CARTESIAN_POINT ( 'NONE',  ( -2.127492191069999983, -26.08233090739999938, -22.84993033459999978 ) ) ;
#11551=CARTESIAN_POINT ( 'NONE',  ( -39.32889484840046634, -73.62261561668437082, 7.218875474177834484 ) ) ;
#11552=CARTESIAN_POINT ( 'NONE',  ( 21.78580818603761671, -37.64222968075310405, -8.476164595188171447 ) ) ;
#11555=CARTESIAN_POINT ( 'NONE',  ( -37.60355029590000697, -74.50000000000000000, -9.356041104380000917 ) ) ;
#11557=CARTESIAN_POINT ( 'NONE',  ( -32.40381740377279840, -80.05388657958994258, -22.56932125262067856 ) ) ;
#11558=AXIS2_PLACEMENT_3D ( 'NONE', #23403, #3443, #12310 ) ;
#11560=CARTESIAN_POINT ( 'NONE',  ( -13.99699122829999887, -67.43047917469999675, 22.37324552669999989 ) ) ;
#11561=CARTESIAN_POINT ( 'NONE',  ( -13.71875444750000028, -58.84831425530000359, 21.01328297090000063 ) ) ;
#11562=DIRECTION ( 'NONE',  ( 1.000000000000000000, 0.000000000000000000, 0.000000000000000000 ) ) ;
#11563=DIRECTION ( 'NONE',  ( 0.000000000000000000, -1.000000000000000000, 0.000000000000000000 ) ) ;
#11565=EDGE_CURVE ( 'NONE', #17228, #14724, #11683, .T. ) ;
#11566=CARTESIAN_POINT ( 'NONE',  ( -11.37119059761108453, -49.51244866342480577, -22.45585869990737393 ) ) ;
#11567=ORIENTED_EDGE ( 'NONE', *, *, #1880, .T. ) ;
#11569=CARTESIAN_POINT ( 'NONE',  ( 30.27730015304011957, -74.21788658106061121, -24.84071712252042730 ) ) ;
#11570=EDGE_CURVE ( 'NONE', #9669, #13629, #2895, .T. ) ;
#11576=CARTESIAN_POINT ( 'NONE',  ( 21.50956136779998573, -52.61368720119948250, 10.11639787089999132 ) ) ;
#11578=AXIS2_PLACEMENT_3D ( 'NONE', #14635, #23531, #14899 ) ;
#11579=CARTESIAN_POINT ( 'NONE',  ( 36.28164458690000060, -74.50000000000000000, -14.97346873880000118 ) ) ;
#11580=CARTESIAN_POINT ( 'NONE',  ( -7.242474372567466290, -73.77182148726545563, -39.65872146218941907 ) ) ;
#11581=FACE_OUTER_BOUND ( 'NONE', #6559, .T. ) ;
#11582=CARTESIAN_POINT ( 'NONE',  ( -21.64068549270000119, -66.52838475369999571, 15.77032591200000233 ) ) ;
#11585=CARTESIAN_POINT ( 'NONE',  ( -12.54443447719999938, -72.70510876110000709, -25.73426150890000130 ) ) ;
#11588=CARTESIAN_POINT ( 'NONE',  ( 21.58194535263011815, -19.48522775728685019, 9.512926974174723327 ) ) ;
#11595=AXIS2_PLACEMENT_3D ( 'NONE', #20778, #11563, #24991 ) ;
#11600=ORIENTED_EDGE ( 'NONE', *, *, #861, .F. ) ;
#11601=EDGE_CURVE ( 'NONE', #10333, #1165, #7992, .T. ) ;
#11602=ORIENTED_EDGE ( 'NONE', *, *, #11904, .F. ) ;
#11604=CARTESIAN_POINT ( 'NONE',  ( 21.48399581230000166, -36.52810941199999917, -9.014522560119999639 ) ) ;
#11605=CARTESIAN_POINT ( 'NONE',  ( 47.13175990429999729, -74.43591472970000211, -1.325790583919999932 ) ) ;
#11606=EDGE_LOOP ( 'NONE', ( #11040, #18647, #18316, #16333 ) ) ;
#11607=CARTESIAN_POINT ( 'NONE',  ( 7.243236069894179785, -73.78481856924898352, -39.68146194261722570 ) ) ;
#11608=CARTESIAN_POINT ( 'NONE',  ( -11.76147443210928500, -63.18033547063078714, 21.37881495694788825 ) ) ;
#11610=CARTESIAN_POINT ( 'NONE',  ( -2.889377628239999662, -70.54208558220000214, -27.60766051819999944 ) ) ;
#11611=FACE_OUTER_BOUND ( 'NONE', #11809, .T. ) ;
#11612=CARTESIAN_POINT ( 'NONE',  ( -15.78701019289999863, -72.82938648530000592, 23.94860758740000151 ) ) ;
#11614=CIRCLE ( 'NONE', #27922, 4.750000000000000000 ) ;
#11615=AXIS2_PLACEMENT_3D ( 'NONE', #27518, #5637, #1284 ) ;
#11616=CARTESIAN_POINT ( 'NONE',  ( 36.39327240949999975, -74.35351771279999866, -14.75026165080000062 ) ) ;
#11618=CARTESIAN_POINT ( 'NONE',  ( -21.99449553610000052, -74.01681409379999366, -32.14594688369999886 ) ) ;
#11619=EDGE_LOOP ( 'NONE', ( #1866, #15166, #22835, #14436 ) ) ;
#11621=CARTESIAN_POINT ( 'NONE',  ( -7.458790909887997422, -73.99982286725833092, 39.02883428035619318 ) ) ;
#11623=ORIENTED_EDGE ( 'NONE', *, *, #17062, .F. ) ;
#11626=CARTESIAN_POINT ( 'NONE',  ( 21.46759780150000196, -62.96338283689998860, 11.34255856240000071 ) ) ;
#11627=CARTESIAN_POINT ( 'NONE',  ( 8.043104929030000960, -34.87912771779999588, -21.12346526210000164 ) ) ;
#11630=ORIENTED_EDGE ( 'NONE', *, *, #27694, .T. ) ;
#11631=CARTESIAN_POINT ( 'NONE',  ( 47.25063473080000165, -79.41040171960000293, -0.8747163666420000316 ) ) ;
#11633=CARTESIAN_POINT ( 'NONE',  ( -11.12754515849999848, -19.46434200899999922, 19.08244047510000030 ) ) ;
#11634=CARTESIAN_POINT ( 'NONE',  ( -11.63050495949999963, -60.55397095009999475, -20.76951049480000222 ) ) ;
#11635=EDGE_CURVE ( 'NONE', #7412, #24358, #6552, .T. ) ;
#11636=AXIS2_PLACEMENT_3D ( 'NONE', #25002, #14075, #554 ) ;
#11637=DIRECTION ( 'NONE',  ( -1.000000000000000000, 0.000000000000000000, 6.308085367188389255E-16 ) ) ;
#11640=ORIENTED_EDGE ( 'NONE', *, *, #19460, .F. ) ;
#11643=ORIENTED_EDGE ( 'NONE', *, *, #22594, .T. ) ;
#11644=CARTESIAN_POINT ( 'NONE',  ( -13.46188194249999981, -19.39368401379999796, 20.39616198339999897 ) ) ;
#11645=CARTESIAN_POINT ( 'NONE',  ( -21.83908241200000333, -74.03505044649999434, -32.25228936610000119 ) ) ;
#11647=CARTESIAN_POINT ( 'NONE',  ( 45.84677419350000349, -80.50000000000000000, -4.286925650119999709 ) ) ;
#11648=CARTESIAN_POINT ( 'NONE',  ( 22.82319683875572736, -42.27314267049876406, -0.5642692666673589930 ) ) ;
#11649=CARTESIAN_POINT ( 'NONE',  ( -10.48404752216234570, -19.47261270939580058, -20.20374288751023428 ) ) ;
#11650=CARTESIAN_POINT ( 'NONE',  ( -3.577689640331730203, -19.50000000000000000, -25.07857796645360793 ) ) ;
#11652=CARTESIAN_POINT ( 'NONE',  ( 21.65968896626973361, -37.88705161499458995, -8.203619567505477050 ) ) ;
#11653=ORIENTED_EDGE ( 'NONE', *, *, #9575, .F. ) ;
#11654=CARTESIAN_POINT ( 'NONE',  ( -32.67527180329999936, -79.50000000000000000, -22.00249031559999935 ) ) ;
#11660=FACE_OUTER_BOUND ( 'NONE', #28193, .T. ) ;
#11661=DIRECTION ( 'NONE',  ( 0.000000000000000000, -1.000000000000000000, 0.000000000000000000 ) ) ;
#11667=CARTESIAN_POINT ( 'NONE',  ( -19.96385611919999903, -52.58489974409999945, 14.40794232450000045 ) ) ;
#11668=CARTESIAN_POINT ( 'NONE',  ( -36.59277592640000165, -79.50000000000000000, -25.98617420859999783 ) ) ;
#11669=DIRECTION ( 'NONE',  ( 0.000000000000000000, 1.000000000000000000, 0.000000000000000000 ) ) ;
#11671=CARTESIAN_POINT ( 'NONE',  ( -14.93121066289999987, -74.50000000000000000, 36.29905574720000061 ) ) ;
#11672=EDGE_CURVE ( 'NONE', #12707, #22756, #9382, .T. ) ;
#11674=EDGE_CURVE ( 'NONE', #3120, #8180, #18212, .T. ) ;
#11676=VERTEX_POINT ( 'NONE', #10119 ) ;
#11681=CARTESIAN_POINT ( 'NONE',  ( 7.252015964940000003, -74.29298176469998793, 40.34085930499999506 ) ) ;
#11682=CARTESIAN_POINT ( 'NONE',  ( 7.880018115929998679, -18.50000000000000000, -19.31987738409999977 ) ) ;
#11683=CIRCLE ( 'NONE', #6597, 7.750000000000000000 ) ;
#11685=CARTESIAN_POINT ( 'NONE',  ( 21.47791241899999903, -36.56811125080000835, -7.356933755090000027 ) ) ;
#11687=FACE_OUTER_BOUND ( 'NONE', #17889, .T. ) ;
#11688=CARTESIAN_POINT ( 'NONE',  ( -17.42343749999999858, -74.50000000000000000, 43.92022684009999978 ) ) ;
#11689=CARTESIAN_POINT ( 'NONE',  ( 9.104027697630002081, -35.96031139400000143, -20.29387716869999991 ) ) ;
#11695=EDGE_LOOP ( 'NONE', ( #11506, #16279, #2270, #24002, #22506 ) ) ;
#11696=DIRECTION ( 'NONE',  ( 0.4794255386042040601, 0.000000000000000000, 0.8775825618903720926 ) ) ;
#11698=CARTESIAN_POINT ( 'NONE',  ( -0.5268692886119999974, -39.36519097800000111, -22.72252104480000057 ) ) ;
#11700=CYLINDRICAL_SURFACE ( 'NONE', #21622, 4.749999999999999112 ) ;
#11702=CARTESIAN_POINT ( 'NONE',  ( 22.26662627820000040, -57.47855601759999900, -7.066909182049999849 ) ) ;
#11706=EDGE_LOOP ( 'NONE', ( #11001, #24331, #4597 ) ) ;
#11707=VECTOR ( 'NONE', #23030, 1000.000000000000000 ) ;
#11709=CARTESIAN_POINT ( 'NONE',  ( 36.47289859480000729, -74.92271630800000537, -14.78463751350000166 ) ) ;
#11711=CARTESIAN_POINT ( 'NONE',  ( -32.77174707999999725, -79.50000000000000000, -21.60034937969999902 ) ) ;
#11714=CARTESIAN_POINT ( 'NONE',  ( 20.49277737539999933, -35.23997945060000347, -8.776869873949999956 ) ) ;
#11715=CARTESIAN_POINT ( 'NONE',  ( 7.250083186822952719, -73.98707088500670181, 40.01432744662073304 ) ) ;
#11716=CARTESIAN_POINT ( 'NONE',  ( -2.363861431290001924, -52.59522851919944486, -24.20187825489998090 ) ) ;
#11717=CARTESIAN_POINT ( 'NONE',  ( 21.58808931389999586, -36.72098037479999988, -8.655529985299999396 ) ) ;
#11722=ORIENTED_EDGE ( 'NONE', *, *, #14908, .T. ) ;
#11723=B_SPLINE_CURVE_WITH_KNOTS ( 'NONE', 5,
 ( #6944, #18306, #26905, #7094, #11576, #20041, #11729, #2279, #22383 ),
 .UNSPECIFIED., .F., .F.,
 ( 6, 3, 6 ),
 ( 0.000000000000000000, 0.5000000000000000000, 1.000000000000000000 ),
 .UNSPECIFIED. ) ;
#11726=EDGE_LOOP ( 'NONE', ( #7213, #5403, #21858, #24708 ) ) ;
#11729=CARTESIAN_POINT ( 'NONE',  ( 22.45957212889998189, -52.58489974409948076, 10.08523539449999085 ) ) ;
#11731=DIRECTION ( 'NONE',  ( 0.9704142011833034598, 0.000000000000000000, 0.2414462220490750377 ) ) ;
#11732=CARTESIAN_POINT ( 'NONE',  ( -7.169550435265128030, -73.50000000000004263, -38.90587669234852797 ) ) ;
#11733=CARTESIAN_POINT ( 'NONE',  ( -14.10481785270000010, -74.02367878169998505, 36.45432549239999531 ) ) ;
#11734=CARTESIAN_POINT ( 'NONE',  ( 9.720248444560001033, -72.82938969829999110, -26.98670033600000195 ) ) ;
#11735=CARTESIAN_POINT ( 'NONE',  ( -13.47268409989999860, -20.68842595469999779, 20.42652994440000214 ) ) ;
#11738=CARTESIAN_POINT ( 'NONE',  ( -11.95864023049999858, -71.65979788389999783, -26.06651585250000025 ) ) ;
#11739=FACE_OUTER_BOUND ( 'NONE', #21510, .T. ) ;
#11741=DIRECTION ( 'NONE',  ( 0.000000000000000000, 1.000000000000000000, 0.000000000000000000 ) ) ;
#11747=ORIENTED_EDGE ( 'NONE', *, *, #11997, .T. ) ;
#11748=AXIS2_PLACEMENT_3D ( 'NONE', #23873, #23729, #3772 ) ;
#11750=CARTESIAN_POINT ( 'NONE',  ( 0.000000000000000000, -56.78056608349999834, 0.000000000000000000 ) ) ;
#11753=ORIENTED_EDGE ( 'NONE', *, *, #24082, .F. ) ;
#11754=VERTEX_POINT ( 'NONE', #23409 ) ;
#11759=CARTESIAN_POINT ( 'NONE',  ( 7.215638845179813465, -73.61009970497924826, -39.29494613562393113 ) ) ;
#11760=CARTESIAN_POINT ( 'NONE',  ( -11.63271255370046831, -62.50667214630417590, 21.20421611403313022 ) ) ;
#11762=B_SPLINE_CURVE_WITH_KNOTS ( 'NONE', 5,
 ( #1816, #19577, #26293, #15178, #4130, #13004 ),
 .UNSPECIFIED., .F., .F.,
 ( 6, 6 ),
 ( 0.000000000000000000, 1.000000000000000000 ),
 .UNSPECIFIED. ) ;
#11763=EDGE_CURVE ( 'NONE', #19780, #14378, #19853, .T. ) ;
#11764=CARTESIAN_POINT ( 'NONE',  ( -4.062024957338500109, -70.93524644749820141, -28.43407472284975412 ) ) ;
#11766=CARTESIAN_POINT ( 'NONE',  ( -4.459622768110000024, -72.00000000000000000, -28.73485779310000154 ) ) ;
#11767=CIRCLE ( 'NONE', #20632, 0.5000000000000004441 ) ;
#11768=CARTESIAN_POINT ( 'NONE',  ( -11.18243144779999909, -57.47855601759999900, 20.51090144570000007 ) ) ;
#11770=CARTESIAN_POINT ( 'NONE',  ( 7.460698725479999927E-15, -74.00000000000000000, 40.00000000000000000 ) ) ;
#11772=CARTESIAN_POINT ( 'NONE',  ( 23.61566637130000146, -60.59571585039999775, -0.5691291156790000416 ) ) ;
#11773=CARTESIAN_POINT ( 'NONE',  ( -21.99377254480000232, -74.28769487450000497, -32.60949123969999874 ) ) ;
#11774=ORIENTED_EDGE ( 'NONE', *, *, #11200, .T. ) ;
#11775=CARTESIAN_POINT ( 'NONE',  ( 26.46310988749999993, -64.24504445130001784, 1.532420830840000026 ) ) ;
#11782=CARTESIAN_POINT ( 'NONE',  ( 21.06982195980000228, -60.33243244399999128, 10.82665592080000216 ) ) ;
#11786=ORIENTED_EDGE ( 'NONE', *, *, #2613, .T. ) ;
#11787=CARTESIAN_POINT ( 'NONE',  ( 20.49588873660000132, -52.63280639819999607, 10.85734681379999955 ) ) ;
#11788=EDGE_CURVE ( 'NONE', #10257, #6300, #19041, .T. ) ;
#11789=CARTESIAN_POINT ( 'NONE',  ( -11.41403033759999985, -60.27227161350000273, -22.50529123499999784 ) ) ;
#11790=CARTESIAN_POINT ( 'NONE',  ( 37.26113007297411883, -80.00000001582722575, -13.81325807140697037 ) ) ;
#11794=VERTEX_POINT ( 'NONE', #19035 ) ;
#11796=ORIENTED_EDGE ( 'NONE', *, *, #14473, .T. ) ;
#11797=CARTESIAN_POINT ( 'NONE',  ( 20.34628061899999807, -52.63293862069999562, 11.13082833170000008 ) ) ;
#11798=CARTESIAN_POINT ( 'NONE',  ( -21.65925653600000444, -74.22385006870000268, -32.64405417670000276 ) ) ;
#11801=CARTESIAN_POINT ( 'NONE',  ( 47.25000000000000000, -77.00000000000000000, 7.327133149349999745E-15 ) ) ;
#11802=EDGE_CURVE ( 'NONE', #7860, #26269, #18759, .T. ) ;
#11803=AXIS2_PLACEMENT_3D ( 'NONE', #25003, #5038, #4756 ) ;
#11805=CARTESIAN_POINT ( 'NONE',  ( -10.44824884758171457, -19.47630530571390750, -20.50788404414224786 ) ) ;
#11806=DIRECTION ( 'NONE',  ( -0.9704142011833033488, 0.000000000000000000, -0.2414462220490755373 ) ) ;
#11808=CARTESIAN_POINT ( 'NONE',  ( 47.19127288053609703, -79.33764839652816647, -1.165204315948687119 ) ) ;
#11809=EDGE_LOOP ( 'NONE', ( #26084, #24781, #473, #2294 ) ) ;
#11810=CARTESIAN_POINT ( 'NONE',  ( -32.48908668560000024, -80.00000024250000763, -22.62871150349999638 ) ) ;
#11814=AXIS2_PLACEMENT_3D ( 'NONE', #14375, #18898, #16413 ) ;
#11817=DIRECTION ( 'NONE',  ( 0.000000000000000000, -1.000000000000000000, 0.000000000000000000 ) ) ;
#11818=ORIENTED_EDGE ( 'NONE', *, *, #2493, .F. ) ;
#11820=CARTESIAN_POINT ( 'NONE',  ( -19.65068252670000248, -52.63280639819999607, 12.32128691209999971 ) ) ;
#11821=LINE ( 'NONE', #25099, #17019 ) ;
#11823=CARTESIAN_POINT ( 'NONE',  ( 23.52622274289999638, -57.40875708169999569, -9.564507863490000261 ) ) ;
#11825=CARTESIAN_POINT ( 'NONE',  ( 26.32473474220000043, -67.65187322490000099, 0.01358298500609999779 ) ) ;
#11828=DIRECTION ( 'NONE',  ( 0.000000000000000000, 1.000000000000000000, 0.000000000000000000 ) ) ;
#11832=DIRECTION ( 'NONE',  ( 0.000000000000000000, 0.000000000000000000, -1.000000000000000000 ) ) ;
#11835=DIRECTION ( 'NONE',  ( 0.000000000000000000, -1.000000000000000000, 0.000000000000000000 ) ) ;
#11837=CARTESIAN_POINT ( 'NONE',  ( 26.85202045726772013, -72.75638125331757067, -10.08991345884111723 ) ) ;
#11840=LINE ( 'NONE', #7497, #24329 ) ;
#11843=EDGE_CURVE ( 'NONE', #23734, #7833, #25103, .T. ) ;
#11844=CARTESIAN_POINT ( 'NONE',  ( -39.95935625357012100, -73.95086734775428283, 7.250038883934483813 ) ) ;
#11845=CARTESIAN_POINT ( 'NONE',  ( 24.58030493329999899, -18.50000000000000000, 2.442848308399999890 ) ) ;
#11849=CARTESIAN_POINT ( 'NONE',  ( -2.552856939384906543, -19.48524588020510961, -23.44805131028554968 ) ) ;
#11850=ADVANCED_FACE ( 'NONE', ( #19312 ), #19474, .T. ) ;
#11852=DIRECTION ( 'NONE',  ( -0.09362217723111272705, 0.000000000000000000, 0.9956077982471339682 ) ) ;
#11856=DIRECTION ( 'NONE',  ( 0.000000000000000000, 1.000000000000000000, 0.000000000000000000 ) ) ;
#11857=CARTESIAN_POINT ( 'NONE',  ( 21.60733108839999872, -40.74566548650000186, -7.843434090929999769 ) ) ;
#11859=DIRECTION ( 'NONE',  ( 0.9704142011833034598, 0.000000000000000000, 0.2414462220490750377 ) ) ;
#11860=ORIENTED_EDGE ( 'NONE', *, *, #16271, .T. ) ;
#11861=DIRECTION ( 'NONE',  ( 0.000000000000000000, 1.000000000000000000, 0.000000000000000000 ) ) ;
#11863=AXIS2_PLACEMENT_3D ( 'NONE', #24928, #15874, #766 ) ;
#11864=CARTESIAN_POINT ( 'NONE',  ( -13.17386516979999911, -67.65118726130000937, 22.79090083579999870 ) ) ;
#11865=CARTESIAN_POINT ( 'NONE',  ( 20.80006503139999907, -34.76181304210000178, -8.489266088069999938 ) ) ;
#11866=CARTESIAN_POINT ( 'NONE',  ( 7.198125313966591499, -73.54003775238612661, 39.10791602262280975 ) ) ;
#11867=AXIS2_PLACEMENT_3D ( 'NONE', #22655, #5165, #5009 ) ;
#11868=DIRECTION ( 'NONE',  ( -0.4692400087391613850, 0.000000000000000000, 0.8830706733883035842 ) ) ;
#11872=VERTEX_POINT ( 'NONE', #8095 ) ;
#11873=CYLINDRICAL_SURFACE ( 'NONE', #8243, 7.250000000000004441 ) ;
#11879=CARTESIAN_POINT ( 'NONE',  ( -7.342773311050000196, -74.12494612390000270, 39.65529513239999915 ) ) ;
#11884=CARTESIAN_POINT ( 'NONE',  ( -21.38368943589999915, -65.50129831189998697, 15.49162513829999988 ) ) ;
#11885=CARTESIAN_POINT ( 'NONE',  ( -13.60927699540000013, -35.85183931319999573, 20.77656409820000150 ) ) ;
#11887=CARTESIAN_POINT ( 'NONE',  ( -12.44921432620000168, -70.96097656259999553, -25.01534913949999961 ) ) ;
#11888=CARTESIAN_POINT ( 'NONE',  ( 7.718703860600000688, -22.46373279069999995, -20.74932018339999829 ) ) ;
#11890=DIRECTION ( 'NONE',  ( 0.000000000000000000, 1.000000000000000000, 0.000000000000000000 ) ) ;
#11892=VERTEX_POINT ( 'NONE', #6330 ) ;
#11893=EDGE_LOOP ( 'NONE', ( #13960, #7703, #8247 ) ) ;
#11896=FACE_OUTER_BOUND ( 'NONE', #10805, .T. ) ;
#11904=EDGE_CURVE ( 'NONE', #11872, #21465, #4594, .T. ) ;
#11906=ORIENTED_EDGE ( 'NONE', *, *, #17192, .F. ) ;
#11908=CARTESIAN_POINT ( 'NONE',  ( -12.07354857445369589, -64.51954438327166486, 21.77354567074241132 ) ) ;
#11911=CARTESIAN_POINT ( 'NONE',  ( 21.56931447779999900, -36.56979901409999911, -6.850353625240000355 ) ) ;
#11913=ADVANCED_FACE ( 'NONE', ( #24257 ), #20340, .T. ) ;
#11914=CARTESIAN_POINT ( 'NONE',  ( -3.967099564299999770, -72.37489743489999228, -28.45199697809999861 ) ) ;
#11916=VERTEX_POINT ( 'NONE', #28749 ) ;
#11918=CARTESIAN_POINT ( 'NONE',  ( -11.91266501540000000, -80.00000000000000000, 46.64429291560000479 ) ) ;
#11920=CARTESIAN_POINT ( 'NONE',  ( 23.48147201540000140, -59.02987586149999544, 0.03822384682579999665 ) ) ;
#11922=ORIENTED_EDGE ( 'NONE', *, *, #13993, .F. ) ;
#11924=FACE_OUTER_BOUND ( 'NONE', #11066, .T. ) ;
#11925=CARTESIAN_POINT ( 'NONE',  ( 36.65772703477473016, -74.21743014740448530, -14.37316385845866407 ) ) ;
#11927=CARTESIAN_POINT ( 'NONE',  ( -12.16975423829999947, -18.50000000000000000, 18.10341905029999765 ) ) ;
#11928=CARTESIAN_POINT ( 'NONE',  ( 24.22382765300000074, -64.24504439390000243, 10.76339935689999905 ) ) ;
#11929=CARTESIAN_POINT ( 'NONE',  ( 8.005872823979998998, -35.01852739750000154, -21.16125435099999663 ) ) ;
#11931=DIRECTION ( 'NONE',  ( 1.000000000000000000, 0.000000000000000000, 0.000000000000000000 ) ) ;
#11933=CARTESIAN_POINT ( 'NONE',  ( -11.48552613400000055, -58.81334883509999401, -22.65395064680000203 ) ) ;
#11934=CARTESIAN_POINT ( 'NONE',  ( 24.89230495879999694, -66.03766500179999355, -10.10284571010000043 ) ) ;
#11935=DIRECTION ( 'NONE',  ( -0.9295286103719527793, 0.000000000000000000, -0.3687499999999814260 ) ) ;
#11938=VERTEX_POINT ( 'NONE', #21639 ) ;
#11939=CARTESIAN_POINT ( 'NONE',  ( -13.59612654140000032, -34.59960680470000227, 20.74868692960000160 ) ) ;
#11944=ADVANCED_FACE ( 'NONE', ( #26161 ), #3168, .T. ) ;
#11946=CARTESIAN_POINT ( 'NONE',  ( -10.46620651823172210, -19.48040574461845509, -20.79821394406996760 ) ) ;
#11949=DIRECTION ( 'NONE',  ( 1.000000000000000000, 0.000000000000000000, 0.000000000000000000 ) ) ;
#11951=CARTESIAN_POINT ( 'NONE',  ( -32.83566817450000030, -79.50000000000000000, -22.22906645670000003 ) ) ;
#11953=CARTESIAN_POINT ( 'NONE',  ( -15.78701020529999965, -72.82938648530000592, 23.94860758700000147 ) ) ;
#11955=ORIENTED_EDGE ( 'NONE', *, *, #899, .T. ) ;
#11956=CARTESIAN_POINT ( 'NONE',  ( -3.027554198780000316, -80.05649091640000847, 46.84443221839999438 ) ) ;
#11961=CARTESIAN_POINT ( 'NONE',  ( -19.13290195579999775, -39.36414254489999820, 12.40799806240000080 ) ) ;
#11963=CARTESIAN_POINT ( 'NONE',  ( 29.03740435909999817, -74.36193762290000109, -26.47099454660000362 ) ) ;
#11964=CARTESIAN_POINT ( 'NONE',  ( 23.97384489419999909, -61.60336911379999947, -9.719973047129998989 ) ) ;
#11966=CARTESIAN_POINT ( 'NONE',  ( 26.37457956329999931, -67.43115654220000010, 0.9352255399990000440 ) ) ;
#11968=CARTESIAN_POINT ( 'NONE',  ( -39.61603006850076980, -73.75061506112956522, -7.239953483554843139 ) ) ;
#11969=AXIS2_PLACEMENT_3D ( 'NONE', #24978, #5166, #9811 ) ;
#11972=DIRECTION ( 'NONE',  ( -0.4692400087391606633, 0.000000000000000000, 0.8830706733883038062 ) ) ;
#11978=CARTESIAN_POINT ( 'NONE',  ( -26.33972759919999973, -80.00000000000000000, -36.23922253580000330 ) ) ;
#11979=CARTESIAN_POINT ( 'NONE',  ( 3.459338121946999694E-15, -73.50000000000000000, -32.25000000000000000 ) ) ;
#11983=CARTESIAN_POINT ( 'NONE',  ( -40.70731707320000226, -74.50000000000000000, 7.215414233289999757 ) ) ;
#11985=CARTESIAN_POINT ( 'NONE',  ( 23.41763709020000306, -53.52700728319999968, -9.527480143570000948 ) ) ;
#11987=CARTESIAN_POINT ( 'NONE',  ( 40.75609756099999714, -80.00000000000000000, -7.713029007999999465 ) ) ;
#11989=CARTESIAN_POINT ( 'NONE',  ( -2.597379844570000262, -26.02764329549999900, -24.46103497820000072 ) ) ;
#11990=CARTESIAN_POINT ( 'NONE',  ( 0.000000000000000000, -82.25000000000000000, 0.000000000000000000 ) ) ;
#11991=CARTESIAN_POINT ( 'NONE',  ( -24.63993737860000266, -72.00000000000000000, 17.98210258840000009 ) ) ;
#11993=AXIS2_PLACEMENT_3D ( 'NONE', #26850, #11379, #4848 ) ;
#11995=CARTESIAN_POINT ( 'NONE',  ( -40.00000000000000000, -69.00000000000000000, 1.332267629549999902E-15 ) ) ;
#11997=EDGE_CURVE ( 'NONE', #11090, #20924, #13245, .T. ) ;
#11999=CARTESIAN_POINT ( 'NONE',  ( -22.22906645670000003, -74.50000000000000000, -32.83566817450000030 ) ) ;
#12003=CARTESIAN_POINT ( 'NONE',  ( 20.83696519829999971, -34.90595158679999344, -8.468982500269998326 ) ) ;
#12004=CARTESIAN_POINT ( 'NONE',  ( 11.19993727630000002, -57.47855601759999900, 20.50134766809999931 ) ) ;
#12008=FACE_OUTER_BOUND ( 'NONE', #12410, .T. ) ;
#12009=CARTESIAN_POINT ( 'NONE',  ( 8.881784197000000993E-16, -19.50000000000000000, 1.776356839399999922E-14 ) ) ;
#12011=EDGE_LOOP ( 'NONE', ( #4217, #27533, #5919, #25832, #8334 ) ) ;
#12016=CARTESIAN_POINT ( 'NONE',  ( -7.250116280630000354, -73.92445350479999888, 39.77266773049999671 ) ) ;
#12017=CARTESIAN_POINT ( 'NONE',  ( -43.75000000000000000, -84.50000000000000000, 0.000000000000000000 ) ) ;
#12018=CARTESIAN_POINT ( 'NONE',  ( -40.70731707320000226, -84.00000000000000000, 7.215414233289999757 ) ) ;
#12019=CARTESIAN_POINT ( 'NONE',  ( 25.22253955729999930, -73.21919417370000360, -29.84906188120000081 ) ) ;
#12024=CARTESIAN_POINT ( 'NONE',  ( -17.94180966909999597, -18.50000000000000000, 18.81731824139999887 ) ) ;
#12025=CARTESIAN_POINT ( 'NONE',  ( -36.59277592640000165, -79.50000000000000000, -27.40038777100000189 ) ) ;
#12026=FACE_OUTER_BOUND ( 'NONE', #25438, .T. ) ;
#12029=ORIENTED_EDGE ( 'NONE', *, *, #19729, .T. ) ;
#12031=EDGE_CURVE ( 'NONE', #13803, #20924, #17354, .T. ) ;
#12032=CARTESIAN_POINT ( 'NONE',  ( -1.981473925119999757, -57.45864736019999697, -23.83876518969999836 ) ) ;
#12037=ADVANCED_FACE ( 'NONE', ( #3948 ), #15914, .T. ) ;
#12041=CIRCLE ( 'NONE', #7883, 0.5000000000000004441 ) ;
#12042=ORIENTED_EDGE ( 'NONE', *, *, #19697, .F. ) ;
#12043=DIRECTION ( 'NONE',  ( 0.000000000000000000, -1.000000000000000000, 0.000000000000000000 ) ) ;
#12044=DIRECTION ( 'NONE',  ( -0.4692400087391606633, 0.000000000000000000, 0.8830706733883038062 ) ) ;
#12046=ORIENTED_EDGE ( 'NONE', *, *, #11788, .F. ) ;
#12048=CARTESIAN_POINT ( 'NONE',  ( -11.39749306474008783, -60.86470925568636403, 20.85929151947415505 ) ) ;
#12049=CARTESIAN_POINT ( 'NONE',  ( -14.50205784900000161, -80.23773587339999835, 36.47412430930000227 ) ) ;
#12050=CARTESIAN_POINT ( 'NONE',  ( 26.98670340789999855, -72.82938977469999031, -9.720255250690000182 ) ) ;
#12051=CARTESIAN_POINT ( 'NONE',  ( -1.372948704489999949, -68.20869413019998717, -26.54380258120000136 ) ) ;
#12052=CARTESIAN_POINT ( 'NONE',  ( -17.13033210379999716, -72.00000000000000000, 23.49748962769999849 ) ) ;
#12056=CARTESIAN_POINT ( 'NONE',  ( 24.62957909909999898, -63.53922775760000263, 0.3042768451749999770 ) ) ;
#12057=CARTESIAN_POINT ( 'NONE',  ( -20.13976432299999786, -61.97101110970000093, 13.88607754689999929 ) ) ;
#12058=ORIENTED_EDGE ( 'NONE', *, *, #21252, .T. ) ;
#12060=CARTESIAN_POINT ( 'NONE',  ( -1.024287211530000130, -18.85467989400000022, -21.87431971389999674 ) ) ;
#12062=ORIENTED_EDGE ( 'NONE', *, *, #8004, .F. ) ;
#12063=TOROIDAL_SURFACE ( 'NONE', #6965, 30.50381168839999901, 2.000000000000000000 ) ;
#12065=LINE ( 'NONE', #26305, #5330 ) ;
#12068=FACE_OUTER_BOUND ( 'NONE', #24153, .T. ) ;
#12071=EDGE_LOOP ( 'NONE', ( #2079, #13251, #25508, #26555 ) ) ;
#12074=CARTESIAN_POINT ( 'NONE',  ( 36.96401661549065665, -79.81539336509945315, -14.32979729325936979 ) ) ;
#12079=CARTESIAN_POINT ( 'NONE',  ( 47.05360719204802677, -74.23346858368026346, -1.678317851455894072 ) ) ;
#12081=CARTESIAN_POINT ( 'NONE',  ( -11.76056861240000018, -34.66497403020000689, 19.52111231130000135 ) ) ;
#12085=VECTOR ( 'NONE', #1948, 1000.000000000000000 ) ;
#12086=AXIS2_PLACEMENT_3D ( 'NONE', #9661, #14331, #25416 ) ;
#12087=ORIENTED_EDGE ( 'NONE', *, *, #16956, .F. ) ;
#12089=SPHERICAL_SURFACE ( 'NONE', #684, 2.000000000000000000 ) ;
#12091=CARTESIAN_POINT ( 'NONE',  ( 8.036479196959999201E-15, -79.00000000000000000, -43.75000000000000000 ) ) ;
#12093=CARTESIAN_POINT ( 'NONE',  ( -32.83566817450000030, -79.65853147379999655, -22.22906645670000003 ) ) ;
#12095=DIRECTION ( 'NONE',  ( 1.000000000000000000, 0.000000000000000000, 0.000000000000000000 ) ) ;
#12097=CARTESIAN_POINT ( 'NONE',  ( -1.461556060870000007, -80.00014850240000897, 47.15629441589999971 ) ) ;
#12098=CARTESIAN_POINT ( 'NONE',  ( -15.22757417880000119, -66.82180077600000345, 22.72230046389999814 ) ) ;
#12100=LINE ( 'NONE', #27985, #15041 ) ;
#12101=CARTESIAN_POINT ( 'NONE',  ( -19.29510002299999982, -26.05152176790000240, 14.13598958989999765 ) ) ;
#12103=CARTESIAN_POINT ( 'NONE',  ( 31.02678878629999559, -72.72326922419999562, -21.89553410619999951 ) ) ;
#12104=CARTESIAN_POINT ( 'NONE',  ( -16.27748161717928710, -72.55114741086336494, 23.56761092879465735 ) ) ;
#12105=CIRCLE ( 'NONE', #28376, 21.03431122519999974 ) ;
#12106=AXIS2_PLACEMENT_3D ( 'NONE', #12255, #1089, #9927 ) ;
#12109=ORIENTED_EDGE ( 'NONE', *, *, #20581, .T. ) ;
#12111=CARTESIAN_POINT ( 'NONE',  ( 19.64679318960000032, -35.95469792330000303, -9.266762188240001308 ) ) ;
#12117=DIRECTION ( 'NONE',  ( 0.000000000000000000, 1.000000000000000000, 0.000000000000000000 ) ) ;
#12118=CARTESIAN_POINT ( 'NONE',  ( 7.194012074090000652, -40.75181153199999784, -21.61346702620000215 ) ) ;
#12122=AXIS2_PLACEMENT_3D ( 'NONE', #6446, #26281, #6304 ) ;
#12123=CARTESIAN_POINT ( 'NONE',  ( -40.33192879147393484, -74.21175622409107575, 7.242418264996894450 ) ) ;
#12124=CIRCLE ( 'NONE', #5157, 2.000000494510000504 ) ;
#12129=CARTESIAN_POINT ( 'NONE',  ( 23.93312658989999875, -65.07443093669999712, -7.727579958389999781 ) ) ;
#12130=FACE_BOUND ( 'NONE', #19663, .T. ) ;
#12131=CARTESIAN_POINT ( 'NONE',  ( -1.237516097069999876, -26.09793778660000285, -22.31349595290000210 ) ) ;
#12133=CARTESIAN_POINT ( 'NONE',  ( -2.289506448460466359, -74.01267423981741445, 46.88251229324449554 ) ) ;
#12134=CARTESIAN_POINT ( 'NONE',  ( 20.59810750441412708, -36.05978015059736208, -9.165578419059432491 ) ) ;
#12135=CARTESIAN_POINT ( 'NONE',  ( 21.70991749090000056, -40.75155002489999845, -6.890073352940000007 ) ) ;
#12138=ORIENTED_EDGE ( 'NONE', *, *, #24879, .F. ) ;
#12143=CIRCLE ( 'NONE', #17723, 7.249999999999999112 ) ;
#12144=TOROIDAL_SURFACE ( 'NONE', #15359, 6.750000000000000000, 2.000000000000000000 ) ;
#12145=VECTOR ( 'NONE', #12287, 1000.000000000000000 ) ;
#12147=CARTESIAN_POINT ( 'NONE',  ( 19.44233901680000187, -34.85245972529999392, -8.988706454689999958 ) ) ;
#12149=AXIS2_PLACEMENT_3D ( 'NONE', #10276, #21514, #26321 ) ;
#12151=CARTESIAN_POINT ( 'NONE',  ( -40.00438978219865049, -74.28332971660954342, 7.315286554457401280 ) ) ;
#12154=ORIENTED_EDGE ( 'NONE', *, *, #2410, .T. ) ;
#12158=CARTESIAN_POINT ( 'NONE',  ( 9.476764215410000247, -84.00000000000000000, 38.08875739639999836 ) ) ;
#12161=EDGE_CURVE ( 'NONE', #26794, #12777, #21628, .T. ) ;
#12162=CARTESIAN_POINT ( 'NONE',  ( -11.57749895095710357, -19.46656749805027076, 19.05743507200596909 ) ) ;
#12163=CARTESIAN_POINT ( 'NONE',  ( -7.260189318799999292, -74.10695981599999982, 39.96660922950000128 ) ) ;
#12166=CARTESIAN_POINT ( 'NONE',  ( 27.75394116159999669, -74.50000000000000000, -27.75394116159999669 ) ) ;
#12171=CARTESIAN_POINT ( 'NONE',  ( 9.024081099289999131, -19.49999992740000110, -18.94592230980000380 ) ) ;
#12174=ORIENTED_EDGE ( 'NONE', *, *, #8900, .T. ) ;
#12175=DIRECTION ( 'NONE',  ( 0.000000000000000000, -1.000000000000000000, 0.000000000000000000 ) ) ;
#12176=ORIENTED_EDGE ( 'NONE', *, *, #25916, .T. ) ;
#12178=CARTESIAN_POINT ( 'NONE',  ( 38.08875739639999836, -82.25000000000000000, 9.476764215410000247 ) ) ;
#12180=CARTESIAN_POINT ( 'NONE',  ( 10.15270808350000031, -36.18298320499999932, -21.93668074720000050 ) ) ;
#12182=AXIS2_PLACEMENT_3D ( 'NONE', #15294, #1937, #13124 ) ;
#12183=DIRECTION ( 'NONE',  ( 1.000000000000000000, 0.000000000000000000, 0.000000000000000000 ) ) ;
#12185=ORIENTED_EDGE ( 'NONE', *, *, #10924, .F. ) ;
#12191=CARTESIAN_POINT ( 'NONE',  ( -14.66608910859999959, -79.49999990050001486, 36.47374631070000106 ) ) ;
#12192=ADVANCED_FACE ( 'NONE', ( #23732 ), #27832, .T. ) ;
#12196=FACE_OUTER_BOUND ( 'NONE', #20076, .T. ) ;
#12198=CARTESIAN_POINT ( 'NONE',  ( 25.71993452759999954, -61.59933877579999972, 1.389394059650000068 ) ) ;
#12199=CARTESIAN_POINT ( 'NONE',  ( -20.88544710529999904, -61.59957509759999539, 15.07454172879999987 ) ) ;
#12200=VECTOR ( 'NONE', #23253, 1000.000000000000000 ) ;
#12204=AXIS2_PLACEMENT_3D ( 'NONE', #23937, #3976, #26276 ) ;
#12205=CARTESIAN_POINT ( 'NONE',  ( -1.878544191320000278, -18.85622860559999836, -22.19735407900000013 ) ) ;
#12206=CARTESIAN_POINT ( 'NONE',  ( 36.75967600126188728, -74.56302832687016746, -14.65138518224945052 ) ) ;
#12207=VERTEX_POINT ( 'NONE', #19221 ) ;
#12209=CARTESIAN_POINT ( 'NONE',  ( 24.78974732560000405, -64.24504771300000527, -10.08508462690000052 ) ) ;
#12210=CARTESIAN_POINT ( 'NONE',  ( 8.986258419809999509, -35.50000000000000000, -19.49544308430000328 ) ) ;
#12211=CARTESIAN_POINT ( 'NONE',  ( 36.32249705850000510, -79.79205832529999043, -14.87545865919999954 ) ) ;
#12213=EDGE_LOOP ( 'NONE', ( #21708, #27086, #28595 ) ) ;
#12214=B_SPLINE_SURFACE_WITH_KNOTS ( 'NONE', 5, 5, ( 
 ( #17584, #6509, #15370, #22107, #15822, #15522 ),
 ( #9120, #4470, #22243, #2293, #20059, #8974 ),
 ( #18021, #6809, #24575, #26919, #24733, #22551 ),
 ( #1376, #14745, #8194, #16114, #18322, #12547 ),
 ( #7924, #8062, #7398, #16952, #20497, #2735 ),
 ( #28161, #5204, #16261, #17080, #13789, #27352 ) ),
 .UNSPECIFIED., .F., .F., .F.,
 ( 6, 6 ),
 ( 6, 6 ),
 ( 0.000000000000000000, 3.318582258109999739 ),
 ( 0.000000000000000000, 0.5000000000000000000 ),
 .UNSPECIFIED. ) ;
#12215=CARTESIAN_POINT ( 'NONE',  ( 37.11608278482759005, -79.94792962045367801, -14.06916263102740494 ) ) ;
#12216=DIRECTION ( 'NONE',  ( -0.3687499999999814260, 0.000000000000000000, 0.9295286103719527793 ) ) ;
#12217=CARTESIAN_POINT ( 'NONE',  ( -2.119605539977385877, -80.25103533751058649, 46.93499847706560502 ) ) ;
#12218=ORIENTED_EDGE ( 'NONE', *, *, #6039, .F. ) ;
#12222=CIRCLE ( 'NONE', #3404, 6.749999999999999112 ) ;
#12226=ORIENTED_EDGE ( 'NONE', *, *, #23115, .F. ) ;
#12228=CARTESIAN_POINT ( 'NONE',  ( 9.561259125210000320, -36.00000000000000000, -20.11250876450000291 ) ) ;
#12229=CARTESIAN_POINT ( 'NONE',  ( 40.30310653829999978, -74.34472676610000974, 7.255206491210000053 ) ) ;
#12231=CARTESIAN_POINT ( 'NONE',  ( 18.85230044170000241, -18.50000000000000000, -8.028472989549999994 ) ) ;
#12234=CARTESIAN_POINT ( 'NONE',  ( -32.60788492590000232, -79.95698119190001307, -21.93599790929999926 ) ) ;
#12236=FACE_OUTER_BOUND ( 'NONE', #17950, .T. ) ;
#12237=ORIENTED_EDGE ( 'NONE', *, *, #7227, .T. ) ;
#12240=CARTESIAN_POINT ( 'NONE',  ( 41.00000000000000000, -74.50000000000000000, 10.20110288159999890 ) ) ;
#12242=VERTEX_POINT ( 'NONE', #23186 ) ;
#12247=CARTESIAN_POINT ( 'NONE',  ( 31.55438929119999614, -73.56648946160001401, -21.86866566000000134 ) ) ;
#12248=CARTESIAN_POINT ( 'NONE',  ( -14.48353243600127449, -74.09718790024807333, 36.26064929535388615 ) ) ;
#12250=CARTESIAN_POINT ( 'NONE',  ( -10.61287167039999879, -19.46510050319999863, 19.30934957549999709 ) ) ;
#12251=DIRECTION ( 'NONE',  ( 0.000000000000000000, 1.000000000000000000, 0.000000000000000000 ) ) ;
#12252=EDGE_LOOP ( 'NONE', ( #6975, #1244, #16732, #27851 ) ) ;
#12253=CARTESIAN_POINT ( 'NONE',  ( 21.01622931789999882, -35.47958268320000030, -8.366917739139999810 ) ) ;
#12255=CARTESIAN_POINT ( 'NONE',  ( -13.66168260340000096, -72.00000000000000000, -27.27344781959999764 ) ) ;
#12256=ORIENTED_EDGE ( 'NONE', *, *, #538, .F. ) ;
#12258=DIRECTION ( 'NONE',  ( 0.000000000000000000, 1.000000000000000000, 0.000000000000000000 ) ) ;
#12260=CARTESIAN_POINT ( 'NONE',  ( 47.25000000000000000, -79.00000000000000000, -7.709388683000000122E-13 ) ) ;
#12262=B_SPLINE_CURVE_WITH_KNOTS ( 'NONE', 3,
 ( #6612, #22500, #2392, #20000, #2238, #6761, #11084, #6905, #13438, #15769, #9514, #15623 ),
 .UNSPECIFIED., .F., .F.,
 ( 4, 2, 2, 2, 2, 4 ),
 ( 0.000000000000000000, 0.2500000000000059952, 0.5000000000000119904, 0.6250000000000104361, 0.7500000000000088818, 1.000000000000000000 ),
 .UNSPECIFIED. ) ;
#12264=TOROIDAL_SURFACE ( 'NONE', #660, 3.750000000000000000, 1.000000000000000000 ) ;
#12270=CARTESIAN_POINT ( 'NONE',  ( 23.52622212079999997, -57.40875702419999982, -9.564509902230000193 ) ) ;
#12271=ORIENTED_EDGE ( 'NONE', *, *, #6717, .T. ) ;
#12272=CARTESIAN_POINT ( 'NONE',  ( -14.38874196869999977, -74.12911414260001663, 36.70801399449999991 ) ) ;
#12273=EDGE_CURVE ( 'NONE', #3056, #27225, #3505, .T. ) ;
#12274=CARTESIAN_POINT ( 'NONE',  ( -14.59919359709999931, -74.50000000000000000, 36.80099833719999936 ) ) ;
#12277=TOROIDAL_SURFACE ( 'NONE', #6690, 3.500000000000000000, 0.5000000000000000000 ) ;
#12278=CARTESIAN_POINT ( 'NONE',  ( 41.23922093270000033, -74.00000000000000000, -13.75000000000000000 ) ) ;
#12279=AXIS2_PLACEMENT_3D ( 'NONE', #6623, #4135, #4722 ) ;
#12280=FACE_OUTER_BOUND ( 'NONE', #20372, .T. ) ;
#12281=FACE_OUTER_BOUND ( 'NONE', #6510, .T. ) ;
#12282=CARTESIAN_POINT ( 'NONE',  ( -10.86152808080000121, -19.46485671829999831, -19.26947891709999894 ) ) ;
#12284=CARTESIAN_POINT ( 'NONE',  ( -32.83566817900000245, -74.50000000069999828, -22.22906645790000013 ) ) ;
#12287=DIRECTION ( 'NONE',  ( 0.000000000000000000, 1.000000000000000000, 0.000000000000000000 ) ) ;
#12288=CARTESIAN_POINT ( 'NONE',  ( 21.08831565240000216, -34.74142176009999616, -8.079293962379999527 ) ) ;
#12289=CARTESIAN_POINT ( 'NONE',  ( 7.249313954219629430, -73.91187068868498500, 39.89765284896063946 ) ) ;
#12290=CARTESIAN_POINT ( 'NONE',  ( -12.71547034009999955, -65.00127802399998700, 21.72228991030000245 ) ) ;
#12295=CARTESIAN_POINT ( 'NONE',  ( -32.20769385759999892, -80.50000045429999318, -22.43272066369999962 ) ) ;
#12297=VERTEX_POINT ( 'NONE', #12231 ) ;
#12298=DIRECTION ( 'NONE',  ( -0.9704142011833032377, 0.000000000000000000, 0.2414462220490753985 ) ) ;
#12299=EDGE_LOOP ( 'NONE', ( #12176, #9717, #209, #20264 ) ) ;
#12300=EDGE_CURVE ( 'NONE', #5390, #2868, #13279, .T. ) ;
#12301=EDGE_CURVE ( 'NONE', #16727, #24784, #5319, .T. ) ;
#12303=CARTESIAN_POINT ( 'NONE',  ( -7.222916535669999583, -73.70405155900000693, 39.27999006289999784 ) ) ;
#12305=FACE_OUTER_BOUND ( 'NONE', #6319, .T. ) ;
#12308=CARTESIAN_POINT ( 'NONE',  ( -22.62548402540000225, -71.48510949040000639, 17.99032368389999803 ) ) ;
#12309=AXIS2_PLACEMENT_3D ( 'NONE', #11750, #7402, #10121 ) ;
#12310=DIRECTION ( 'NONE',  ( 1.000000000000000000, 0.000000000000000000, 0.000000000000000000 ) ) ;
#12311=CARTESIAN_POINT ( 'NONE',  ( 9.006609686890000077, -25.56710209000000233, -19.14378067089999647 ) ) ;
#12312=DIRECTION ( 'NONE',  ( -0.8349149399068952482, 0.000000000000000000, -0.5503789995269311452 ) ) ;
#12313=CARTESIAN_POINT ( 'NONE',  ( 20.07635942769760717, -19.46686856774696750, 9.756771846234537193 ) ) ;
#12320=CARTESIAN_POINT ( 'NONE',  ( 9.382534041599999597, -37.36473931380000124, -22.70474454669999886 ) ) ;
#12323=CARTESIAN_POINT ( 'NONE',  ( 19.86393766627161384, -19.48166550808161190, -8.699994293302530934 ) ) ;
#12327=ORIENTED_EDGE ( 'NONE', *, *, #9782, .F. ) ;
#12329=CARTESIAN_POINT ( 'NONE',  ( 8.638917257509998393, -36.16233246459999862, -20.97577343430000241 ) ) ;
#12330=CARTESIAN_POINT ( 'NONE',  ( -14.93121080350000085, -79.49999975080000070, 36.29905574549999869 ) ) ;
#12333=VERTEX_POINT ( 'NONE', #26496 ) ;
#12336=CARTESIAN_POINT ( 'NONE',  ( -32.54749500401306506, -74.13779231108122758, -22.15949318078843433 ) ) ;
#12337=CARTESIAN_POINT ( 'NONE',  ( 36.29989756469999662, -74.04896632250000721, -14.30540807509999901 ) ) ;
#12339=CARTESIAN_POINT ( 'NONE',  ( 10.00000000000000000, -89.00000000000000000, 0.000000000000000000 ) ) ;
#12340=CARTESIAN_POINT ( 'NONE',  ( -2.954912485889999552, -18.62107711730000048, -23.35157406449999939 ) ) ;
#12341=CARTESIAN_POINT ( 'NONE',  ( 36.45653638919409190, -74.05039938899749075, -14.06393186641748549 ) ) ;
#12342=ORIENTED_EDGE ( 'NONE', *, *, #25122, .F. ) ;
#12346=CARTESIAN_POINT ( 'NONE',  ( 7.135467526410000261, -73.50000000000000000, 38.71641004229999794 ) ) ;
#12349=CARTESIAN_POINT ( 'NONE',  ( -3.016175157618312674, -80.46478795248187055, 46.60229631513919202 ) ) ;
#12351=EDGE_LOOP ( 'NONE', ( #11335, #1147, #8824, #12674 ) ) ;
#12353=CARTESIAN_POINT ( 'NONE',  ( 21.57230431649999858, -55.03616289790000593, 10.16045490650000005 ) ) ;
#12355=EDGE_CURVE ( 'NONE', #2148, #22592, #5086, .T. ) ;
#12360=CARTESIAN_POINT ( 'NONE',  ( 39.54203581910000054, -73.97629583779999507, 7.314380512899999687 ) ) ;
#12361=B_SPLINE_CURVE_WITH_KNOTS ( 'NONE', 3,
 ( #20009, #17835, #15479, #15632, #10948, #19858, #6462, #9078, #24390, #27021, #17981, #26873, #18125, #15928 ),
 .UNSPECIFIED., .F., .F.,
 ( 4, 2, 1, 1, 1, 1, 2, 2, 4 ),
 ( 0.000000000000000000, 0.2500000000000070499, 0.3750000000000102696, 0.4375000000000084377, 0.4687500000000041078, 0.4843750000000019429, 0.4921875000000042188, 0.5000000000000064393, 1.000000000000000000 ),
 .UNSPECIFIED. ) ;
#12362=FACE_OUTER_BOUND ( 'NONE', #16463, .T. ) ;
#12365=EDGE_LOOP ( 'NONE', ( #12372, #21497, #2228, #219, #4263 ) ) ;
#12370=CARTESIAN_POINT ( 'NONE',  ( -2.674853241030000038E-13, -79.50000000000000000, 47.25000000000000000 ) ) ;
#12371=CARTESIAN_POINT ( 'NONE',  ( 22.77479925683983453, -18.50000000000000000, 9.339609901686905857 ) ) ;
#12372=ORIENTED_EDGE ( 'NONE', *, *, #5502, .F. ) ;
#12374=DIRECTION ( 'NONE',  ( 0.000000000000000000, 1.000000000000000000, 0.000000000000000000 ) ) ;
#12376=CARTESIAN_POINT ( 'NONE',  ( 27.75394116159999669, -74.50000000000000000, -27.75394116159999669 ) ) ;
#12378=B_SPLINE_CURVE_WITH_KNOTS ( 'NONE', 3,
 ( #17659, #28432, #28576, #13267 ),
 .UNSPECIFIED., .F., .F.,
 ( 4, 4 ),
 ( 0.000000000000000000, 1.000000000000000000 ),
 .UNSPECIFIED. ) ;
#12379=DIRECTION ( 'NONE',  ( 0.000000000000000000, 1.000000000000000000, 0.000000000000000000 ) ) ;
#12380=EDGE_CURVE ( 'NONE', #25468, #25683, #24613, .T. ) ;
#12382=ORIENTED_EDGE ( 'NONE', *, *, #9937, .T. ) ;
#12383=CARTESIAN_POINT ( 'NONE',  ( 21.47202455769999929, -36.32770022289999901, -7.310015199259999541 ) ) ;
#12384=CARTESIAN_POINT ( 'NONE',  ( 21.48170913309999719, -36.74612371620000317, -7.403099323020000178 ) ) ;
#12386=ADVANCED_FACE ( 'NONE', ( #7686 ), #17174, .T. ) ;
#12387=EDGE_LOOP ( 'NONE', ( #7976, #5788, #117, #11313, #28149, #12838, #28375 ) ) ;
#12392=CARTESIAN_POINT ( 'NONE',  ( 7.810721577829999873, -36.56420440790000015, -21.46720264389999855 ) ) ;
#12394=EDGE_LOOP ( 'NONE', ( #7244, #19318, #25091, #18133, #18661 ) ) ;
#12399=CARTESIAN_POINT ( 'NONE',  ( 47.25000000000000000, -75.00000000000000000, -1.245115460929999944E-12 ) ) ;
#12400=CARTESIAN_POINT ( 'NONE',  ( -14.76023875769999982, -74.50000000000000000, 45.51464203040000456 ) ) ;
#12401=CARTESIAN_POINT ( 'NONE',  ( -14.65986943260000075, -74.43317772470001614, 36.47430876989999859 ) ) ;
#12402=CARTESIAN_POINT ( 'NONE',  ( -2.184883600050000041, -19.44981017030000103, -22.64094073680000108 ) ) ;
#12404=ORIENTED_EDGE ( 'NONE', *, *, #23716, .T. ) ;
#12406=CARTESIAN_POINT ( 'NONE',  ( 9.004237477329999351, -35.65077419509999146, -19.54737253879999770 ) ) ;
#12407=CARTESIAN_POINT ( 'NONE',  ( 9.970358942569999883, -64.36570081249999475, -24.55403841179999702 ) ) ;
#12409=CARTESIAN_POINT ( 'NONE',  ( 6.929578963970000061, -35.67530021650000549, -21.51138254459999999 ) ) ;
#12410=EDGE_LOOP ( 'NONE', ( #1783, #10672, #15965, #18325 ) ) ;
#12415=CARTESIAN_POINT ( 'NONE',  ( 7.872101281680000007, -35.50412903890000393, -21.29303334629999966 ) ) ;
#12425=SURFACE_STYLE_USAGE ( .BOTH. , #8340 ) ;
#12427=EDGE_LOOP ( 'NONE', ( #6274, #18370, #9888, #15289, #8841 ) ) ;
#12431=CARTESIAN_POINT ( 'NONE',  ( -11.36637761219085974, -19.46558541313919122, 19.07288134243155042 ) ) ;
#12434=TOROIDAL_SURFACE ( 'NONE', #3615, 3.500000000000000000, 0.5000000000000000000 ) ;
#12436=CARTESIAN_POINT ( 'NONE',  ( 26.54452309970000101, -74.08494070260000797, -28.96748645319999937 ) ) ;
#12437=CARTESIAN_POINT ( 'NONE',  ( -22.51355778779999994, -71.15590230399999427, 17.45830423950000210 ) ) ;
#12438=FACE_OUTER_BOUND ( 'NONE', #12365, .T. ) ;
#12439=CARTESIAN_POINT ( 'NONE',  ( -19.05610772012959586, -19.48585536715970790, 13.96205032450363070 ) ) ;
#12440=CARTESIAN_POINT ( 'NONE',  ( 7.745600378490000715, -35.22612198869999389, -21.28939742640000077 ) ) ;
#12443=VERTEX_POINT ( 'NONE', #2755 ) ;
#12444=ADVANCED_FACE ( 'NONE', ( #11611 ), #592, .T. ) ;
#12445=EDGE_CURVE ( 'NONE', #6367, #17644, #21812, .T. ) ;
#12446=ORIENTED_EDGE ( 'NONE', *, *, #11200, .F. ) ;
#12447=CARTESIAN_POINT ( 'NONE',  ( -2.349966181920000174, -58.68498324069999939, -24.40456951870000069 ) ) ;
#12449=CYLINDRICAL_SURFACE ( 'NONE', #28340, 7.250000000000004441 ) ;
#12450=CARTESIAN_POINT ( 'NONE',  ( 21.23424069599999697, -35.30313414209999934, -7.936589188299999265 ) ) ;
#12451=ADVANCED_FACE ( 'NONE', ( #12305 ), #25725, .T. ) ;
#12454=CARTESIAN_POINT ( 'NONE',  ( -7.600472224666014576, -74.00014642295832346, -38.79568063749085383 ) ) ;
#12455=ORIENTED_EDGE ( 'NONE', *, *, #27753, .F. ) ;
#12456=CARTESIAN_POINT ( 'NONE',  ( 7.356933064080000584, -36.56811125840000187, -21.47791245320000186 ) ) ;
#12457=CYLINDRICAL_SURFACE ( 'NONE', #1557, 4.750000000000001776 ) ;
#12458=CIRCLE ( 'NONE', #15755, 10.50000000000000000 ) ;
#12459=CARTESIAN_POINT ( 'NONE',  ( -14.65665294340000102, -79.49999999100000991, 36.94583912339999898 ) ) ;
#12460=CARTESIAN_POINT ( 'NONE',  ( -17.82598797839999705, -18.50000000000000000, 11.16764024010000078 ) ) ;
#12463=CARTESIAN_POINT ( 'NONE',  ( 23.42789392040000251, -57.47571038070000782, 0.04069498556230000119 ) ) ;
#12464=CARTESIAN_POINT ( 'NONE',  ( -20.24912682730000313, -60.33063645209999493, 14.55614817839999908 ) ) ;
#12465=EDGE_CURVE ( 'NONE', #17023, #23155, #4621, .T. ) ;
#12468=DIRECTION ( 'NONE',  ( -0.9704142011833034598, 0.000000000000000000, -0.2414462220490750932 ) ) ;
#12469=CARTESIAN_POINT ( 'NONE',  ( 7.734359568749999525, -19.46510050329999686, -20.63161913629999944 ) ) ;
#12470=CARTESIAN_POINT ( 'NONE',  ( -1.123994816189999746, -18.50000000000000000, -21.31890798069999704 ) ) ;
#12472=B_SPLINE_CURVE_WITH_KNOTS ( 'NONE', 5,
 ( #14104, #2749, #583, #27224, #11456, #27367, #16129, #7411, #5064 ),
 .UNSPECIFIED., .F., .F.,
 ( 6, 3, 6 ),
 ( -2.709627183969999908, -2.032180022599999969, 0.000000000000000000 ),
 .UNSPECIFIED. ) ;
#12474=CARTESIAN_POINT ( 'NONE',  ( -18.78219790299999659, -19.46510053389999939, 11.52011550950000007 ) ) ;
#12476=CARTESIAN_POINT ( 'NONE',  ( 36.44456167670000468, -80.16838065170000505, -14.57571988100000127 ) ) ;
#12477=ORIENTED_EDGE ( 'NONE', *, *, #3383, .F. ) ;
#12479=EDGE_CURVE ( 'NONE', #21398, #19169, #453, .T. ) ;
#12482=CARTESIAN_POINT ( 'NONE',  ( -0.8937627406131904984, -79.83893697280288393, 47.19469876916298290 ) ) ;
#12483=ORIENTED_EDGE ( 'NONE', *, *, #962, .T. ) ;
#12484=CARTESIAN_POINT ( 'NONE',  ( 46.35082477299641113, -73.60002620146318009, -3.497084493779065273 ) ) ;
#12487=CARTESIAN_POINT ( 'NONE',  ( 20.77029242319999724, -55.05312981980000586, 10.65636466579999997 ) ) ;
#12488=CARTESIAN_POINT ( 'NONE',  ( 20.33566493080000015, -36.00000000000000000, -9.885503730140001721 ) ) ;
#12489=CARTESIAN_POINT ( 'NONE',  ( -7.432602092569998931, -73.95640471630001400, -39.04179453189999549 ) ) ;
#12492=CARTESIAN_POINT ( 'NONE',  ( 19.55164490770000185, -35.69157978159999800, -9.020399939569999859 ) ) ;
#12499=CIRCLE ( 'NONE', #26018, 7.250000000000000000 ) ;
#12500=CYLINDRICAL_SURFACE ( 'NONE', #19951, 7.250000000000004441 ) ;
#12502=CARTESIAN_POINT ( 'NONE',  ( 2.798556025240000070E-15, -74.00000000000000000, 3.175502518160000051E-15 ) ) ;
#12505=CARTESIAN_POINT ( 'NONE',  ( -0.5335602090409999887, -52.63293862069999562, -23.18581005440000098 ) ) ;
#12508=CARTESIAN_POINT ( 'NONE',  ( -3.730706918080000545, -79.99999997399999074, 46.61318877480000111 ) ) ;
#12509=CARTESIAN_POINT ( 'NONE',  ( -2.619606055569999814, -19.50000000000000000, -24.29997775220000023 ) ) ;
#12512=FACE_OUTER_BOUND ( 'NONE', #288, .T. ) ;
#12514=CARTESIAN_POINT ( 'NONE',  ( 30.15764098150000194, -74.11221873130000404, -25.07651571669999768 ) ) ;
#12515=EDGE_CURVE ( 'NONE', #21652, #3233, #23196, .T. ) ;
#12517=TOROIDAL_SURFACE ( 'NONE', #11595, 38.75000000000000000, 0.5000000000000000000 ) ;
#12520=CARTESIAN_POINT ( 'NONE',  ( 19.55068593369999874, -35.72724450179999423, -9.038647877299998967 ) ) ;
#12521=VERTEX_POINT ( 'NONE', #1527 ) ;
#12522=CARTESIAN_POINT ( 'NONE',  ( 19.55285847160000046, -35.83289739509999805, -9.107180759300000261 ) ) ;
#12524=ORIENTED_EDGE ( 'NONE', *, *, #5885, .T. ) ;
#12529=CYLINDRICAL_SURFACE ( 'NONE', #16438, 2.000000000000001776 ) ;
#12531=ORIENTED_EDGE ( 'NONE', *, *, #24534, .T. ) ;
#12536=CARTESIAN_POINT ( 'NONE',  ( 18.88171271619999914, -18.50000000000000000, -8.341252404190001357 ) ) ;
#12537=CARTESIAN_POINT ( 'NONE',  ( -14.60455326470000159, -74.31496036839999419, 36.89972645289999775 ) ) ;
#12539=ORIENTED_EDGE ( 'NONE', *, *, #21552, .F. ) ;
#12541=ADVANCED_FACE ( 'NONE', ( #19148 ), #5875, .T. ) ;
#12543=CARTESIAN_POINT ( 'NONE',  ( 0.000000000000000000, -84.00000000000000000, 0.000000000000000000 ) ) ;
#12546=CARTESIAN_POINT ( 'NONE',  ( 9.605468207570000416, -64.60177787579999631, -24.16120251349999748 ) ) ;
#12547=CARTESIAN_POINT ( 'NONE',  ( -39.45579440579999897, -74.12477399269999978, -7.440489808749999767 ) ) ;
#12548=ADVANCED_FACE ( 'NONE', ( #28256 ), #9647, .F. ) ;
#12549=CARTESIAN_POINT ( 'NONE',  ( 20.49658111199999766, -57.47855574479999774, 11.20865868970000001 ) ) ;
#12551=ORIENTED_EDGE ( 'NONE', *, *, #3910, .F. ) ;
#12556=DIRECTION ( 'NONE',  ( -0.3687499999999814260, 0.000000000000000000, 0.9295286103719527793 ) ) ;
#12557=CARTESIAN_POINT ( 'NONE',  ( 24.05168182727625847, -63.71467881788436927, 10.72464045306219660 ) ) ;
#12558=DIRECTION ( 'NONE',  ( 0.000000000000000000, -1.000000000000000000, 0.000000000000000000 ) ) ;
#12560=CARTESIAN_POINT ( 'NONE',  ( 0.000000000000000000, -86.00000000000000000, 0.000000000000000000 ) ) ;
#12562=CIRCLE ( 'NONE', #1006, 7.249999999999999112 ) ;
#12563=TOROIDAL_SURFACE ( 'NONE', #22367, 6.750000000000000000, 0.5000000000000000000 ) ;
#12564=CARTESIAN_POINT ( 'NONE',  ( 21.21808873300000187, -34.59820414320000026, -7.670973475509999417 ) ) ;
#12569=ORIENTED_EDGE ( 'NONE', *, *, #4441, .T. ) ;
#12574=DIRECTION ( 'NONE',  ( 0.000000000000000000, 0.000000000000000000, -1.000000000000000000 ) ) ;
#12575=CARTESIAN_POINT ( 'NONE',  ( 27.75394116159999669, -74.50000000000000000, -27.75394116159999669 ) ) ;
#12578=DIRECTION ( 'NONE',  ( 0.000000000000000000, 1.000000000000000000, 0.000000000000000000 ) ) ;
#12579=CARTESIAN_POINT ( 'NONE',  ( -11.92913933939999893, -65.75576304719999143, -23.66118000710000047 ) ) ;
#12580=CARTESIAN_POINT ( 'NONE',  ( 7.049162148299999764, -36.56981899800000235, -21.51316774079999661 ) ) ;
#12581=CARTESIAN_POINT ( 'NONE',  ( -10.31531692359999930, -18.50000000000000000, 18.33249795759999756 ) ) ;
#12586=EDGE_CURVE ( 'NONE', #1954, #14463, #2704, .T. ) ;
#12587=AXIS2_PLACEMENT_3D ( 'NONE', #27164, #7202, #16068 ) ;
#12589=CARTESIAN_POINT ( 'NONE',  ( 22.27494768480000076, -37.97325501589999419, -9.063917176249999486 ) ) ;
#12590=CARTESIAN_POINT ( 'NONE',  ( -2.596377074909999916, -62.44588796569999545, -25.54838417140000217 ) ) ;
#12593=CARTESIAN_POINT ( 'NONE',  ( 19.65745263667615816, -19.48583448325832634, -8.821903065879004302 ) ) ;
#12600=AXIS2_PLACEMENT_3D ( 'NONE', #5289, #946, #5568 ) ;
#12603=CARTESIAN_POINT ( 'NONE',  ( -14.34007285459999892, -80.00000123130000418, 37.07570051250000631 ) ) ;
#12605=CARTESIAN_POINT ( 'NONE',  ( -22.22906645670000003, -74.50000000000000000, -32.83566817450000030 ) ) ;
#12606=EDGE_CURVE ( 'NONE', #27953, #20968, #24078, .T. ) ;
#12607=CARTESIAN_POINT ( 'NONE',  ( 22.14119312130000239, -18.50000000000000000, 8.928410838750000522 ) ) ;
#12608=CARTESIAN_POINT ( 'NONE',  ( -32.47338858185761268, -74.10435492515816236, -22.14149567788639317 ) ) ;
#12609=DIRECTION ( 'NONE',  ( 0.000000000000000000, -1.000000000000000000, 0.000000000000000000 ) ) ;
#12611=CARTESIAN_POINT ( 'NONE',  ( 24.78974732560000405, -64.24504771300000527, -10.08508462690000052 ) ) ;
#12616=ADVANCED_FACE ( 'NONE', ( #3214 ), #9887, .T. ) ;
#12619=CARTESIAN_POINT ( 'NONE',  ( -31.89935321680000158, -74.00000000000000000, -21.99985828019999801 ) ) ;
#12620=CARTESIAN_POINT ( 'NONE',  ( 36.39191644179999940, -79.45170616170001665, -14.80043607370000025 ) ) ;
#12622=TOROIDAL_SURFACE ( 'NONE', #5661, 3.500000000000000000, 0.5000000000000000000 ) ;
#12626=CARTESIAN_POINT ( 'NONE',  ( 46.01499598271041691, -73.50000000000001421, -4.057494375605252834 ) ) ;
#12628=CARTESIAN_POINT ( 'NONE',  ( 21.63571023749999966, -57.45864773929999814, 10.20337500120000129 ) ) ;
#12630=CARTESIAN_POINT ( 'NONE',  ( -7.268571389559999929, -74.08839659379999887, -39.96417052329999819 ) ) ;
#12631=VERTEX_POINT ( 'NONE', #14136 ) ;
#12632=DIRECTION ( 'NONE',  ( 0.5301416321220551175, 0.000000000000000000, 0.8479091047340886478 ) ) ;
#12636=AXIS2_PLACEMENT_3D ( 'NONE', #6106, #21994, #19236 ) ;
#12644=VERTEX_POINT ( 'NONE', #22892 ) ;
#12648=CARTESIAN_POINT ( 'NONE',  ( 34.06016921999999880, -74.00000000000000000, -13.75000000000000000 ) ) ;
#12654=AXIS2_PLACEMENT_3D ( 'NONE', #20406, #7302, #20996 ) ;
#12655=DIRECTION ( 'NONE',  ( 9.280770596480004008E-17, 0.000000000000000000, -1.000000000000000000 ) ) ;
#12656=TOROIDAL_SURFACE ( 'NONE', #26642, 6.750000000000000000, 0.5000000000000000000 ) ;
#12658=EDGE_CURVE ( 'NONE', #25468, #19780, #12902, .T. ) ;
#12659=LINE ( 'NONE', #1627, #4730 ) ;
#12660=CARTESIAN_POINT ( 'NONE',  ( 21.38475920739999836, -35.91217828539999601, -7.828362488440000710 ) ) ;
#12661=VERTEX_POINT ( 'NONE', #13984 ) ;
#12662=CARTESIAN_POINT ( 'NONE',  ( 21.49488803819999916, -36.89279931859999806, -7.765148297399999677 ) ) ;
#12663=CARTESIAN_POINT ( 'NONE',  ( 7.599202867396026129, -18.61794787490824277, -20.27108518235802137 ) ) ;
#12664=ORIENTED_EDGE ( 'NONE', *, *, #26640, .F. ) ;
#12666=B_SPLINE_SURFACE_WITH_KNOTS ( 'NONE', 5, 5, ( 
 ( #13763, #2705, #16230, #247, #18290, #27180 ),
 ( #11864, #2414, #11560, #6781, #4587, #5022 ),
 ( #25142, #16087, #22964, #13910, #20627, #14057 ),
 ( #9673, #5175, #15791, #3006, #20775, #13612 ),
 ( #26889, #22522, #831, #18584, #15643, #24701 ),
 ( #4735, #24547, #13462, #11267, #20176, #9090 ) ),
 .UNSPECIFIED., .F., .F., .F.,
 ( 6, 6 ),
 ( 6, 6 ),
 ( 9.718751496520001254, 14.66109853230000049 ),
 ( 0.000000000000000000, 2.000000000000000000 ),
 .UNSPECIFIED. ) ;
#12672=CARTESIAN_POINT ( 'NONE',  ( 8.563702697320000112, -53.27760474060000462, -22.19980545599999999 ) ) ;
#12674=ORIENTED_EDGE ( 'NONE', *, *, #11452, .F. ) ;
#12676=CARTESIAN_POINT ( 'NONE',  ( 22.30116796419999758, -27.06785567060000020, -0.1709765798629999944 ) ) ;
#12677=CARTESIAN_POINT ( 'NONE',  ( 22.98572682540000045, -65.40406720010000186, 11.05257029390000056 ) ) ;
#12679=ORIENTED_EDGE ( 'NONE', *, *, #1413, .F. ) ;
#12683=CARTESIAN_POINT ( 'NONE',  ( -14.18001136240000015, -74.03309514170000227, 36.27836971480000017 ) ) ;
#12686=ORIENTED_EDGE ( 'NONE', *, *, #18731, .F. ) ;
#12689=CARTESIAN_POINT ( 'NONE',  ( -13.18754275750000104, -69.02891040180000459, -23.50545369980000032 ) ) ;
#12690=CARTESIAN_POINT ( 'NONE',  ( 21.69654716690000029, -58.73757401350000151, 10.24315597560000057 ) ) ;
#12691=CARTESIAN_POINT ( 'NONE',  ( -11.58786380919999992, -27.06642317520000063, -19.05189997919999811 ) ) ;
#12699=CARTESIAN_POINT ( 'NONE',  ( 21.40257419309999776, -18.50000000000000000, 0.9664833869290000434 ) ) ;
#12701=VERTEX_POINT ( 'NONE', #23719 ) ;
#12707=VERTEX_POINT ( 'NONE', #10023 ) ;
#12712=ADVANCED_FACE ( 'NONE', ( #28224, #23305 ), #27819, .T. ) ;
#12720=CARTESIAN_POINT ( 'NONE',  ( -22.19764394599999946, -69.10489204579999978, 16.61088088690000220 ) ) ;
#12722=CARTESIAN_POINT ( 'NONE',  ( -19.55651890851374475, -19.49660179764862633, 14.34605571524100043 ) ) ;
#12724=CARTESIAN_POINT ( 'NONE',  ( 7.120076906740000489, -35.74888742009999731, -21.45961752960000268 ) ) ;
#12727=VERTEX_POINT ( 'NONE', #1311 ) ;
#12730=CARTESIAN_POINT ( 'NONE',  ( -0.8504652179830000103, -58.79428935229999098, -23.42987164899999897 ) ) ;
#12731=AXIS2_PLACEMENT_3D ( 'NONE', #15658, #20643, #20190 ) ;
#12732=CARTESIAN_POINT ( 'NONE',  ( 9.393614097370001303, -37.99999999279999230, -22.97877291159999658 ) ) ;
#12735=CARTESIAN_POINT ( 'NONE',  ( -19.54048411320001222, -52.63055504210016267, 12.61913916920000034 ) ) ;
#12736=EDGE_CURVE ( 'NONE', #21778, #6019, #18151, .T. ) ;
#12739=CARTESIAN_POINT ( 'NONE',  ( 10.20110288159999890, -82.25000000000000000, -41.00000000000000000 ) ) ;
#12742=DIRECTION ( 'NONE',  ( 1.000000000000000000, 0.000000000000000000, 0.000000000000000000 ) ) ;
#12745=CIRCLE ( 'NONE', #10882, 0.5000000000000012212 ) ;
#12746=CARTESIAN_POINT ( 'NONE',  ( -17.93028678539999987, -18.50000000000000000, 10.99759328500000066 ) ) ;
#12750=ORIENTED_EDGE ( 'NONE', *, *, #7964, .F. ) ;
#12753=CARTESIAN_POINT ( 'NONE',  ( -5.679770007689999289, -79.50000000000000000, 47.25000000000000000 ) ) ;
#12757=CARTESIAN_POINT ( 'NONE',  ( -32.63753603780000390, -74.26163306789999297, -22.10337284230000066 ) ) ;
#12758=CARTESIAN_POINT ( 'NONE',  ( 36.29172732829999859, -79.00000000000000000, -14.94947765220000058 ) ) ;
#12760=AXIS2_PLACEMENT_3D ( 'NONE', #25302, #16823, #7799 ) ;
#12763=CARTESIAN_POINT ( 'NONE',  ( -0.8970218170808564873, -79.84013848330904750, 47.19429349399515417 ) ) ;
#12765=EDGE_CURVE ( 'NONE', #22592, #20540, #423, .T. ) ;
#12766=CARTESIAN_POINT ( 'NONE',  ( -12.22902281399961844, -69.69726684069728151, -24.77074626774463084 ) ) ;
#12767=DIRECTION ( 'NONE',  ( 0.000000000000000000, -1.000000000000000000, 0.000000000000000000 ) ) ;
#12769=AXIS2_PLACEMENT_3D ( 'NONE', #13680, #18055, #5088 ) ;
#12770=CARTESIAN_POINT ( 'NONE',  ( 22.81627243510000014, -54.99674360790000094, 10.21013232080000144 ) ) ;
#12772=CARTESIAN_POINT ( 'NONE',  ( -7.367397733560000717, -74.05254684259999465, -39.49475000900000765 ) ) ;
#12775=DIRECTION ( 'NONE',  ( 1.000000000000000000, 0.000000000000000000, 0.000000000000000000 ) ) ;
#12776=EDGE_CURVE ( 'NONE', #10585, #8240, #11146, .T. ) ;
#12777=VERTEX_POINT ( 'NONE', #15091 ) ;
#12778=CARTESIAN_POINT ( 'NONE',  ( 9.136262649109999856, -36.24018116499999564, -21.32348944479999986 ) ) ;
#12780=CARTESIAN_POINT ( 'NONE',  ( -3.638844514300000110, -18.50000000000000000, -24.22839726010000305 ) ) ;
#12784=DIRECTION ( 'NONE',  ( 0.000000000000000000, -1.000000000000000000, 0.000000000000000000 ) ) ;
#12786=CARTESIAN_POINT ( 'NONE',  ( -0.8454043835150000241, -53.84414347720000649, -23.22093481959999650 ) ) ;
#12793=CARTESIAN_POINT ( 'NONE',  ( 20.58776654729999933, -18.50000000000000000, 8.497741595429999961 ) ) ;
#12795=CARTESIAN_POINT ( 'NONE',  ( 36.70830950850000107, -75.00000000000000000, -14.75000000000000000 ) ) ;
#12800=EDGE_LOOP ( 'NONE', ( #19278, #27959, #11361, #18929 ) ) ;
#12801=ADVANCED_FACE ( 'NONE', ( #13349 ), #8709, .T. ) ;
#12802=CARTESIAN_POINT ( 'NONE',  ( 21.02097499579999962, -36.24640870310000196, -8.676716518870000172 ) ) ;
#12803=CARTESIAN_POINT ( 'NONE',  ( 6.850353625200000351, -36.56979901409999911, -21.56931447779999900 ) ) ;
#12810=CARTESIAN_POINT ( 'NONE',  ( 19.43643804750000115, -34.66800313659999944, -8.988996126470000902 ) ) ;
#12811=CARTESIAN_POINT ( 'NONE',  ( -10.77422065139999852, -19.15825174789999963, -19.39513388339999622 ) ) ;
#12815=CARTESIAN_POINT ( 'NONE',  ( 25.32712246539999867, -57.40875703270000230, 1.379782582989999895 ) ) ;
#12816=CARTESIAN_POINT ( 'NONE',  ( 24.30013770089999880, -66.02175891730000501, 10.80690825860000004 ) ) ;
#12818=ORIENTED_EDGE ( 'NONE', *, *, #12658, .F. ) ;
#12820=CYLINDRICAL_SURFACE ( 'NONE', #8529, 0.5000000000000012212 ) ;
#12822=DIRECTION ( 'NONE',  ( 0.000000000000000000, -1.000000000000000000, 0.000000000000000000 ) ) ;
#12824=CARTESIAN_POINT ( 'NONE',  ( 28.63360536809999957, -72.82938840390001189, 1.697633657649999961 ) ) ;
#12826=CARTESIAN_POINT ( 'NONE',  ( 9.038647564319999717, -35.72724395809999720, -19.55068592700000352 ) ) ;
#12827=FACE_OUTER_BOUND ( 'NONE', #13178, .T. ) ;
#12828=FACE_OUTER_BOUND ( 'NONE', #11726, .T. ) ;
#12829=CARTESIAN_POINT ( 'NONE',  ( 22.43070387670000088, -60.15167146970000545, 10.24377596799999957 ) ) ;
#12835=CARTESIAN_POINT ( 'NONE',  ( -32.70331798974049775, -74.50000000070001249, -22.03951504806313011 ) ) ;
#12836=CARTESIAN_POINT ( 'NONE',  ( 24.22382764319999993, -64.24504439390000243, 10.76339940740000145 ) ) ;
#12837=DIRECTION ( 'NONE',  ( 0.2414462220490755373, 0.000000000000000000, 0.9704142011833032377 ) ) ;
#12838=ORIENTED_EDGE ( 'NONE', *, *, #23477, .F. ) ;
#12840=B_SPLINE_SURFACE_WITH_KNOTS ( 'NONE', 5, 5, ( 
 ( #2475, #22870, #4797, #6988, #26946, #9295 ),
 ( #22429, #15700, #20684, #20087, #25046, #15852 ),
 ( #20376, #6692, #151, #5079, #15554, #13369 ),
 ( #22722, #2760, #11773, #22579, #305, #24458 ),
 ( #13816, #22273, #17911, #26804, #27092, #11471 ),
 ( #8849, #17762, #9144, #26648, #6836, #20529 ),
 ( #4494, #18049, #11618, #445, #24606, #24761 ),
 ( #2911, #13674, #2622, #18197, #7133, #598 ),
 ( #16001, #24905, #4935, #9442, #18350, #27237 ) ),
 .UNSPECIFIED., .F., .F., .F.,
 ( 6, 3, 6 ),
 ( 6, 6 ),
 ( 0.2311830627119999815, 0.9730373362299999940, 1.893943578530000060 ),
 ( 0.000000000000000000, 0.5000000000000000000 ),
 .UNSPECIFIED. ) ;
#12842=DIRECTION ( 'NONE',  ( 1.000000000000000000, 0.000000000000000000, 0.000000000000000000 ) ) ;
#12845=ORIENTED_EDGE ( 'NONE', *, *, #25573, .F. ) ;
#12849=CARTESIAN_POINT ( 'NONE',  ( 21.82773932530000138, -18.50000000000000000, 1.697762045069999948 ) ) ;
#12850=CARTESIAN_POINT ( 'NONE',  ( -24.63993737860000266, -72.00000000000000000, 17.98210258840000009 ) ) ;
#12855=EDGE_CURVE ( 'NONE', #24745, #23918, #6040, .T. ) ;
#12857=CARTESIAN_POINT ( 'NONE',  ( -18.51066704717978695, -19.46987374639787305, 12.90209632547328944 ) ) ;
#12858=CARTESIAN_POINT ( 'NONE',  ( 7.355131038309999703, -34.88462684899999999, -21.34291130700000139 ) ) ;
#12860=EDGE_LOOP ( 'NONE', ( #21519, #23167, #5608, #20995 ) ) ;
#12861=CARTESIAN_POINT ( 'NONE',  ( 7.383548971359999769, -18.50000000000000000, -19.69582298410000121 ) ) ;
#12862=CARTESIAN_POINT ( 'NONE',  ( 22.92823879609999693, -37.07368284070000186, -9.571688886919998751 ) ) ;
#12864=AXIS2_PLACEMENT_3D ( 'NONE', #18044, #22717, #11168 ) ;
#12865=CARTESIAN_POINT ( 'NONE',  ( 7.151043167926666833, -36.56947960410957421, -21.49478374055488317 ) ) ;
#12867=CARTESIAN_POINT ( 'NONE',  ( -20.51033946140000097, -54.98594849529999351, 14.82152834640000094 ) ) ;
#12868=DIRECTION ( 'NONE',  ( 0.9952295494196654602, 0.000000000000000000, -0.09756097560976770278 ) ) ;
#12872=AXIS2_PLACEMENT_3D ( 'NONE', #25554, #3415, #21737 ) ;
#12875=DIRECTION ( 'NONE',  ( 0.4794255386042036160, 0.000000000000000000, 0.8775825618903723147 ) ) ;
#12878=CARTESIAN_POINT ( 'NONE',  ( 20.70007164369999941, -19.44981017030000103, 9.428305666440000010 ) ) ;
#12879=CARTESIAN_POINT ( 'NONE',  ( -22.21882404873914396, -74.32470999146529778, -32.79282312874325100 ) ) ;
#12880=AXIS2_PLACEMENT_3D ( 'NONE', #14925, #12183, #1562 ) ;
#12881=CARTESIAN_POINT ( 'NONE',  ( 21.64091288609999708, -18.86472494550000079, 9.360502753589999614 ) ) ;
#12882=CARTESIAN_POINT ( 'NONE',  ( -32.70912902188079130, -74.24831373276512636, -22.19863839555747020 ) ) ;
#12883=DIRECTION ( 'NONE',  ( 0.000000000000000000, -1.000000000000000000, 0.000000000000000000 ) ) ;
#12885=DIRECTION ( 'NONE',  ( 0.9704142011833032377, 0.000000000000000000, 0.2414462220490753985 ) ) ;
#12887=EDGE_CURVE ( 'NONE', #18987, #11754, #27372, .T. ) ;
#12888=CARTESIAN_POINT ( 'NONE',  ( -7.208022861691824268, -73.58162913641194791, 39.21655428041565727 ) ) ;
#12892=DIRECTION ( 'NONE',  ( -1.000000000000000000, 0.000000000000000000, 6.217248937900000596E-16 ) ) ;
#12894=CARTESIAN_POINT ( 'NONE',  ( -22.47178550313523360, -79.93075540391261313, -32.73115669477952849 ) ) ;
#12898=B_SPLINE_SURFACE_WITH_KNOTS ( 'NONE', 5, 5, ( 
 ( #12171, #7394, #9983, #5620, #9564, #16692 ),
 ( #27207, #27778, #9698, #7246, #712, #11888 ),
 ( #12311, #25454, #20941, #16411, #25318, #7693 ),
 ( #5201, #14084, #18463, #27349, #18612, #14236 ),
 ( #23404, #23264, #3306, #3170, #1000, #5047 ),
 ( #16258, #14373, #25168, #3036, #13936, #854 ) ),
 .UNSPECIFIED., .F., .F., .F.,
 ( 6, 6 ),
 ( 6, 6 ),
 ( 12.34870487170000075, 33.81329059570000339 ),
 ( 0.000000000000000000, 2.000000000000000000 ),
 .UNSPECIFIED. ) ;
#12899=CARTESIAN_POINT ( 'NONE',  ( 19.55285847160000046, -35.83289739509999805, -9.107180759300000261 ) ) ;
#12901=ORIENTED_EDGE ( 'NONE', *, *, #22380, .F. ) ;
#12902=CIRCLE ( 'NONE', #11025, 0.5000000000000004441 ) ;
#12904=AXIS2_PLACEMENT_3D ( 'NONE', #4354, #15108, #26065 ) ;
#12906=CARTESIAN_POINT ( 'NONE',  ( 20.42111665379999863, -55.05574748869999979, 11.17031783180000026 ) ) ;
#12907=CARTESIAN_POINT ( 'NONE',  ( 45.99664575370000108, -73.93831497249999529, -4.396813293179999249 ) ) ;
#12908=ORIENTED_EDGE ( 'NONE', *, *, #4859, .F. ) ;
#12910=CARTESIAN_POINT ( 'NONE',  ( 47.19280574540000117, -74.66665734379999719, -1.149945984370000174 ) ) ;
#12911=ORIENTED_EDGE ( 'NONE', *, *, #2888, .T. ) ;
#12913=CARTESIAN_POINT ( 'NONE',  ( -12.07243358760000085, -45.73899999920000425, -24.77970463289999969 ) ) ;
#12917=VERTEX_POINT ( 'NONE', #3587 ) ;
#12920=DIRECTION ( 'NONE',  ( 1.000000000000000000, 0.000000000000000000, 0.000000000000000000 ) ) ;
#12921=CARTESIAN_POINT ( 'NONE',  ( -2.363861431270000146, -52.59522851940000265, -24.20187825489999867 ) ) ;
#12923=CARTESIAN_POINT ( 'NONE',  ( -19.68803165839999991, -18.87168151170000030, 14.53288016459999987 ) ) ;
#12924=ORIENTED_EDGE ( 'NONE', *, *, #16848, .F. ) ;
#12928=VECTOR ( 'NONE', #5431, 1000.000000000000000 ) ;
#12930=CYLINDRICAL_SURFACE ( 'NONE', #3608, 3.749999999999996447 ) ;
#12932=DIRECTION ( 'NONE',  ( 1.000000000000000000, 0.000000000000000000, 0.000000000000000000 ) ) ;
#12936=DIRECTION ( 'NONE',  ( 1.000000000000000000, 0.000000000000000000, 0.000000000000000000 ) ) ;
#12937=CARTESIAN_POINT ( 'NONE',  ( -11.90992159600000200, -57.47815920179999694, -20.09952900869999937 ) ) ;
#12938=ORIENTED_EDGE ( 'NONE', *, *, #28312, .T. ) ;
#12941=CIRCLE ( 'NONE', #17661, 7.250000000000000000 ) ;
#12943=CARTESIAN_POINT ( 'NONE',  ( 19.87955124240000160, -35.87174558430000104, -9.133536657829999683 ) ) ;
#12944=CARTESIAN_POINT ( 'NONE',  ( 9.476764215410000247, -82.25000000000000000, -38.08875739639999836 ) ) ;
#12947=AXIS2_PLACEMENT_3D ( 'NONE', #16976, #10387, #8086 ) ;
#12948=VECTOR ( 'NONE', #14773, 1000.000000000000000 ) ;
#12949=CARTESIAN_POINT ( 'NONE',  ( -3.369214011477492665, -68.11464510236007186, -27.57567578509392803 ) ) ;
#12950=CARTESIAN_POINT ( 'NONE',  ( -0.5853762890571154731, -19.20927481204733311, -22.01698796243409717 ) ) ;
#12951=CARTESIAN_POINT ( 'NONE',  ( 9.024081099289999131, -19.49999992740000110, -18.94592230980000380 ) ) ;
#12952=LINE ( 'NONE', #27769, #12200 ) ;
#12953=DIRECTION ( 'NONE',  ( 0.09756097560976997873, 0.000000000000000000, 0.9952295494196653491 ) ) ;
#12954=CARTESIAN_POINT ( 'NONE',  ( -10.06158909070000007, -18.61865660339999806, -19.91781936479999970 ) ) ;
#12955=LINE ( 'NONE', #8731, #20913 ) ;
#12958=CARTESIAN_POINT ( 'NONE',  ( 22.82317425849999992, -42.27249569770000193, -0.5642684588070000506 ) ) ;
#12959=CARTESIAN_POINT ( 'NONE',  ( 25.04292896270000313, -70.80052042889998631, 11.98325363630000062 ) ) ;
#12962=EDGE_CURVE ( 'NONE', #13629, #9669, #8260, .T. ) ;
#12963=CARTESIAN_POINT ( 'NONE',  ( -2.453167969115414238, -64.58097188162675195, -25.72104633702097942 ) ) ;
#12965=CARTESIAN_POINT ( 'NONE',  ( 25.14694229440000228, -65.07443093669999712, -0.3759436444569999591 ) ) ;
#12966=EDGE_LOOP ( 'NONE', ( #17929, #25248, #28702, #17585 ) ) ;
#12967=EDGE_CURVE ( 'NONE', #15667, #27517, #16187, .T. ) ;
#12968=CARTESIAN_POINT ( 'NONE',  ( 36.82697890865670587, -80.36910032511354984, -13.57704402516810305 ) ) ;
#12969=B_SPLINE_CURVE_WITH_KNOTS ( 'NONE', 3,
 ( #1516, #25172, #10360, #7249, #569, #25703 ),
 .UNSPECIFIED., .F., .F.,
 ( 4, 2, 4 ),
 ( 0.000000000000000000, 0.5000000000000000000, 1.000000000000000000 ),
 .UNSPECIFIED. ) ;
#12970=AXIS2_PLACEMENT_3D ( 'NONE', #9335, #11661, #24945 ) ;
#12972=CARTESIAN_POINT ( 'NONE',  ( 7.733063023050000595, -63.62941396979999809, -23.24181039339999799 ) ) ;
#12974=EDGE_CURVE ( 'NONE', #12631, #27292, #1156, .T. ) ;
#12975=CARTESIAN_POINT ( 'NONE',  ( 21.83262230589999930, -60.24417646120000569, 10.33011226949999894 ) ) ;
#12976=CARTESIAN_POINT ( 'NONE',  ( 24.08167113289999861, -63.05444450430000813, -9.753780024779999280 ) ) ;
#12978=AXIS2_PLACEMENT_3D ( 'NONE', #3699, #12558, #14350 ) ;
#12989=ADVANCED_FACE ( 'NONE', ( #3455 ), #16408, .T. ) ;
#12990=DIRECTION ( 'NONE',  ( 0.000000000000000000, 1.000000000000000000, 0.000000000000000000 ) ) ;
#12993=CARTESIAN_POINT ( 'NONE',  ( 3.768036230260000150E-15, -69.00000000000000000, 40.00000000000000000 ) ) ;
#12995=ORIENTED_EDGE ( 'NONE', *, *, #25510, .F. ) ;
#12996=CARTESIAN_POINT ( 'NONE',  ( 25.26718046270000073, -45.73899999920000425, 6.129403842640000377 ) ) ;
#12999=AXIS2_PLACEMENT_3D ( 'NONE', #20036, #6083, #18002 ) ;
#13000=TOROIDAL_SURFACE ( 'NONE', #23710, 43.34897771020000334, 20.00000000000000000 ) ;
#13002=CARTESIAN_POINT ( 'NONE',  ( 21.88953683090000268, -18.85523522049999912, -0.4607248773119999585 ) ) ;
#13003=CARTESIAN_POINT ( 'NONE',  ( -38.65106240728522380, -73.99999920929936081, -7.498734568567304137 ) ) ;
#13004=CARTESIAN_POINT ( 'NONE',  ( 23.52622212079999997, -57.40875702419999982, -9.564509902230000193 ) ) ;
#13012=CARTESIAN_POINT ( 'NONE',  ( 7.548681495209999426, -35.51902686380000063, -21.37164025960000302 ) ) ;
#13013=CARTESIAN_POINT ( 'NONE',  ( 19.35265720810000190, -32.04884292379999522, -8.993109114790000191 ) ) ;
#13016=CARTESIAN_POINT ( 'NONE',  ( 8.201027188560001235, -18.50000000000000000, -19.45829122079999962 ) ) ;
#13017=CIRCLE ( 'NONE', #22840, 3.750000000000000000 ) ;
#13018=AXIS2_PLACEMENT_3D ( 'NONE', #28139, #17059, #25953 ) ;
#13020=CARTESIAN_POINT ( 'NONE',  ( -1.970171503600000040, -60.24417646110000391, -24.07266168299999975 ) ) ;
#13022=CARTESIAN_POINT ( 'NONE',  ( -20.30439858460000124, -57.41946977150000464, 14.68516942459999974 ) ) ;
#13023=DIRECTION ( 'NONE',  ( 0.000000000000000000, 1.000000000000000000, 0.000000000000000000 ) ) ;
#13024=EDGE_CURVE ( 'NONE', #5884, #19001, #1313, .T. ) ;
#13026=CARTESIAN_POINT ( 'NONE',  ( 21.21808932789999957, -34.59820509829999935, -7.670972970100000232 ) ) ;
#13027=CARTESIAN_POINT ( 'NONE',  ( 7.253641904899999382, -74.31847293630001161, -40.32207487370000365 ) ) ;
#13030=ORIENTED_EDGE ( 'NONE', *, *, #16045, .T. ) ;
#13031=CARTESIAN_POINT ( 'NONE',  ( -14.19188836390000041, -80.00000061209999558, 37.13021406550000592 ) ) ;
#13033=CARTESIAN_POINT ( 'NONE',  ( -9.483174519389997670, -18.50000000000000000, -21.05226109790000066 ) ) ;
#13034=EDGE_CURVE ( 'NONE', #19989, #24375, #25035, .T. ) ;
#13035=AXIS2_PLACEMENT_3D ( 'NONE', #6317, #28316, #21913 ) ;
#13036=CARTESIAN_POINT ( 'NONE',  ( 32.39999999999999858, -86.00000000000000000, 3.967724586379999025E-15 ) ) ;
#13039=CARTESIAN_POINT ( 'NONE',  ( 22.63564271879999978, -18.50000000000000000, 8.833840388520000531 ) ) ;
#13040=CARTESIAN_POINT ( 'NONE',  ( 19.97576656849999921, -74.00000000000000000, -19.97576656849999921 ) ) ;
#13043=B_SPLINE_CURVE_WITH_KNOTS ( 'NONE', 3,
 ( #28158, #27747, #23641, #10491, #14472, #21317, #18994, #19406, #28287, #19132, #8318, #7785, #27874, #16805, #26112, #14334, #12133, #21050, #25840 ),
 .UNSPECIFIED., .F., .F.,
 ( 4, 2, 2, 2, 1, 1, 1, 2, 2, 2, 4 ),
 ( 0.000000000000000000, 0.2499999999999667488, 0.3749999999999501510, 0.4374999999999416578, 0.4687499999999342193, 0.4843749999999327760, 0.4921874999999295563, 0.4960937499999287792, 0.4999999999999280575, 0.7499999999999641398, 1.000000000000000000 ),
 .UNSPECIFIED. ) ;
#13048=EDGE_LOOP ( 'NONE', ( #2946, #18081, #16889, #11906, #5704 ) ) ;
#13049=DIRECTION ( 'NONE',  ( 1.000000000000000000, 0.000000000000000000, 0.000000000000000000 ) ) ;
#13050=CARTESIAN_POINT ( 'NONE',  ( -32.19107628040000435, -74.02008960720000630, -22.07235371499999843 ) ) ;
#13052=CARTESIAN_POINT ( 'NONE',  ( 24.90033419343626875, -40.03422670538211747, 1.393580993394984757 ) ) ;
#13055=CIRCLE ( 'NONE', #12600, 38.75000000000000000 ) ;
#13056=EDGE_LOOP ( 'NONE', ( #18467, #285, #23703, #18045, #27639, #23913, #14763, #7286, #28799, #10880, #9455, #23946, #7774, #4131, #4350, #13060 ) ) ;
#13057=CIRCLE ( 'NONE', #26101, 3.749999999999996447 ) ;
#13060=ORIENTED_EDGE ( 'NONE', *, *, #20433, .T. ) ;
#13063=VERTEX_POINT ( 'NONE', #19874 ) ;
#13064=CARTESIAN_POINT ( 'NONE',  ( 45.84677419350000349, -80.50000000000000000, -4.286925650119999709 ) ) ;
#13065=CARTESIAN_POINT ( 'NONE',  ( -22.22906621679999972, -79.65851410119999798, -32.83566840089999772 ) ) ;
#13067=ORIENTED_EDGE ( 'NONE', *, *, #24061, .F. ) ;
#13069=EDGE_CURVE ( 'NONE', #14954, #2162, #19892, .T. ) ;
#13070=CARTESIAN_POINT ( 'NONE',  ( 0.000000000000000000, -57.47855601759999900, 0.000000000000000000 ) ) ;
#13071=CARTESIAN_POINT ( 'NONE',  ( -0.7584661595949999668, -18.50000000000000000, -21.02157855700000155 ) ) ;
#13073=EDGE_CURVE ( 'NONE', #5555, #25224, #14779, .T. ) ;
#13076=LINE ( 'NONE', #8697, #5505 ) ;
#13077=CARTESIAN_POINT ( 'NONE',  ( -1.156066514279999957, -56.26441942339999969, -23.35759358749999848 ) ) ;
#13079=CIRCLE ( 'NONE', #1943, 1.000000000000000888 ) ;
#13080=CARTESIAN_POINT ( 'NONE',  ( 11.21116711998534576, -72.35538559737412356, -26.93475422593673230 ) ) ;
#13081=CARTESIAN_POINT ( 'NONE',  ( -40.00000000000000000, -69.00000000000000000, 3.236300116779999679E-15 ) ) ;
#13087=CARTESIAN_POINT ( 'NONE',  ( 20.38105827579999740, -18.50000000000000000, 8.542818265839999370 ) ) ;
#13089=B_SPLINE_SURFACE_WITH_KNOTS ( 'NONE', 5, 5, ( 
 ( #20220, #9133, #10716, #12907, #2164, #26934 ),
 ( #6369, #15096, #19631, #11000, #15236, #24297 ),
 ( #8684, #17602, #4341, #8833, #15542, #24448 ),
 ( #2307, #11157, #20075, #24748, #16274, #13953 ),
 ( #4783, #18626, #7264, #13802, #25030, #5364 ),
 ( #15837, #22707, #434, #25188, #27079, #9282 ),
 ( #22568, #9578, #18182, #18480, #9428, #7121 ),
 ( #20670, #11605, #15985, #730, #20513, #22856 ),
 ( #18334, #24891, #4924, #13662, #2899, #2608 ) ),
 .UNSPECIFIED., .F., .F., .F.,
 ( 6, 3, 6 ),
 ( 6, 6 ),
 ( 4.259926120710000319, 7.604735995929999604, 9.437975975800000583 ),
 ( 0.000000000000000000, 0.5000000000000000000 ),
 .UNSPECIFIED. ) ;
#13091=DIRECTION ( 'NONE',  ( 0.000000000000000000, 1.000000000000000000, 0.000000000000000000 ) ) ;
#13094=ORIENTED_EDGE ( 'NONE', *, *, #15036, .T. ) ;
#13095=CARTESIAN_POINT ( 'NONE',  ( 28.66034821447630065, -72.31232981782518721, 2.687344020524678356 ) ) ;
#13102=CARTESIAN_POINT ( 'NONE',  ( -26.33972759919999973, -74.00000000000000000, -36.23922253580000330 ) ) ;
#13103=ORIENTED_EDGE ( 'NONE', *, *, #14473, .F. ) ;
#13110=EDGE_CURVE ( 'NONE', #5390, #7572, #16400, .T. ) ;
#13112=CARTESIAN_POINT ( 'NONE',  ( 24.71478468710000342, -57.43018267659999765, 1.313252578800000014 ) ) ;
#13113=CARTESIAN_POINT ( 'NONE',  ( -27.40038777100000189, -77.00000000000000000, -36.59277592640000165 ) ) ;
#13114=CARTESIAN_POINT ( 'NONE',  ( 39.27497438177074685, -73.60295742109256878, 7.213678002735273154 ) ) ;
#13115=VERTEX_POINT ( 'NONE', #24706 ) ;
#13118=CARTESIAN_POINT ( 'NONE',  ( 41.00000000000000000, -74.00000000000000000, -10.20110288159999890 ) ) ;
#13120=CARTESIAN_POINT ( 'NONE',  ( 28.25592597320000010, -71.94685997979999570, 1.272191253259999932 ) ) ;
#13123=DIRECTION ( 'NONE',  ( 1.000000000000000000, 0.000000000000000000, -1.734723475976805517E-15 ) ) ;
#13124=DIRECTION ( 'NONE',  ( 1.000000000000000000, 0.000000000000000000, 0.000000000000000000 ) ) ;
#13125=CARTESIAN_POINT ( 'NONE',  ( 20.87785960109999905, -60.34598855900000558, 11.06351907140000002 ) ) ;
#13126=AXIS2_PLACEMENT_3D ( 'NONE', #21825, #1321, #12775 ) ;
#13129=VERTEX_POINT ( 'NONE', #13466 ) ;
#13130=CARTESIAN_POINT ( 'NONE',  ( -2.619606055569999814, -19.50000000000000000, -24.29997775220000023 ) ) ;
#13132=ADVANCED_FACE ( 'NONE', ( #9677 ), #17119, .F. ) ;
#13134=ORIENTED_EDGE ( 'NONE', *, *, #8119, .T. ) ;
#13138=CARTESIAN_POINT ( 'NONE',  ( 20.63024960799999974, -19.43020100670000261, -7.734540904970000241 ) ) ;
#13139=CARTESIAN_POINT ( 'NONE',  ( -7.135467526410000261, -73.65707963269998970, -38.71641004229999794 ) ) ;
#13141=ORIENTED_EDGE ( 'NONE', *, *, #26655, .F. ) ;
#13142=CARTESIAN_POINT ( 'NONE',  ( -3.653527372796985695, -80.06168500522677789, 46.47637749218215220 ) ) ;
#13146=ORIENTED_EDGE ( 'NONE', *, *, #12465, .T. ) ;
#13147=FACE_OUTER_BOUND ( 'NONE', #24412, .T. ) ;
#13149=DIRECTION ( 'NONE',  ( 0.09756097560976716154, 0.000000000000000000, 0.9952295494196655712 ) ) ;
#13152=CARTESIAN_POINT ( 'NONE',  ( 22.98887299579999777, -18.62004679909999894, 1.721454723069999915 ) ) ;
#13154=VERTEX_POINT ( 'NONE', #4740 ) ;
#13162=CARTESIAN_POINT ( 'NONE',  ( 0.000000000000000000, -65.07443093669999712, 0.000000000000000000 ) ) ;
#13164=DIRECTION ( 'NONE',  ( -0.1988145312159089739, -0.9099612708765829616, -0.3639275582888334415 ) ) ;
#13169=CARTESIAN_POINT ( 'NONE',  ( 22.97877291159999658, -37.99999999279999230, -9.393614097370001303 ) ) ;
#13170=AXIS2_PLACEMENT_3D ( 'NONE', #3093, #16611, #18381 ) ;
#13171=CARTESIAN_POINT ( 'NONE',  ( -13.13212274099999988, -63.41261178559999223, 21.16710223579999806 ) ) ;
#13174=CARTESIAN_POINT ( 'NONE',  ( -19.77751067240000182, -52.59522851940014476, 14.14810317790000838 ) ) ;
#13178=EDGE_LOOP ( 'NONE', ( #14507, #1894, #14082, #14024 ) ) ;
#13179=AXIS2_PLACEMENT_3D ( 'NONE', #18421, #18123, #15924 ) ;
#13180=CARTESIAN_POINT ( 'NONE',  ( 21.44183145790000111, -35.25283582229999979, -7.100559644140000515 ) ) ;
#13182=ORIENTED_EDGE ( 'NONE', *, *, #5597, .T. ) ;
#13183=ADVANCED_FACE ( 'NONE', ( #20180 ), #18015, .F. ) ;
#13186=CARTESIAN_POINT ( 'NONE',  ( -9.525302004199998507, -18.50000000000000000, -21.25953894639999930 ) ) ;
#13187=CIRCLE ( 'NONE', #26691, 3.499999999999999556 ) ;
#13189=CARTESIAN_POINT ( 'NONE',  ( 20.91081638819999711, -19.16559685929999901, 9.386484010540000256 ) ) ;
#13190=CARTESIAN_POINT ( 'NONE',  ( 10.31091299859999921, -69.35841635670000471, -25.71411929689999809 ) ) ;
#13192=ORIENTED_EDGE ( 'NONE', *, *, #5714, .T. ) ;
#13193=CARTESIAN_POINT ( 'NONE',  ( -12.84659744679999882, -72.82938648530000592, -25.64625568420000334 ) ) ;
#13194=CARTESIAN_POINT ( 'NONE',  ( 26.72438235069999735, -72.61900956739999913, -10.64645804510000104 ) ) ;
#13196=CARTESIAN_POINT ( 'NONE',  ( 22.82359378984540399, -61.65624515446846488, -7.265242739030600916 ) ) ;
#13197=ORIENTED_EDGE ( 'NONE', *, *, #27129, .F. ) ;
#13198=TOROIDAL_SURFACE ( 'NONE', #7655, 3.750000000000000000, 1.000000000000000000 ) ;
#13200=EDGE_CURVE ( 'NONE', #18713, #19738, #22432, .T. ) ;
#13203=VERTEX_POINT ( 'NONE', #4 ) ;
#13205=CARTESIAN_POINT ( 'NONE',  ( -40.65853658540000026, -84.50000000000000000, 6.717799458580000049 ) ) ;
#13210=ADVANCED_FACE ( 'NONE', ( #2477 ), #6416, .T. ) ;
#13211=DIRECTION ( 'NONE',  ( 1.000000000000000000, 0.000000000000000000, 0.000000000000000000 ) ) ;
#13213=ORIENTED_EDGE ( 'NONE', *, *, #3589, .T. ) ;
#13218=CARTESIAN_POINT ( 'NONE',  ( 19.43643804750000115, -34.66800313659999944, -8.988996126470000902 ) ) ;
#13221=CARTESIAN_POINT ( 'NONE',  ( -11.53802887301132607, -59.75213514187333175, -22.74397602207726266 ) ) ;
#13223=EDGE_LOOP ( 'NONE', ( #4836, #19018, #6654, #21111 ) ) ;
#13224=CARTESIAN_POINT ( 'NONE',  ( 36.31506118079999368, -74.00004962420000254, -14.00376701259999912 ) ) ;
#13226=LINE ( 'NONE', #19928, #22739 ) ;
#13228=CARTESIAN_POINT ( 'NONE',  ( 9.720255118479999012, -72.82938648530000592, -26.98670296669999757 ) ) ;
#13229=CARTESIAN_POINT ( 'NONE',  ( 21.47791241899999903, -36.56811125080000835, -7.356933755090000027 ) ) ;
#13230=ORIENTED_EDGE ( 'NONE', *, *, #25925, .T. ) ;
#13236=CARTESIAN_POINT ( 'NONE',  ( 21.42899162430000359, -18.50000000000000000, 8.464585110160001591 ) ) ;
#13242=FACE_OUTER_BOUND ( 'NONE', #16968, .T. ) ;
#13243=ORIENTED_EDGE ( 'NONE', *, *, #3255, .T. ) ;
#13245=B_SPLINE_CURVE_WITH_KNOTS ( 'NONE', 3,
 ( #2408, #11264, #11411, #11557, #20466, #9088 ),
 .UNSPECIFIED., .F., .F.,
 ( 4, 2, 4 ),
 ( 0.000000000000000000, 0.5000000000000000000, 1.000000000000000000 ),
 .UNSPECIFIED. ) ;
#13250=CARTESIAN_POINT ( 'NONE',  ( 30.91973185770000043, -72.00365067099998839, -22.05221014440000005 ) ) ;
#13251=ORIENTED_EDGE ( 'NONE', *, *, #9843, .T. ) ;
#13253=CARTESIAN_POINT ( 'NONE',  ( 9.885503723209998483, -36.00000000000000000, -20.33566493420000043 ) ) ;
#13255=CARTESIAN_POINT ( 'NONE',  ( -9.949002106569999171, -18.50000000000000000, -18.82416880939999970 ) ) ;
#13256=CARTESIAN_POINT ( 'NONE',  ( 47.20252187080182438, -79.30480005358090523, -1.049247932104649506 ) ) ;
#13257=ORIENTED_EDGE ( 'NONE', *, *, #2860, .F. ) ;
#13259=CARTESIAN_POINT ( 'NONE',  ( 24.24555580839999891, -27.00851495059999863, 1.474038313269999900 ) ) ;
#13260=LINE ( 'NONE', #13113, #8781 ) ;
#13261=CARTESIAN_POINT ( 'NONE',  ( -32.77174708219999388, -74.50000000000000000, -21.60034937629999874 ) ) ;
#13263=CARTESIAN_POINT ( 'NONE',  ( -1.084624312358362319, -65.04696244768176427, -25.11520602852569439 ) ) ;
#13265=CARTESIAN_POINT ( 'NONE',  ( 7.138278311610000593, -60.29602444460000044, -22.47789715730000282 ) ) ;
#13266=ORIENTED_EDGE ( 'NONE', *, *, #11083, .T. ) ;
#13267=CARTESIAN_POINT ( 'NONE',  ( 25.14694229440000228, -65.07443093669999712, -0.3759436444569999591 ) ) ;
#13269=CARTESIAN_POINT ( 'NONE',  ( 24.83705061268925007, -74.21720588690770626, -30.28267051683909372 ) ) ;
#13270=CARTESIAN_POINT ( 'NONE',  ( -12.19593855029999929, -68.24200910160000433, -24.12327046570000277 ) ) ;
#13271=EDGE_CURVE ( 'NONE', #22982, #10474, #22138, .T. ) ;
#13272=CARTESIAN_POINT ( 'NONE',  ( -11.53652411959999924, -49.87340317219999974, -20.08903528430000307 ) ) ;
#13275=AXIS2_PLACEMENT_3D ( 'NONE', #26832, #15728, #24641 ) ;
#13277=EDGE_CURVE ( 'NONE', #14660, #5636, #15231, .T. ) ;
#13278=ORIENTED_EDGE ( 'NONE', *, *, #17232, .F. ) ;
#13279=B_SPLINE_CURVE_WITH_KNOTS ( 'NONE', 5,
 ( #10168, #14828, #19087, #21143, #21549, #27973 ),
 .UNSPECIFIED., .F., .F.,
 ( 6, 6 ),
 ( -46.92787229070000166, 0.000000000000000000 ),
 .UNSPECIFIED. ) ;
#13283=ORIENTED_EDGE ( 'NONE', *, *, #21706, .F. ) ;
#13284=AXIS2_PLACEMENT_3D ( 'NONE', #21018, #25394, #20735 ) ;
#13286=CARTESIAN_POINT ( 'NONE',  ( 20.31493464609999933, -22.48307172219999828, -8.521724737190000454 ) ) ;
#13287=CARTESIAN_POINT ( 'NONE',  ( 22.20081257617079018, -19.46558063074879996, 0.3071883854471966213 ) ) ;
#13288=ORIENTED_EDGE ( 'NONE', *, *, #10404, .T. ) ;
#13289=DIRECTION ( 'NONE',  ( 1.000000000000000000, 0.000000000000000000, 0.000000000000000000 ) ) ;
#13292=CARTESIAN_POINT ( 'NONE',  ( 9.275138546780000937, -35.95833528409999502, -19.65753135889999825 ) ) ;
#13295=CARTESIAN_POINT ( 'NONE',  ( 21.89545778420000133, -18.85485920039999996, -0.1610960871889999813 ) ) ;
#13300=CARTESIAN_POINT ( 'NONE',  ( -13.08672874900000060, -19.48537664570000061, 19.65389566680000044 ) ) ;
#13302=CARTESIAN_POINT ( 'NONE',  ( -13.66168260340000096, -72.00000000000000000, -27.27344781959999764 ) ) ;
#13303=LINE ( 'NONE', #24250, #8752 ) ;
#13304=CARTESIAN_POINT ( 'NONE',  ( -12.31890027530000076, -66.79872818030000303, -23.02601073709999824 ) ) ;
#13307=ORIENTED_EDGE ( 'NONE', *, *, #16973, .F. ) ;
#13313=VERTEX_POINT ( 'NONE', #153 ) ;
#13314=CARTESIAN_POINT ( 'NONE',  ( -12.24789267649999935, -65.07443092999999124, 21.96586367309999943 ) ) ;
#13315=CARTESIAN_POINT ( 'NONE',  ( -1.878699226219999963, -64.89165510060000486, -25.21178815420000063 ) ) ;
#13317=CARTESIAN_POINT ( 'NONE',  ( -19.68721726160000074, -53.84414347720000649, 12.34260908240000099 ) ) ;
#13318=CARTESIAN_POINT ( 'NONE',  ( -10.93437413680000070, -19.50000027030000282, -21.85842452360000010 ) ) ;
#13321=CARTESIAN_POINT ( 'NONE',  ( 28.11272953839543121, -74.46129532805292683, -27.39515278475305493 ) ) ;
#13322=CARTESIAN_POINT ( 'NONE',  ( 7.135466578850000019, -73.50000064450000536, -38.71640869449999656 ) ) ;
#13324=CARTESIAN_POINT ( 'NONE',  ( -35.88566914520000495, -77.00000000000000000, -26.69328098980000163 ) ) ;
#13325=CARTESIAN_POINT ( 'NONE',  ( -40.65853658540000026, -84.50000000000000000, -6.717799458580000049 ) ) ;
#13326=CARTESIAN_POINT ( 'NONE',  ( 22.61819354930000259, -45.94038128989999592, 10.08865270770000144 ) ) ;
#13329=CARTESIAN_POINT ( 'NONE',  ( 20.51027266010000005, -57.91805314620000189, 11.21560917149999881 ) ) ;
#13332=VERTEX_POINT ( 'NONE', #15703 ) ;
#13333=FACE_OUTER_BOUND ( 'NONE', #10973, .T. ) ;
#13337=CARTESIAN_POINT ( 'NONE',  ( 22.77210041255538187, -61.43103207892549023, -7.246012015154788877 ) ) ;
#13338=ORIENTED_EDGE ( 'NONE', *, *, #15956, .T. ) ;
#13341=B_SPLINE_CURVE_WITH_KNOTS ( 'NONE', 5,
 ( #25982, #6298, #15163, #23800, #3835, #12699, #21613, #1666, #19418, #28299, #26708, #15308, #2531, #24225, #15908, #4853, #4410, #4698 ),
 .UNSPECIFIED., .F., .F.,
 ( 6, 3, 3, 3, 3, 6 ),
 ( 0.000000000000000000, 1.123597682109999996, 2.251105814029999763, 3.378920982540000395, 4.507089344450000645, 5.576980695509999642 ),
 .UNSPECIFIED. ) ;
#13342=PLANE ( 'NONE',  #4214 ) ;
#13343=CARTESIAN_POINT ( 'NONE',  ( -32.18652848360000007, -74.02659082439998883, -22.03329363239999950 ) ) ;
#13349=FACE_OUTER_BOUND ( 'NONE', #19882, .T. ) ;
#13350=ORIENTED_EDGE ( 'NONE', *, *, #2125, .T. ) ;
#13353=ORIENTED_EDGE ( 'NONE', *, *, #24715, .F. ) ;
#13357=VERTEX_POINT ( 'NONE', #24609 ) ;
#13359=CARTESIAN_POINT ( 'NONE',  ( 22.56940788859976266, -57.43018266628944701, 10.15711811299984646 ) ) ;
#13360=AXIS2_PLACEMENT_3D ( 'NONE', #26138, #28596, #26284 ) ;
#13362=CARTESIAN_POINT ( 'NONE',  ( 9.165580138570000202, -36.00000000019999646, -20.59810116059999885 ) ) ;
#13367=CARTESIAN_POINT ( 'NONE',  ( -4.439198032609999743E-16, -77.00000000000000000, 47.25000000000000000 ) ) ;
#13368=CARTESIAN_POINT ( 'NONE',  ( -39.23650411529999360, -73.50070240710000746, 7.229383731089999543 ) ) ;
#13369=CARTESIAN_POINT ( 'NONE',  ( -21.62384810780000066, -74.29049705580000307, -32.72083640759999668 ) ) ;
#13371=CIRCLE ( 'NONE', #22724, 7.750000000000000000 ) ;
#13372=CARTESIAN_POINT ( 'NONE',  ( -43.75000000000000000, -79.00000000000000000, 0.000000000000000000 ) ) ;
#13373=CARTESIAN_POINT ( 'NONE',  ( -7.627568735119999666, -74.00000000000000000, 38.62788659690000515 ) ) ;
#13374=CARTESIAN_POINT ( 'NONE',  ( -18.19213461030000190, -18.50000000000000000, 11.15819842919999871 ) ) ;
#13377=EDGE_CURVE ( 'NONE', #12777, #5069, #3206, .T. ) ;
#13378=CARTESIAN_POINT ( 'NONE',  ( 9.307782790770433579, -57.43039233035062097, -22.95932714880148851 ) ) ;
#13382=EDGE_CURVE ( 'NONE', #28507, #9115, #2624, .T. ) ;
#13385=CIRCLE ( 'NONE', #11536, 0.5000000000000004441 ) ;
#13387=ORIENTED_EDGE ( 'NONE', *, *, #25925, .F. ) ;
#13390=AXIS2_PLACEMENT_3D ( 'NONE', #3518, #12374, #21282 ) ;
#13391=CARTESIAN_POINT ( 'NONE',  ( -13.85849061559999917, -57.40875702409999803, 21.24403769210000092 ) ) ;
#13392=CARTESIAN_POINT ( 'NONE',  ( 5.258016244619999627E-13, -84.50000000000000000, -5.364597654989999396E-13 ) ) ;
#13397=CARTESIAN_POINT ( 'NONE',  ( -13.82310862920000005, -74.00000000000000000, 36.20061004769999613 ) ) ;
#13399=CARTESIAN_POINT ( 'NONE',  ( -7.325370793560000315, -72.00000000000000000, -24.94672208400000102 ) ) ;
#13402=CARTESIAN_POINT ( 'NONE',  ( 47.25000000000000000, -79.00000000000000000, -7.709388683000000122E-13 ) ) ;
#13404=VECTOR ( 'NONE', #17473, 1000.000000000000000 ) ;
#13405=DIRECTION ( 'NONE',  ( 0.000000000000000000, -1.000000000000000000, 0.000000000000000000 ) ) ;
#13406=CARTESIAN_POINT ( 'NONE',  ( -20.38196585287909457, -61.35680953179207364, 12.44223151297076058 ) ) ;
#13407=AXIS2_PLACEMENT_3D ( 'NONE', #19713, #15037, #17537 ) ;
#13409=VERTEX_POINT ( 'NONE', #9593 ) ;
#13410=EDGE_CURVE ( 'NONE', #8136, #15352, #28157, .T. ) ;
#13411=DIRECTION ( 'NONE',  ( 1.000000000000000000, 0.000000000000000000, 0.000000000000000000 ) ) ;
#13413=CARTESIAN_POINT ( 'NONE',  ( -22.65530694619999963, -72.00000000000000000, 18.22957389299999775 ) ) ;
#13415=CARTESIAN_POINT ( 'NONE',  ( 27.46886385830000066, -68.58900653949999082, 1.888124754229999924 ) ) ;
#13418=CARTESIAN_POINT ( 'NONE',  ( 28.97576656849999566, -38.00000000000000000, -19.97576656850000987 ) ) ;
#13420=CARTESIAN_POINT ( 'NONE',  ( 23.64759572430000034, -63.25393901619999326, -9.386700920010000004 ) ) ;
#13421=CARTESIAN_POINT ( 'NONE',  ( 0.000000000000000000, -82.25000000000000000, 40.00000000000000000 ) ) ;
#13422=DIRECTION ( 'NONE',  ( 0.09756097560976997873, 0.000000000000000000, -0.9952295494196653491 ) ) ;
#13423=CIRCLE ( 'NONE', #16706, 3.000000000000000000 ) ;
#13426=CARTESIAN_POINT ( 'NONE',  ( -2.619606461630943350, -19.18584080450747464, -24.29997790279570680 ) ) ;
#13429=CARTESIAN_POINT ( 'NONE',  ( 30.45033996220000105, -74.00000000000000000, 1.805359716810000181 ) ) ;
#13433=CARTESIAN_POINT ( 'NONE',  ( 22.62855517031298547, -19.47102808830224419, 0.9225138090183480077 ) ) ;
#13435=ORIENTED_EDGE ( 'NONE', *, *, #4032, .F. ) ;
#13436=FACE_OUTER_BOUND ( 'NONE', #8037, .T. ) ;
#13437=CARTESIAN_POINT ( 'NONE',  ( 8.295955541540001477, -37.60239178479999822, -21.68561411610000178 ) ) ;
#13438=CARTESIAN_POINT ( 'NONE',  ( 21.37812247595803328, -35.07876462143099161, -7.265514940539457456 ) ) ;
#13445=ORIENTED_EDGE ( 'NONE', *, *, #23090, .F. ) ;
#13446=ADVANCED_FACE ( 'NONE', ( #16145 ), #16203, .T. ) ;
#13448=CARTESIAN_POINT ( 'NONE',  ( -14.19924994259999984, -18.50000000000000000, 19.48093193789999944 ) ) ;
#13451=AXIS2_PLACEMENT_3D ( 'NONE', #7824, #10115, #5352 ) ;
#13452=CIRCLE ( 'NONE', #944, 1.000000000000000888 ) ;
#13453=DIRECTION ( 'NONE',  ( 0.9952295494196653491, 0.000000000000000000, 0.09756097560976997873 ) ) ;
#13454=CARTESIAN_POINT ( 'NONE',  ( -11.35954001540000036, -79.50000000000000000, 45.25000000000000000 ) ) ;
#13455=CARTESIAN_POINT ( 'NONE',  ( -9.476764215410000247, -84.00000000000000000, -38.08875739639999836 ) ) ;
#13460=CARTESIAN_POINT ( 'NONE',  ( 36.30177426670000074, -74.72020149879999451, -14.92507557220000081 ) ) ;
#13461=VERTEX_POINT ( 'NONE', #20531 ) ;
#13462=CARTESIAN_POINT ( 'NONE',  ( -13.22200285019999910, -64.89165763220000827, 21.54860465570000017 ) ) ;
#13464=CARTESIAN_POINT ( 'NONE',  ( 7.243395527602854322, -74.19510049697379372, 40.30949744634092013 ) ) ;
#13466=CARTESIAN_POINT ( 'NONE',  ( 38.71640881029999548, -73.50000064450000536, 7.135467304789999687 ) ) ;
#13467=CIRCLE ( 'NONE', #8346, 0.5000000000000004441 ) ;
#13469=CARTESIAN_POINT ( 'NONE',  ( -11.18016241693830182, -57.44036992075809422, -21.74842387285283962 ) ) ;
#13471=CARTESIAN_POINT ( 'NONE',  ( -7.472970580910000216, -74.00000000000000000, -38.65569705749999940 ) ) ;
#13472=CARTESIAN_POINT ( 'NONE',  ( 21.47791250119999873, -36.56811126780000620, -7.356933704980000321 ) ) ;
#13473=CARTESIAN_POINT ( 'NONE',  ( 7.562806955129999231, -74.00032110550000652, -39.03038279139999389 ) ) ;
#13474=ORIENTED_EDGE ( 'NONE', *, *, #21482, .T. ) ;
#13476=EDGE_CURVE ( 'NONE', #5258, #26105, #10078, .T. ) ;
#13478=CARTESIAN_POINT ( 'NONE',  ( 20.75931401429999923, -45.99312545570000310, 10.28958141490000067 ) ) ;
#13480=CARTESIAN_POINT ( 'NONE',  ( -21.60034937969999902, -74.50000000000000000, -32.77174707999999725 ) ) ;
#13482=CARTESIAN_POINT ( 'NONE',  ( 20.53475900819999822, -58.35721757130000498, 11.22800283159999957 ) ) ;
#13485=ORIENTED_EDGE ( 'NONE', *, *, #12967, .T. ) ;
#13486=DIRECTION ( 'NONE',  ( -0.04481497625361005599, -0.9975499440283644992, -0.05371896380604832683 ) ) ;
#13489=CARTESIAN_POINT ( 'NONE',  ( 20.42887670810370437, -19.46987374644096391, 9.579659739538350038 ) ) ;
#13496=DIRECTION ( 'NONE',  ( -0.3687499999999814260, 0.000000000000000000, 0.9295286103719527793 ) ) ;
#13497=CARTESIAN_POINT ( 'NONE',  ( 25.24946330670458394, -54.25046843273178609, 1.378801988918380239 ) ) ;
#13501=CARTESIAN_POINT ( 'NONE',  ( -22.91248086744062107, -71.02126462269738738, 15.84901304865810800 ) ) ;
#13505=AXIS2_PLACEMENT_3D ( 'NONE', #26813, #4653, #22440 ) ;
#13507=CARTESIAN_POINT ( 'NONE',  ( -22.56855420249999966, -80.00000000000000000, -32.68889834139999806 ) ) ;
#13508=TOROIDAL_SURFACE ( 'NONE', #537, 38.75000000000000000, 0.5000000000000000000 ) ;
#13510=TOROIDAL_SURFACE ( 'NONE', #4687, 6.750000000000000000, 0.5000000000000000000 ) ;
#13512=ADVANCED_FACE ( 'NONE', ( #7428 ), #20974, .F. ) ;
#13515=B_SPLINE_CURVE_WITH_KNOTS ( 'NONE', 5,
 ( #2229, #20145, #4551, #20441, #22636, #214 ),
 .UNSPECIFIED., .F., .F.,
 ( 6, 6 ),
 ( 0.000000000000000000, 1.000000000000000000 ),
 .UNSPECIFIED. ) ;
#13516=ORIENTED_EDGE ( 'NONE', *, *, #20815, .F. ) ;
#13519=CARTESIAN_POINT ( 'NONE',  ( -40.37845838710000379, -74.24284936579999794, 7.248115120149999591 ) ) ;
#13523=CARTESIAN_POINT ( 'NONE',  ( -7.588683564822256145, -74.00000000115923626, 38.71475194765147165 ) ) ;
#13524=CARTESIAN_POINT ( 'NONE',  ( 40.65508461000000295, -80.00000000000000000, -13.75000000000000000 ) ) ;
#13525=ORIENTED_EDGE ( 'NONE', *, *, #7861, .T. ) ;
#13530=CARTESIAN_POINT ( 'NONE',  ( 47.11548663039999951, -79.82827424500000291, -1.752954514250000040 ) ) ;
#13534=AXIS2_PLACEMENT_3D ( 'NONE', #10312, #7878, #14295 ) ;
#13537=CARTESIAN_POINT ( 'NONE',  ( 23.36166352360000076, -57.47815920179999694, -0.2645301549009999587 ) ) ;
#13539=CARTESIAN_POINT ( 'NONE',  ( -22.22906645670000003, -79.25000000000000000, -32.83566817450000030 ) ) ;
#13542=ORIENTED_EDGE ( 'NONE', *, *, #27055, .T. ) ;
#13543=CARTESIAN_POINT ( 'NONE',  ( -13.76297350900000005, -49.80571413040000550, 21.08331308489999856 ) ) ;
#13545=ORIENTED_EDGE ( 'NONE', *, *, #8641, .F. ) ;
#13550=DIRECTION ( 'NONE',  ( 0.000000000000000000, 1.000000000000000000, 0.000000000000000000 ) ) ;
#13553=CIRCLE ( 'NONE', #21925, 3.500000000000003109 ) ;
#13554=CARTESIAN_POINT ( 'NONE',  ( 21.70902145223586288, -37.93282145858484000, -8.317949937562373108 ) ) ;
#13555=EDGE_LOOP ( 'NONE', ( #12029, #3324, #394, #18777, #22569, #5639 ) ) ;
#13560=CARTESIAN_POINT ( 'NONE',  ( 39.83391879089067800, -73.87273571681690498, 7.248098695790405444 ) ) ;
#13565=ORIENTED_EDGE ( 'NONE', *, *, #1633, .T. ) ;
#13568=CARTESIAN_POINT ( 'NONE',  ( 21.45986210613797596, -74.01270519314725505, -32.43345270094494737 ) ) ;
#13570=CARTESIAN_POINT ( 'NONE',  ( -11.37720190070000115, -49.80573906490000269, -22.46074069029999976 ) ) ;
#13573=CARTESIAN_POINT ( 'NONE',  ( 40.70731707320000226, -77.00000000000000000, 7.215414233289999757 ) ) ;
#13574=CARTESIAN_POINT ( 'NONE',  ( -10.13149969890000079, -18.50000000000000000, 18.43352821810000108 ) ) ;
#13576=VECTOR ( 'NONE', #22921, 1000.000000000000000 ) ;
#13577=EDGE_LOOP ( 'NONE', ( #16992, #3340, #13638, #16698, #3846, #921 ) ) ;
#13585=CARTESIAN_POINT ( 'NONE',  ( 22.55098976337314909, -19.46994031921913049, 0.8437242863546875471 ) ) ;
#13587=VERTEX_POINT ( 'NONE', #18353 ) ;
#13588=CARTESIAN_POINT ( 'NONE',  ( 26.84105869354614526, -72.49728541232093448, -10.88571253161128105 ) ) ;
#13590=CARTESIAN_POINT ( 'NONE',  ( 8.520390455640001193, -37.01762350529999424, -21.57375892880000023 ) ) ;
#13591=CARTESIAN_POINT ( 'NONE',  ( 45.89652019322726062, -73.81415926414906892, -4.323399998322560833 ) ) ;
#13594=CIRCLE ( 'NONE', #17315, 3.499999999999999556 ) ;
#13595=CARTESIAN_POINT ( 'NONE',  ( 9.476764215410000247, -74.50000000000000000, -38.08875739639999836 ) ) ;
#13596=CARTESIAN_POINT ( 'NONE',  ( 21.49478374063930630, -36.56947960183979518, -7.151043167494730568 ) ) ;
#13597=CARTESIAN_POINT ( 'NONE',  ( 25.26718046270000073, -18.50000000000000000, 6.129403842640000377 ) ) ;
#13598=B_SPLINE_CURVE_WITH_KNOTS ( 'NONE', 5,
 ( #2076, #40, #21877, #10915, #19823, #3959 ),
 .UNSPECIFIED., .F., .F.,
 ( 6, 6 ),
 ( 0.000000000000000000, 1.000000000000000000 ),
 .UNSPECIFIED. ) ;
#13603=B_SPLINE_CURVE_WITH_KNOTS ( 'NONE', 5,
 ( #7798, #23383, #7672, #3425, #8204, #6010, #12290, #14889, #21199 ),
 .UNSPECIFIED., .F., .F.,
 ( 6, 3, 6 ),
 ( 0.000000000000000000, 0.5000000000000000000, 1.000000000000000000 ),
 .UNSPECIFIED. ) ;
#13604=CARTESIAN_POINT ( 'NONE',  ( 25.32712259480000228, -57.40875702469999453, 1.379782074460000230 ) ) ;
#13605=DIRECTION ( 'NONE',  ( 1.000000000000000000, 0.000000000000000000, 0.000000000000000000 ) ) ;
#13606=CARTESIAN_POINT ( 'NONE',  ( -36.59277592640000165, -77.00000000000000000, -25.98617420859999783 ) ) ;
#13612=CARTESIAN_POINT ( 'NONE',  ( -14.87113501819999861, -65.53648121479999133, 22.45123099050000093 ) ) ;
#13613=CARTESIAN_POINT ( 'NONE',  ( -14.25684790429999893, -62.95263723189999183, 21.84526217519999847 ) ) ;
#13614=DIRECTION ( 'NONE',  ( 0.000000000000000000, 1.000000000000000000, 0.000000000000000000 ) ) ;
#13617=CARTESIAN_POINT ( 'NONE',  ( 20.16453947749999998, -36.00000000000000000, -9.644867042430000481 ) ) ;
#13618=CIRCLE ( 'NONE', #6637, 30.50381168839999901 ) ;
#13620=ADVANCED_FACE ( 'NONE', ( #8385 ), #28213, .T. ) ;
#13622=ORIENTED_EDGE ( 'NONE', *, *, #28400, .T. ) ;
#13624=CARTESIAN_POINT ( 'NONE',  ( -7.215414233289999757, -74.50000000000000000, -40.70731707320000226 ) ) ;
#13625=CARTESIAN_POINT ( 'NONE',  ( 28.91153913726728675, -74.37196457031747343, -26.52194363930463794 ) ) ;
#13628=CARTESIAN_POINT ( 'NONE',  ( 23.07334373890000023, -54.17834560379999687, 10.34261593159999926 ) ) ;
#13629=VERTEX_POINT ( 'NONE', #10283 ) ;
#13632=DIRECTION ( 'NONE',  ( 0.000000000000000000, -1.000000000000000000, 0.000000000000000000 ) ) ;
#13635=CARTESIAN_POINT ( 'NONE',  ( 22.15526589779999966, -65.02054951249999704, 11.85001090629999965 ) ) ;
#13638=ORIENTED_EDGE ( 'NONE', *, *, #20675, .F. ) ;
#13639=CARTESIAN_POINT ( 'NONE',  ( -12.78246122589999878, -70.56976055389999658, -24.52593635099999858 ) ) ;
#13642=CIRCLE ( 'NONE', #1124, 1.000000000000000888 ) ;
#13644=CARTESIAN_POINT ( 'NONE',  ( 23.81686956487109086, -64.79566076651281037, -7.674173441228443693 ) ) ;
#13647=EDGE_LOOP ( 'NONE', ( #4185, #3549, #13353, #19820 ) ) ;
#13648=EDGE_CURVE ( 'NONE', #26062, #19169, #23317, .T. ) ;
#13650=CIRCLE ( 'NONE', #1137, 2.500000000000000444 ) ;
#13657=B_SPLINE_CURVE_WITH_KNOTS ( 'NONE', 5,
 ( #5427, #23207, #650, #27294, #18405, #7331 ),
 .UNSPECIFIED., .F., .F.,
 ( 6, 6 ),
 ( 0.000000000000000000, 1.000000000000000000 ),
 .UNSPECIFIED. ) ;
#13658=DIRECTION ( 'NONE',  ( 0.000000000000000000, 1.000000000000000000, 0.000000000000000000 ) ) ;
#13659=VERTEX_POINT ( 'NONE', #25895 ) ;
#13660=CARTESIAN_POINT ( 'NONE',  ( -22.62019343126265625, -69.58561462934873987, 15.11541909148706075 ) ) ;
#13662=CARTESIAN_POINT ( 'NONE',  ( 47.17354595309999610, -74.60192833800000756, -1.119582300150000043 ) ) ;
#13664=AXIS2_PLACEMENT_3D ( 'NONE', #8460, #28428, #6423 ) ;
#13665=CARTESIAN_POINT ( 'NONE',  ( -10.05832918090000128, -74.00000000000000000, 34.34024345419999946 ) ) ;
#13666=CARTESIAN_POINT ( 'NONE',  ( -22.71848792900000191, -80.00000000000000000, -32.61798286559999838 ) ) ;
#13669=DIRECTION ( 'NONE',  ( 1.000000000000000000, 0.000000000000000000, 0.000000000000000000 ) ) ;
#13673=CARTESIAN_POINT ( 'NONE',  ( -39.12193274490000050, -73.75841684550000821, 7.250133233359999707 ) ) ;
#13674=CARTESIAN_POINT ( 'NONE',  ( -22.01433816329999971, -74.00000000000000000, -32.02416862469999614 ) ) ;
#13677=CARTESIAN_POINT ( 'NONE',  ( -7.485351522714842609, -73.99989166819224806, 38.96151920400748025 ) ) ;
#13678=CARTESIAN_POINT ( 'NONE',  ( 21.42681242760168914, -35.72549454987603212, -7.289241608393363769 ) ) ;
#13680=CARTESIAN_POINT ( 'NONE',  ( 0.000000000000000000, -86.00000000000000000, 0.000000000000000000 ) ) ;
#13682=CARTESIAN_POINT ( 'NONE',  ( 8.113043114279999912, -34.60505749659999708, -21.05852214609999962 ) ) ;
#13684=EDGE_CURVE ( 'NONE', #14853, #18925, #12458, .T. ) ;
#13685=CARTESIAN_POINT ( 'NONE',  ( -11.07305194678827043, -18.50000000000000000, -24.81486620154639411 ) ) ;
#13686=ORIENTED_EDGE ( 'NONE', *, *, #19776, .T. ) ;
#13687=CARTESIAN_POINT ( 'NONE',  ( 21.50956136780000350, -52.61368720120000120, 10.11639787090000020 ) ) ;
#13690=EDGE_CURVE ( 'NONE', #16909, #12644, #8301, .T. ) ;
#13691=CARTESIAN_POINT ( 'NONE',  ( -12.66643311790000048, -65.04696659260000047, -21.71432957020000032 ) ) ;
#13692=CARTESIAN_POINT ( 'NONE',  ( 25.02058483049999538, -57.41946977210000114, 1.375913446200000001 ) ) ;
#13695=VERTEX_POINT ( 'NONE', #12339 ) ;
#13696=DIRECTION ( 'NONE',  ( 0.000000000000000000, -1.000000000000000000, 0.000000000000000000 ) ) ;
#13697=CARTESIAN_POINT ( 'NONE',  ( 46.76737938683341156, -73.86778755184377587, -2.601362616105526993 ) ) ;
#13698=ORIENTED_EDGE ( 'NONE', *, *, #21796, .T. ) ;
#13700=CARTESIAN_POINT ( 'NONE',  ( -11.18242929300000021, -57.47855601759999900, 20.51090108450000216 ) ) ;
#13702=ORIENTED_EDGE ( 'NONE', *, *, #27873, .T. ) ;
#13705=CARTESIAN_POINT ( 'NONE',  ( -41.00000000000000000, -84.00000000000000000, -10.20110288159999890 ) ) ;
#13706=CARTESIAN_POINT ( 'NONE',  ( 26.50442268124868050, -71.53529804145092896, -9.316922704210117701 ) ) ;
#13707=AXIS2_PLACEMENT_3D ( 'NONE', #15932, #9224, #22514 ) ;
#13709=FACE_OUTER_BOUND ( 'NONE', #25502, .T. ) ;
#13710=ORIENTED_EDGE ( 'NONE', *, *, #20397, .F. ) ;
#13718=CARTESIAN_POINT ( 'NONE',  ( -21.43329341219999762, -64.24504445130001784, 15.59675287610000005 ) ) ;
#13722=CARTESIAN_POINT ( 'NONE',  ( -18.72487404859999671, -26.08233090750000116, 13.26742744989999956 ) ) ;
#13723=CARTESIAN_POINT ( 'NONE',  ( 27.03609113194391256, -74.42256117523155012, -28.47179119120458424 ) ) ;
#13724=CARTESIAN_POINT ( 'NONE',  ( 32.34203265880000089, -73.93832878009999376, -20.34158615750000010 ) ) ;
#13725=CARTESIAN_POINT ( 'NONE',  ( -14.76920872520722128, -74.23817965565569921, 36.28536762717221364 ) ) ;
#13726=ADVANCED_FACE ( 'NONE', ( #27804 ), #17144, .F. ) ;
#13728=EDGE_CURVE ( 'NONE', #5438, #20928, #10604, .T. ) ;
#13729=ORIENTED_EDGE ( 'NONE', *, *, #806, .T. ) ;
#13730=CARTESIAN_POINT ( 'NONE',  ( -39.06010443616429484, -73.53996501803551666, -7.188997797805019907 ) ) ;
#13733=B_SPLINE_CURVE_WITH_KNOTS ( 'NONE', 3,
 ( #5631, #14095, #9571, #5491, #3451, #1280 ),
 .UNSPECIFIED., .F., .F.,
 ( 4, 2, 4 ),
 ( 0.000000000000000000, 0.5000000000000000000, 1.000000000000000000 ),
 .UNSPECIFIED. ) ;
#13734=DIRECTION ( 'NONE',  ( 0.000000000000000000, 1.000000000000000000, 0.000000000000000000 ) ) ;
#13738=CARTESIAN_POINT ( 'NONE',  ( 23.17742085089960113, -19.47933631450631253, 1.304785058156784361 ) ) ;
#13740=CARTESIAN_POINT ( 'NONE',  ( 26.85156072424344131, -72.47607639700331106, -10.93820933281734042 ) ) ;
#13742=CARTESIAN_POINT ( 'NONE',  ( 7.971459325760000603, -37.27103823680000261, -21.55676125340000127 ) ) ;
#13743=CARTESIAN_POINT ( 'NONE',  ( 8.594185256147103047, -19.47869450728761720, -20.00856785065116838 ) ) ;
#13744=ORIENTED_EDGE ( 'NONE', *, *, #22310, .T. ) ;
#13747=CARTESIAN_POINT ( 'NONE',  ( 24.39713797690000163, -19.18584095090000119, 1.459766401380000023 ) ) ;
#13749=CARTESIAN_POINT ( 'NONE',  ( -2.135291575822543475, -19.47314420526490863, -22.69925340028805039 ) ) ;
#13751=CARTESIAN_POINT ( 'NONE',  ( -0.8452062098759999254, -52.63280639819999607, -23.17863372589999926 ) ) ;
#13752=DIRECTION ( 'NONE',  ( 0.000000000000000000, 1.000000000000000000, 0.000000000000000000 ) ) ;
#13754=B_SPLINE_CURVE_WITH_KNOTS ( 'NONE', 3,
 ( #15931, #378, #11100, #24835, #2402, #8783, #26581, #24691, #9222, #24251, #20013, #20166, #13604 ),
 .UNSPECIFIED., .F., .F.,
 ( 4, 2, 2, 1, 2, 2, 4 ),
 ( 0.000000000000000000, 0.2499999999999875655, 0.3749999999999815703, 0.4374999999999798495, 0.4687499999999790168, 0.4999999999999781286, 1.000000000000000000 ),
 .UNSPECIFIED. ) ;
#13756=CARTESIAN_POINT ( 'NONE',  ( 37.60355029590000697, -84.50000000000000000, -9.356041104380000917 ) ) ;
#13759=ORIENTED_EDGE ( 'NONE', *, *, #8307, .F. ) ;
#13762=CARTESIAN_POINT ( 'NONE',  ( -14.55867152370000106, -64.24504444460001196, 22.15151623919999935 ) ) ;
#13763=CARTESIAN_POINT ( 'NONE',  ( -13.44405735660000012, -68.28990366489999531, 22.97003097380000014 ) ) ;
#13767=CARTESIAN_POINT ( 'NONE',  ( -3.666223272120000027E-16, -84.50000000000000000, -40.00000000000000000 ) ) ;
#13768=CARTESIAN_POINT ( 'NONE',  ( -11.25973246350476487, -41.21911678045049854, -22.28515149975225285 ) ) ;
#13770=DIRECTION ( 'NONE',  ( 1.000000000000000000, 0.000000000000000000, 0.000000000000000000 ) ) ;
#13779=CARTESIAN_POINT ( 'NONE',  ( -7.248542667678731455, -73.88534697526095840, -39.85457864233587344 ) ) ;
#13780=CARTESIAN_POINT ( 'NONE',  ( 20.05190523629999788, -18.61827554290000108, 9.243272875029999724 ) ) ;
#13781=CARTESIAN_POINT ( 'NONE',  ( -20.91226881559999740, -64.69849613010001121, 14.77252284299999907 ) ) ;
#13783=ORIENTED_EDGE ( 'NONE', *, *, #2237, .F. ) ;
#13784=CARTESIAN_POINT ( 'NONE',  ( -12.17507554820000060, -71.31774462289999406, -25.53716782429999910 ) ) ;
#13787=ADVANCED_FACE ( 'NONE', ( #6060 ), #23989, .F. ) ;
#13788=CARTESIAN_POINT ( 'NONE',  ( 20.16789755236859705, -19.46756325250261455, 9.702623992525639451 ) ) ;
#13789=CARTESIAN_POINT ( 'NONE',  ( -38.65569830309999588, -74.00000023179998720, -7.472969336320000266 ) ) ;
#13798=CARTESIAN_POINT ( 'NONE',  ( -19.88709748648987485, -26.11257320932467252, 14.48079129993961978 ) ) ;
#13800=CARTESIAN_POINT ( 'NONE',  ( -22.67424940895870478, -69.82955780735299811, 15.23442037431579976 ) ) ;
#13802=CARTESIAN_POINT ( 'NONE',  ( 46.87568470190000625, -74.15546349729999065, -2.521714412790000193 ) ) ;
#13803=VERTEX_POINT ( 'NONE', #15081 ) ;
#13804=CARTESIAN_POINT ( 'NONE',  ( 7.217717631489795060, -73.61799623139430082, -39.31656870534071402 ) ) ;
#13808=CARTESIAN_POINT ( 'NONE',  ( -2.555683107399999709, -71.82672919469999329, -28.11473569369999836 ) ) ;
#13809=EDGE_CURVE ( 'NONE', #11515, #11754, #8535, .T. ) ;
#13813=ADVANCED_FACE ( 'NONE', ( #20201 ), #4167, .F. ) ;
#13814=CARTESIAN_POINT ( 'NONE',  ( -10.50000000000000000, -89.50000000000000000, 4.573100142190000219E-16 ) ) ;
#13816=CARTESIAN_POINT ( 'NONE',  ( -22.14868796429999875, -74.09723562380000317, -32.50232833649999975 ) ) ;
#13821=CARTESIAN_POINT ( 'NONE',  ( -18.51733628490000072, -18.50000000000000000, 14.45311368080000136 ) ) ;
#13822=ORIENTED_EDGE ( 'NONE', *, *, #16045, .F. ) ;
#13826=CARTESIAN_POINT ( 'NONE',  ( 8.079305843170001111, -34.74137583460000656, -21.08830559229999935 ) ) ;
#13828=PLANE ( 'NONE',  #9498 ) ;
#13829=VERTEX_POINT ( 'NONE', #19614 ) ;
#13830=CARTESIAN_POINT ( 'NONE',  ( 47.11061145800000105, -79.77209722760001398, -1.777386438419999992 ) ) ;
#13832=B_SPLINE_SURFACE_WITH_KNOTS ( 'NONE', 5, 5, ( 
 ( #20669, #25334, #20811, #15984, #11604, #25029, #873, #22855, #8077 ),
 ( #18625, #2898, #728, #27520, #5879, #7567, #5363, #14247, #20959 ),
 ( #26163, #24109, #6188, #24259, #8515, #21930, #4295, #8362, #12589 ),
 ( #1692, #17417, #21780, #22079, #10674, #8227, #6033, #14919, #10960 ),
 ( #19869, #28619, #6478, #10530, #17701, #19446, #26592, #15058, #21500 ),
 ( #1979, #17121, #10397, #4144, #19590, #12862, #28475, #19316, #13169 ) ),
 .UNSPECIFIED., .F., .F., .F.,
 ( 6, 6 ),
 ( 6, 3, 6 ),
 ( 4.007746616509999527, 6.717368912360000444 ),
 ( 0.000000000000000000, 1.000000000000000000, 2.000000000000000000 ),
 .UNSPECIFIED. ) ;
#13834=CARTESIAN_POINT ( 'NONE',  ( -11.04119194200000109, -18.61783138060000198, 18.70101294130000014 ) ) ;
#13835=CARTESIAN_POINT ( 'NONE',  ( -11.81703488210000152, -60.57882006589999691, -20.52627317210000157 ) ) ;
#13836=CARTESIAN_POINT ( 'NONE',  ( 25.63123037620000133, -69.68000722649999545, -9.264901491119999832 ) ) ;
#13842=CARTESIAN_POINT ( 'NONE',  ( 30.97576656850000276, -72.00000000000000000, -19.97576656849999921 ) ) ;
#13843=CARTESIAN_POINT ( 'NONE',  ( -21.60034937969999902, -74.39508596250000494, -32.77174707999999725 ) ) ;
#13844=EDGE_LOOP ( 'NONE', ( #14491, #27807, #16581, #19392 ) ) ;
#13845=AXIS2_PLACEMENT_3D ( 'NONE', #22284, #15563, #11022 ) ;
#13846=CARTESIAN_POINT ( 'NONE',  ( -2.581268101460000075, -55.47051022630000006, -25.18513566209999865 ) ) ;
#13849=CARTESIAN_POINT ( 'NONE',  ( 9.341186407280000196E-15, -73.50000000000000000, 32.75000000000000000 ) ) ;
#13852=DIRECTION ( 'NONE',  ( 0.2414462220490760924, 0.000000000000000000, 0.9704142011833030157 ) ) ;
#13854=ADVANCED_FACE ( 'NONE', ( #15366 ), #27853, .T. ) ;
#13855=DIRECTION ( 'NONE',  ( 0.000000000000000000, 1.000000000000000000, 0.000000000000000000 ) ) ;
#13857=CARTESIAN_POINT ( 'NONE',  ( -32.75442352089999787, -74.37394555080000202, -21.60834384349999837 ) ) ;
#13860=CARTESIAN_POINT ( 'NONE',  ( 7.627568735119999666, -74.00000000000000000, 38.62788659690000515 ) ) ;
#13861=CARTESIAN_POINT ( 'NONE',  ( -22.07768936720000141, -67.34374581909999335, 16.43776412940000142 ) ) ;
#13866=CARTESIAN_POINT ( 'NONE',  ( -18.82092041760000001, -26.09894693429999890, 11.90111641600000070 ) ) ;
#13867=DIRECTION ( 'NONE',  ( 0.4692400087391608854, 0.000000000000000000, -0.8830706733883039172 ) ) ;
#13868=CARTESIAN_POINT ( 'NONE',  ( -20.56018235820000228, -57.40875686090000585, 14.85415984670000000 ) ) ;
#13869=CARTESIAN_POINT ( 'NONE',  ( 22.22481399220000142, -59.04179743959999627, -7.379008407440000639 ) ) ;
#13870=CARTESIAN_POINT ( 'NONE',  ( 26.64666883629999816, -68.06111992670000177, 1.045296570979999951 ) ) ;
#13873=ORIENTED_EDGE ( 'NONE', *, *, #3727, .F. ) ;
#13874=DIRECTION ( 'NONE',  ( 0.000000000000000000, -1.000000000000000000, 0.000000000000000000 ) ) ;
#13879=AXIS2_PLACEMENT_3D ( 'NONE', #1038, #20688, #23293 ) ;
#13880=CARTESIAN_POINT ( 'NONE',  ( -24.52910776410000082, -80.00000000000000000, -34.42860270069999729 ) ) ;
#13884=DIRECTION ( 'NONE',  ( 0.000000000000000000, 0.000000000000000000, 1.000000000000000000 ) ) ;
#13886=CARTESIAN_POINT ( 'NONE',  ( 9.334885652660000588, -35.98248194970000213, -19.73601135230000025 ) ) ;
#13888=ORIENTED_EDGE ( 'NONE', *, *, #17777, .F. ) ;
#13889=ADVANCED_FACE ( 'NONE', ( #13333 ), #922, .T. ) ;
#13893=FACE_OUTER_BOUND ( 'NONE', #24956, .T. ) ;
#13895=CARTESIAN_POINT ( 'NONE',  ( -2.528726852669999747, -39.31812514059999586, -24.13485223549999859 ) ) ;
#13899=CARTESIAN_POINT ( 'NONE',  ( 21.30736387581682934, -36.52594040275587872, -8.753883468101205878 ) ) ;
#13900=CARTESIAN_POINT ( 'NONE',  ( 22.06548297080000154, -49.09615641340000280, -8.529247663889998776 ) ) ;
#13901=DIRECTION ( 'NONE',  ( 0.9704142011833032377, 0.000000000000000000, -0.2414462220490753985 ) ) ;
#13904=CARTESIAN_POINT ( 'NONE',  ( 36.38830550880000203, -74.66455843740000375, -14.80879927640000027 ) ) ;
#13906=AXIS2_PLACEMENT_3D ( 'NONE', #4712, #223, #17973 ) ;
#13908=CARTESIAN_POINT ( 'NONE',  ( -22.36358135397400915, -79.84238795997771376, -32.77853236111499058 ) ) ;
#13910=CARTESIAN_POINT ( 'NONE',  ( -14.26285779270000020, -66.60919528889999697, 22.17889389219999785 ) ) ;
#13911=CARTESIAN_POINT ( 'NONE',  ( 19.49544348129999705, -35.50000000000000000, -8.986258391389998934 ) ) ;
#13912=CARTESIAN_POINT ( 'NONE',  ( -12.04650752959999949, -69.29982884310000202, -25.46956806489999892 ) ) ;
#13914=CARTESIAN_POINT ( 'NONE',  ( 27.11492913210000211, -72.00000000000000000, 10.50528373760000100 ) ) ;
#13915=CARTESIAN_POINT ( 'NONE',  ( 20.64008983129999919, -36.00000000000000000, -9.237424967780000884 ) ) ;
#13917=CARTESIAN_POINT ( 'NONE',  ( -11.43065410415306360, -54.25046843265613461, -22.55607764996867814 ) ) ;
#13920=CARTESIAN_POINT ( 'NONE',  ( -1.372953186662330349, -68.20869324698577429, -26.54380194214392219 ) ) ;
#13927=DIRECTION ( 'NONE',  ( 0.000000000000000000, 1.000000000000000000, 0.000000000000000000 ) ) ;
#13931=CARTESIAN_POINT ( 'NONE',  ( -14.44374894240000096, -74.20280742140000996, 36.65188832069999592 ) ) ;
#13933=CARTESIAN_POINT ( 'NONE',  ( -13.46935432499999941, -20.29228382570000022, 20.41725230879999842 ) ) ;
#13934=ORIENTED_EDGE ( 'NONE', *, *, #28769, .T. ) ;
#13935=CARTESIAN_POINT ( 'NONE',  ( -12.70614022820000066, -71.64735197429999403, -25.11726403489999981 ) ) ;
#13936=CARTESIAN_POINT ( 'NONE',  ( 8.113044424579999969, -34.60505785169999626, -21.05852071150000171 ) ) ;
#13943=EDGE_LOOP ( 'NONE', ( #14180, #9425, #17590, #22708 ) ) ;
#13944=CIRCLE ( 'NONE', #19980, 7.750000000000000000 ) ;
#13945=EDGE_CURVE ( 'NONE', #24813, #22412, #21546, .T. ) ;
#13946=CARTESIAN_POINT ( 'NONE',  ( -2.353367699040000094, -57.44036955189999816, -24.34033158609999958 ) ) ;
#13947=CARTESIAN_POINT ( 'NONE',  ( 9.452942635460001242, -37.37167648650000018, -22.96193664180000127 ) ) ;
#13950=ORIENTED_EDGE ( 'NONE', *, *, #11222, .T. ) ;
#13951=CARTESIAN_POINT ( 'NONE',  ( -22.50373292842316886, -69.08892850191131174, 14.88162393626444668 ) ) ;
#13953=CARTESIAN_POINT ( 'NONE',  ( 46.77849477899999897, -74.12949171449999142, -3.288587074160000068 ) ) ;
#13956=CARTESIAN_POINT ( 'NONE',  ( -11.41973371908083301, -61.05366698308790774, 20.89350501692665318 ) ) ;
#13958=CARTESIAN_POINT ( 'NONE',  ( -3.360703170379999438, -72.70510570390000282, -28.43098690960000141 ) ) ;
#13959=CARTESIAN_POINT ( 'NONE',  ( -14.97759602049999827, -68.79203770149999286, 22.77015088919999997 ) ) ;
#13960=ORIENTED_EDGE ( 'NONE', *, *, #19807, .T. ) ;
#13961=AXIS2_PLACEMENT_3D ( 'NONE', #4822, #24783, #4515 ) ;
#13963=CARTESIAN_POINT ( 'NONE',  ( 36.68836020269999665, -74.16367787109999199, -14.39348829000000052 ) ) ;
#13964=CARTESIAN_POINT ( 'NONE',  ( -12.09704001540000107, -74.00000000000000000, 47.10905722069999513 ) ) ;
#13965=CARTESIAN_POINT ( 'NONE',  ( 24.62807377229999872, -60.38561542509999924, 1.171175192380000230 ) ) ;
#13969=CARTESIAN_POINT ( 'NONE',  ( -7.435894661898926117, -73.99970680622588759, 39.09073924653432641 ) ) ;
#13971=ORIENTED_EDGE ( 'NONE', *, *, #21169, .T. ) ;
#13973=CARTESIAN_POINT ( 'NONE',  ( 21.36082767509999769, -61.85641277710000452, 10.97888673409999960 ) ) ;
#13976=FACE_OUTER_BOUND ( 'NONE', #25558, .T. ) ;
#13978=CARTESIAN_POINT ( 'NONE',  ( 47.11148591230000449, -79.71592019339999524, -1.801975019300000147 ) ) ;
#13980=CARTESIAN_POINT ( 'NONE',  ( -12.05127807179999877, -63.53922775760000263, -21.48197960690000130 ) ) ;
#13981=CARTESIAN_POINT ( 'NONE',  ( 37.17270558886492893, -79.97602054853541631, -13.97001007350288404 ) ) ;
#13982=CIRCLE ( 'NONE', #25171, 6.749999999999999112 ) ;
#13983=CARTESIAN_POINT ( 'NONE',  ( 46.25000000000000000, -75.00000000000000000, -13.75000000000000000 ) ) ;
#13984=CARTESIAN_POINT ( 'NONE',  ( 7.564829567879999012E-15, -69.50000000000000000, 47.25000000000000000 ) ) ;
#13991=CARTESIAN_POINT ( 'NONE',  ( 20.69873715099999956, -52.63055504209999924, 10.61298605969999898 ) ) ;
#13993=EDGE_CURVE ( 'NONE', #24483, #21652, #25999, .T. ) ;
#13994=EDGE_LOOP ( 'NONE', ( #24032, #26043, #25784, #17300, #6756 ) ) ;
#13996=EDGE_CURVE ( 'NONE', #26201, #20928, #13423, .T. ) ;
#14001=CARTESIAN_POINT ( 'NONE',  ( 47.01838349386816418, -79.64000543255396281, -2.294466949720601168 ) ) ;
#14002=ORIENTED_EDGE ( 'NONE', *, *, #16116, .T. ) ;
#14003=CARTESIAN_POINT ( 'NONE',  ( -32.56304129029999217, -80.37807044109999310, -21.91706417159999987 ) ) ;
#14007=DIRECTION ( 'NONE',  ( 0.9295286103719511139, 0.000000000000000000, 0.3687499999999862554 ) ) ;
#14013=CARTESIAN_POINT ( 'NONE',  ( -19.73589946059999889, -32.67314204020000545, 14.40166454639999927 ) ) ;
#14015=CARTESIAN_POINT ( 'NONE',  ( 20.84156035690000053, -36.00000000000000000, -10.47482617329999854 ) ) ;
#14016=CARTESIAN_POINT ( 'NONE',  ( 22.21260241310000083, -59.01992241779999659, -8.007694976899999872 ) ) ;
#14017=CARTESIAN_POINT ( 'NONE',  ( 26.10056038380000132, -66.79872818009998525, 0.8445247833500000301 ) ) ;
#14018=EDGE_CURVE ( 'NONE', #19383, #7537, #3850, .T. ) ;
#14020=DIRECTION ( 'NONE',  ( 0.000000000000000000, 1.000000000000000000, 0.000000000000000000 ) ) ;
#14021=FACE_BOUND ( 'NONE', #11302, .T. ) ;
#14022=CARTESIAN_POINT ( 'NONE',  ( 21.30736387649999841, -36.52594040320000346, -8.753883468490000652 ) ) ;
#14024=ORIENTED_EDGE ( 'NONE', *, *, #17528, .F. ) ;
#14026=CARTESIAN_POINT ( 'NONE',  ( 7.215414233289999757, -74.50000000000000000, 40.70731707320000226 ) ) ;
#14027=CARTESIAN_POINT ( 'NONE',  ( 46.45339896309999261, -74.00000000000000000, -4.166463576890000020 ) ) ;
#14028=CIRCLE ( 'NONE', #7973, 0.4999999999999982236 ) ;
#14029=ADVANCED_FACE ( 'NONE', ( #14083 ), #7104, .T. ) ;
#14032=DIRECTION ( 'NONE',  ( 0.000000000000000000, -1.000000000000000000, 0.000000000000000000 ) ) ;
#14034=B_SPLINE_CURVE_WITH_KNOTS ( 'NONE', 3,
 ( #18415, #4559, #365, #2542, #24825, #26722, #26866, #4862, #9070, #13743, #22643, #18266, #27013, #518, #7199, #27304, #2682, #20153, #22346 ),
 .UNSPECIFIED., .F., .F.,
 ( 4, 2, 2, 2, 1, 1, 1, 2, 2, 2, 4 ),
 ( 0.000000000000000000, 0.2499999999997740696, 0.3749999999996625477, 0.4374999999996090905, 0.4687499999995831668, 0.4843749999995707878, 0.4921874999995670130, 0.4960937499995651256, 0.4999999999995631272, 0.7499999999997815081, 1.000000000000000000 ),
 .UNSPECIFIED. ) ;
#14038=DIRECTION ( 'NONE',  ( 0.9295286103719527793, 0.000000000000000000, 0.3687499999999814260 ) ) ;
#14039=CARTESIAN_POINT ( 'NONE',  ( 23.99041810810000186, -19.49268907760000147, 1.535546174039999823 ) ) ;
#14041=ORIENTED_EDGE ( 'NONE', *, *, #19562, .T. ) ;
#14042=CARTESIAN_POINT ( 'NONE',  ( -2.204108355239595252, -19.47440675035694113, -22.78057140629209698 ) ) ;
#14044=CARTESIAN_POINT ( 'NONE',  ( -1.520194665700000058, -32.72716367869999488, -22.67437676309999972 ) ) ;
#14048=FACE_OUTER_BOUND ( 'NONE', #15832, .T. ) ;
#14049=CARTESIAN_POINT ( 'NONE',  ( 7.426814492070000107, -35.28814190290000141, -21.34788074219999743 ) ) ;
#14050=DIRECTION ( 'NONE',  ( 0.000000000000000000, 1.000000000000000000, 0.000000000000000000 ) ) ;
#14053=AXIS2_PLACEMENT_3D ( 'NONE', #15118, #10460, #27991 ) ;
#14056=EDGE_CURVE ( 'NONE', #22316, #24445, #6437, .T. ) ;
#14057=CARTESIAN_POINT ( 'NONE',  ( -15.04362262010000073, -66.18012799950000158, 22.59069390079999806 ) ) ;
#14058=CARTESIAN_POINT ( 'NONE',  ( 8.991798710090000313, -35.60470291170000223, -19.53731210289999964 ) ) ;
#14060=ADVANCED_FACE ( 'NONE', ( #24870 ), #24517, .T. ) ;
#14061=CARTESIAN_POINT ( 'NONE',  ( -2.567353809430000133, -52.57401960329944757, -24.80239345939998330 ) ) ;
#14063=CARTESIAN_POINT ( 'NONE',  ( -39.31219897219543924, -74.09468416701456306, 7.479537002224956765 ) ) ;
#14065=CIRCLE ( 'NONE', #15921, 3.499999999999999556 ) ;
#14069=CARTESIAN_POINT ( 'NONE',  ( 23.50753042992814557, -18.50000000000000000, 9.440918867846139761 ) ) ;
#14075=DIRECTION ( 'NONE',  ( 0.000000000000000000, -1.000000000000000000, 0.000000000000000000 ) ) ;
#14077=CARTESIAN_POINT ( 'NONE',  ( -7.243395527613476936, -74.19510049677808183, -40.30949744608958696 ) ) ;
#14078=CARTESIAN_POINT ( 'NONE',  ( -14.59815767989999991, -74.50000000000000000, 36.63377406709999917 ) ) ;
#14081=B_SPLINE_SURFACE_WITH_KNOTS ( 'NONE', 5, 5, ( 
 ( #13700, #20108, #24481, #9164, #176, #2056, #27118, #23, #13391 ),
 ( #18221, #4514, #10896, #19803, #28683, #2343, #9024, #17930, #13543 ),
 ( #22451, #2497, #24782, #11351, #21132, #22745, #18808, #2787, #14141 ),
 ( #5256, #23039, #3088, #12081, #25500, #2935, #10027, #25372, #11939 ),
 ( #1055, #5531, #27559, #25075, #23312, #7602, #23177, #7456, #20852 ),
 ( #25227, #14420, #27700, #912, #14281, #7738, #16166, #16605, #11644 ) ),
 .UNSPECIFIED., .F., .F., .F.,
 ( 6, 6 ),
 ( 6, 3, 6 ),
 ( 33.01978391549999969, 86.80576485550000143 ),
 ( 0.000000000000000000, 1.000000000000000000, 2.000000000000000000 ),
 .UNSPECIFIED. ) ;
#14082=ORIENTED_EDGE ( 'NONE', *, *, #7478, .F. ) ;
#14083=FACE_OUTER_BOUND ( 'NONE', #28407, .T. ) ;
#14084=CARTESIAN_POINT ( 'NONE',  ( 8.968815321630000170, -28.58309803750000100, -19.70170933860000062 ) ) ;
#14085=CARTESIAN_POINT ( 'NONE',  ( -0.8479692464762066395, -57.47815905588110041, -23.34776748300164684 ) ) ;
#14090=B_SPLINE_CURVE_WITH_KNOTS ( 'NONE', 5,
 ( #2269, #11116, #8948, #17857, #26755, #13469, #22375, #2422, #11277 ),
 .UNSPECIFIED., .F., .F.,
 ( 6, 3, 6 ),
 ( 0.000000000000000000, 0.5000000000000000000, 1.000000000000000000 ),
 .UNSPECIFIED. ) ;
#14091=ORIENTED_EDGE ( 'NONE', *, *, #700, .F. ) ;
#14092=TOROIDAL_SURFACE ( 'NONE', #8945, 3.750000000000000000, 1.000000000000000000 ) ;
#14094=B_SPLINE_CURVE_WITH_KNOTS ( 'NONE', 3,
 ( #17768, #11177, #26653, #6697, #2325, #15558, #24463, #22277 ),
 .UNSPECIFIED., .F., .F.,
 ( 4, 2, 2, 4 ),
 ( 0.000000000000000000, 0.2500000000000013323, 0.5000000000000026645, 1.000000000000000000 ),
 .UNSPECIFIED. ) ;
#14095=CARTESIAN_POINT ( 'NONE',  ( -14.14515361762423495, -80.00000000000660805, 37.00794155579307443 ) ) ;
#14097=ADVANCED_FACE ( 'NONE', ( #9847 ), #7552, .F. ) ;
#14101=AXIS2_PLACEMENT_3D ( 'NONE', #22286, #6848, #2331 ) ;
#14104=CARTESIAN_POINT ( 'NONE',  ( 9.885503723209998483, -36.00000000000000000, -20.33566493420000043 ) ) ;
#14105=ORIENTED_EDGE ( 'NONE', *, *, #13277, .F. ) ;
#14106=CARTESIAN_POINT ( 'NONE',  ( 7.240437622353804947, -74.25043946920976623, -40.38463872251576703 ) ) ;
#14107=CARTESIAN_POINT ( 'NONE',  ( 24.58030493329999899, -18.50000000000000000, 2.442848308399999890 ) ) ;
#14109=B_SPLINE_CURVE_WITH_KNOTS ( 'NONE', 5,
 ( #27449, #9931, #21301, #7494, #14318, #23214 ),
 .UNSPECIFIED., .F., .F.,
 ( 6, 6 ),
 ( 0.000000000000000000, 1.000000000000000000 ),
 .UNSPECIFIED. ) ;
#14110=CARTESIAN_POINT ( 'NONE',  ( -1.403101961229999972, -65.53445078080000030, -25.32578616130000171 ) ) ;
#14111=CIRCLE ( 'NONE', #17827, 0.5000000000000027756 ) ;
#14114=CARTESIAN_POINT ( 'NONE',  ( 36.26491344080000090, -73.99869055300000298, -14.02738897890000125 ) ) ;
#14116=CARTESIAN_POINT ( 'NONE',  ( 24.45008145339999928, -61.97075362790000241, 0.7927955552359999825 ) ) ;
#14119=VERTEX_POINT ( 'NONE', #3860 ) ;
#14121=CARTESIAN_POINT ( 'NONE',  ( -2.377347181619999805, -18.50000000000000000, -21.46086959390000004 ) ) ;
#14124=CARTESIAN_POINT ( 'NONE',  ( -11.35954001540000036, -80.00000000000000000, 45.25000000000000000 ) ) ;
#14125=CIRCLE ( 'NONE', #3438, 0.4999999999999982236 ) ;
#14126=CARTESIAN_POINT ( 'NONE',  ( 22.08519268120000234, -61.72813301749999937, 10.48040124129999917 ) ) ;
#14129=DIRECTION ( 'NONE',  ( 1.000000000000000000, 0.000000000000000000, 0.000000000000000000 ) ) ;
#14130=ORIENTED_EDGE ( 'NONE', *, *, #17372, .F. ) ;
#14131=DIRECTION ( 'NONE',  ( -5.551115123129999410E-17, 0.000000000000000000, -1.000000000000000000 ) ) ;
#14132=ADVANCED_FACE ( 'NONE', ( #25453 ), #28052, .T. ) ;
#14133=CARTESIAN_POINT ( 'NONE',  ( -11.22008280819999904, -57.43018266680000039, -22.06025754099999858 ) ) ;
#14134=AXIS2_PLACEMENT_3D ( 'NONE', #4163, #1436, #3744 ) ;
#14135=CYLINDRICAL_SURFACE ( 'NONE', #15382, 11.00000000000000000 ) ;
#14136=CARTESIAN_POINT ( 'NONE',  ( 21.34788034980000049, -35.28814072549999281, -7.426815654249999454 ) ) ;
#14138=LINE ( 'NONE', #5103, #1049 ) ;
#14141=CARTESIAN_POINT ( 'NONE',  ( -13.67553535689999933, -42.20265308159999762, 20.91818002200000137 ) ) ;
#14142=DIRECTION ( 'NONE',  ( 0.3388747807339289597, 0.000000000000000000, 0.9408314849018030168 ) ) ;
#14143=VERTEX_POINT ( 'NONE', #26002 ) ;
#14145=AXIS2_PLACEMENT_3D ( 'NONE', #14124, #27243, #22729 ) ;
#14146=ORIENTED_EDGE ( 'NONE', *, *, #5182, .F. ) ;
#14149=CARTESIAN_POINT ( 'NONE',  ( -10.45871993891135077, -19.47933382267855151, -20.72446925435193421 ) ) ;
#14150=CARTESIAN_POINT ( 'NONE',  ( -12.07243358760000085, -19.50000000000000000, -24.77970463289999969 ) ) ;
#14152=CARTESIAN_POINT ( 'NONE',  ( 0.000000000000000000, -84.00000000000000000, 0.000000000000000000 ) ) ;
#14153=ORIENTED_EDGE ( 'NONE', *, *, #19729, .F. ) ;
#14155=B_SPLINE_CURVE_WITH_KNOTS ( 'NONE', 3,
 ( #25162, #7239, #22831, #269, #7097, #24865, #27496, #14077, #16405, #9692, #9558, #7546, #5039, #4899, #27341, #705, #18457, #9111, #13779, #2435, #24721, #9258, #11580, #4605, #2874, #20335, #18157, #7386, #20795, #4758, #20488, #11732, #5193 ),
 .UNSPECIFIED., .F., .F.,
 ( 4, 2, 2, 1, 1, 1, 2, 2, 2, 1, 1, 1, 2, 2, 2, 1, 1, 1, 2, 2, 4 ),
 ( 0.000000000000000000, 0.1250000000000962286, 0.1875000000001503520, 0.2187500000001845191, 0.2343750000002016165, 0.2421875000002045586, 0.2460937500002118861, 0.2500000000002191580, 0.3750000000000335287, 0.4374999999999393263, 0.4687499999998910316, 0.4843749999998623323, 0.4921874999998526179, 0.4999999999998428479, 0.6249999999997827294, 0.6874999999997485345, 0.7187499999997233324, 0.7343749999997187805, 0.7421874999997200018, 0.7499999999997212230, 1.000000000000000000 ),
 .UNSPECIFIED. ) ;
#14157=EDGE_CURVE ( 'NONE', #20989, #4763, #17619, .T. ) ;
#14159=VERTEX_POINT ( 'NONE', #23542 ) ;
#14162=CARTESIAN_POINT ( 'NONE',  ( 22.58213832176329916, -18.62337006874614076, 9.587758685844438133 ) ) ;
#14166=CARTESIAN_POINT ( 'NONE',  ( -19.08606228369999869, -39.36011816909999794, 12.73950996719999829 ) ) ;
#14168=CARTESIAN_POINT ( 'NONE',  ( 30.51745573710000059, -72.51545259190000081, -23.74117753099999817 ) ) ;
#14170=CARTESIAN_POINT ( 'NONE',  ( 22.56729896340000252, -60.49415570080000037, -8.664781794339999621 ) ) ;
#14172=CARTESIAN_POINT ( 'NONE',  ( 25.99900580609999778, -64.47177033809998647, 1.411681635039999883 ) ) ;
#14173=CIRCLE ( 'NONE', #12279, 7.249999999999999112 ) ;
#14174=B_SPLINE_CURVE_WITH_KNOTS ( 'NONE', 3,
 ( #6449, #15315, #22055, #27009, #11244, #22340, #10938, #22496, #9066, #17969, #20445, #11393, #26863, #6903, #19844, #69, #2234, #13740, #22640, #13588, #15916, #15464, #19996, #515, #6758, #15621, #24521, #24821, #2679, #9362, #11837, #2978, #7196 ),
 .UNSPECIFIED., .F., .F.,
 ( 4, 2, 2, 1, 1, 1, 2, 2, 2, 2, 1, 2, 2, 2, 2, 1, 2, 2, 4 ),
 ( 0.000000000000000000, 0.1249999999998855915, 0.1874999999998287481, 0.2187499999998012978, 0.2343749999997877531, 0.2421874999997861155, 0.2460937499997827016, 0.2499999999997792877, 0.3749999999998528399, 0.4374999999998868128, 0.4687499999999028000, 0.4843749999999092948, 0.4999999999999157341, 0.6249999999999484857, 0.6874999999999675815, 0.7187499999999762412, 0.7343749999999791278, 0.7499999999999819034, 1.000000000000000000 ),
 .UNSPECIFIED. ) ;
#14175=DIRECTION ( 'NONE',  ( 0.000000000000000000, 1.000000000000000000, 0.000000000000000000 ) ) ;
#14177=CARTESIAN_POINT ( 'NONE',  ( -39.31656870549072380, -73.61799623142519522, -7.217717631503997033 ) ) ;
#14178=CARTESIAN_POINT ( 'NONE',  ( 21.49088915159999758, -36.91774715450000599, -8.428213728399999383 ) ) ;
#14179=CARTESIAN_POINT ( 'NONE',  ( -7.627568735119999666, -74.00000000000000000, -38.62788659690000515 ) ) ;
#14180=ORIENTED_EDGE ( 'NONE', *, *, #7384, .T. ) ;
#14181=TOROIDAL_SURFACE ( 'NONE', #24397, 3.500000000000000000, 0.5000000000000000000 ) ;
#14182=LINE ( 'NONE', #23868, #4584 ) ;
#14186=CARTESIAN_POINT ( 'NONE',  ( 6.850353673539999910, -36.56979899590000116, -21.56931441210000244 ) ) ;
#14191=CARTESIAN_POINT ( 'NONE',  ( -12.96004524251607570, -19.48405186614310480, 19.61898934477310519 ) ) ;
#14192=DIRECTION ( 'NONE',  ( 0.000000000000000000, 1.000000000000000000, 0.000000000000000000 ) ) ;
#14194=AXIS2_PLACEMENT_3D ( 'NONE', #26571, #18121, #4561 ) ;
#14195=CARTESIAN_POINT ( 'NONE',  ( -1.163833269605216492, -19.46453794989949770, -22.07359787591765610 ) ) ;
#14198=CARTESIAN_POINT ( 'NONE',  ( -2.013197380030000261, -45.98073373379999396, -23.47693395669999816 ) ) ;
#14200=EDGE_CURVE ( 'NONE', #21056, #7866, #3718, .T. ) ;
#14201=CARTESIAN_POINT ( 'NONE',  ( -38.71641004229999794, -73.50000000000000000, 7.135467526410000261 ) ) ;
#14203=CARTESIAN_POINT ( 'NONE',  ( 21.57753409760000096, -40.74985578519999763, -7.517162733340000180 ) ) ;
#14204=ADVANCED_FACE ( 'NONE', ( #12438 ), #1144, .T. ) ;
#14211=AXIS2_PLACEMENT_3D ( 'NONE', #985, #25572, #25148 ) ;
#14214=CARTESIAN_POINT ( 'NONE',  ( 7.844208135530000625, -36.11002484140000490, -21.41825414589999710 ) ) ;
#14216=CONICAL_SURFACE ( 'NONE', #8580, 25.14975229270001833, 0.4276056667390000787 ) ;
#14217=CARTESIAN_POINT ( 'NONE',  ( -1.993723132860002245, -52.61368720119944697, -23.68602550419998209 ) ) ;
#14218=DIRECTION ( 'NONE',  ( 0.000000000000000000, 1.000000000000000000, 0.000000000000000000 ) ) ;
#14222=CARTESIAN_POINT ( 'NONE',  ( 31.23163825569150731, -74.11403145701621042, -23.50616654247474813 ) ) ;
#14224=EDGE_LOOP ( 'NONE', ( #5379, #1189, #17267, #8806, #11643, #15896, #19521 ) ) ;
#14225=CARTESIAN_POINT ( 'NONE',  ( 23.03829042120000281, -52.56313962710000709, 10.32398954119999956 ) ) ;
#14228=B_SPLINE_CURVE_WITH_KNOTS ( 'NONE', 5,
 ( #12295, #21206, #18449, #3017, #27487, #27636 ),
 .UNSPECIFIED., .F., .F.,
 ( 6, 6 ),
 ( 0.000000000000000000, 1.000000000000000000 ),
 .UNSPECIFIED. ) ;
#14231=CARTESIAN_POINT ( 'NONE',  ( 23.56216202090000067, -73.65810230149999427, -30.93625454709999900 ) ) ;
#14232=EDGE_CURVE ( 'NONE', #5689, #26262, #4111, .T. ) ;
#14236=CARTESIAN_POINT ( 'NONE',  ( 7.691806989790000770, -28.53090832400000210, -20.98512114160000053 ) ) ;
#14237=CARTESIAN_POINT ( 'NONE',  ( -0.5413028987460000163, -57.47855601759999900, -23.35488904649999853 ) ) ;
#14239=ORIENTED_EDGE ( 'NONE', *, *, #301, .F. ) ;
#14240=EDGE_CURVE ( 'NONE', #13063, #23453, #11065, .T. ) ;
#14241=ORIENTED_EDGE ( 'NONE', *, *, #19698, .T. ) ;
#14242=CARTESIAN_POINT ( 'NONE',  ( -2.585646219300000048, -58.19955223950000089, -25.25977729030000063 ) ) ;
#14247=CARTESIAN_POINT ( 'NONE',  ( 22.08144638359999945, -37.65454154180000046, -8.887095524860001206 ) ) ;
#14248=DIRECTION ( 'NONE',  ( -0.000000000000000000, 1.000000000000000000, 0.000000000000000000 ) ) ;
#14251=DIRECTION ( 'NONE',  ( -0.9295286103719527793, 0.000000000000000000, -0.3687499999999814260 ) ) ;
#14252=DIRECTION ( 'NONE',  ( 0.000000000000000000, -1.000000000000000000, 0.000000000000000000 ) ) ;
#14253=CARTESIAN_POINT ( 'NONE',  ( -14.81965868650000040, -80.12520894669999905, 36.34494071330000509 ) ) ;
#14254=CARTESIAN_POINT ( 'NONE',  ( -2.686253848720000281, -64.98911155900000836, -26.08437766659999824 ) ) ;
#14255=CARTESIAN_POINT ( 'NONE',  ( -13.44405896729999839, -68.28990507160000334, 22.97003116759999841 ) ) ;
#14257=CARTESIAN_POINT ( 'NONE',  ( -14.66608910859999959, -79.49999990052810972, 36.47374631070000106 ) ) ;
#14260=CARTESIAN_POINT ( 'NONE',  ( 25.02058483049999538, -57.41946977210000114, 1.375913446200000001 ) ) ;
#14261=CARTESIAN_POINT ( 'NONE',  ( -20.55514986509999886, -63.54004463729999230, 13.57251594750000123 ) ) ;
#14262=ORIENTED_EDGE ( 'NONE', *, *, #13690, .T. ) ;
#14263=CARTESIAN_POINT ( 'NONE',  ( 0.000000000000000000, -89.00000000000000000, 0.000000000000000000 ) ) ;
#14264=CARTESIAN_POINT ( 'NONE',  ( -2.900367791859999933, -18.50000000000000000, -22.38632968349999786 ) ) ;
#14267=CARTESIAN_POINT ( 'NONE',  ( -14.16021440419999955, -18.50000000000000000, 19.51963099740000018 ) ) ;
#14271=CARTESIAN_POINT ( 'NONE',  ( -12.99961906594058370, -67.23928497083132072, 22.67538121095307346 ) ) ;
#14273=CARTESIAN_POINT ( 'NONE',  ( -11.54098094750000136, -61.67863912299999640, -22.71160036779999913 ) ) ;
#14274=CARTESIAN_POINT ( 'NONE',  ( 25.99810659739999963, -69.13393204870000375, -10.72511447639999993 ) ) ;
#14276=ORIENTED_EDGE ( 'NONE', *, *, #19435, .T. ) ;
#14277=EDGE_CURVE ( 'NONE', #22701, #10529, #6624, .T. ) ;
#14281=CARTESIAN_POINT ( 'NONE',  ( -12.31618287409999901, -19.44965574909999617, 19.12321486129999926 ) ) ;
#14284=DIRECTION ( 'NONE',  ( 0.000000000000000000, 1.000000000000000000, 0.000000000000000000 ) ) ;
#14288=CARTESIAN_POINT ( 'NONE',  ( -11.29202010641374621, -19.46468326931980997, -18.92074617257421920 ) ) ;
#14289=FACE_OUTER_BOUND ( 'NONE', #11706, .T. ) ;
#14291=CARTESIAN_POINT ( 'NONE',  ( 47.09481590257341566, -79.53590158212925587, -1.887627026932961138 ) ) ;
#14294=EDGE_CURVE ( 'NONE', #25354, #3493, #13303, .T. ) ;
#14295=DIRECTION ( 'NONE',  ( -1.000000000000000000, 0.000000000000000000, -3.154042683594194627E-16 ) ) ;
#14296=CARTESIAN_POINT ( 'NONE',  ( -32.61798281429999946, -80.00000000000000000, -22.71848787769999944 ) ) ;
#14303=CARTESIAN_POINT ( 'NONE',  ( -19.51583823489999858, -52.61368720120000120, 13.56962763329999966 ) ) ;
#14305=CARTESIAN_POINT ( 'NONE',  ( 31.96452224769999617, -73.88714870409999946, -21.93835394839999964 ) ) ;
#14306=CARTESIAN_POINT ( 'NONE',  ( 23.56559805210000036, -58.81638232979999970, -9.577937461890000392 ) ) ;
#14308=ORIENTED_EDGE ( 'NONE', *, *, #11539, .T. ) ;
#14311=ADVANCED_FACE ( 'NONE', ( #8506 ), #27416, .T. ) ;
#14313=CARTESIAN_POINT ( 'NONE',  ( 20.26985721470000001, -35.99252858750000428, -9.303161554559999047 ) ) ;
#14317=B_SPLINE_SURFACE_WITH_KNOTS ( 'NONE', 5, 5, ( 
 ( #12575, #7688, #23400, #23540, #25865, #7812, #12166, #28049, #1545 ),
 ( #21346, #10250, #10105, #25313, #12436, #19302, #27911, #21489, #27646 ),
 ( #5341, #1405, #1140, #28186, #5757, #5616, #3576, #12019, #16553 ),
 ( #14770, #3715, #8217, #14231, #7949, #14499, #16837, #14367, #23260 ),
 ( #18892, #20936, #14641, #19025, #25449, #3165, #9978, #8087, #3303 ),
 ( #27774, #16686, #25590, #3440, #19163, #5892, #23119, #5480, #996 ) ),
 .UNSPECIFIED., .F., .F., .F.,
 ( 6, 6 ),
 ( 6, 3, 6 ),
 ( 0.000000000000000000, 12.56695009720000122 ),
 ( 0.000000000000000000, 1.000000000000000000, 2.000000000000000000 ),
 .UNSPECIFIED. ) ;
#14318=CARTESIAN_POINT ( 'NONE',  ( -21.05833095636783270, -65.01950792717818217, 13.71407545850738785 ) ) ;
#14321=ADVANCED_FACE ( 'NONE', ( #4288 ), #11095, .T. ) ;
#14324=AXIS2_PLACEMENT_3D ( 'NONE', #17824, #361, #8765 ) ;
#14325=CARTESIAN_POINT ( 'NONE',  ( -40.42867112537203411, -74.28469014306668328, 7.237400523868926072 ) ) ;
#14327=CARTESIAN_POINT ( 'NONE',  ( -12.98455916887866479, -19.48459622965902938, 19.64307623567460936 ) ) ;
#14330=CARTESIAN_POINT ( 'NONE',  ( 19.98345451299999809, -18.50000000000000000, -7.491375432139999901 ) ) ;
#14331=DIRECTION ( 'NONE',  ( 0.000000000000000000, -1.000000000000000000, 0.000000000000000000 ) ) ;
#14334=CARTESIAN_POINT ( 'NONE',  ( -1.851961808682860200, -74.06886391613052467, 47.01299730337805016 ) ) ;
#14337=CARTESIAN_POINT ( 'NONE',  ( 22.83553957720000227, -53.24879282940000280, -9.272014655159999563 ) ) ;
#14338=CARTESIAN_POINT ( 'NONE',  ( -39.48500436417592141, -74.13942000225500806, -7.435977656810683456 ) ) ;
#14339=CARTESIAN_POINT ( 'NONE',  ( 36.24656906829999770, -74.82938568209999630, -15.05817820240000060 ) ) ;
#14346=AXIS2_PLACEMENT_3D ( 'NONE', #27974, #10576, #8011 ) ;
#14347=CARTESIAN_POINT ( 'NONE',  ( 21.12347101519999981, -34.87913938230000355, -8.043102957309999468 ) ) ;
#14349=AXIS2_PLACEMENT_3D ( 'NONE', #26217, #10727, #6245 ) ;
#14350=DIRECTION ( 'NONE',  ( 1.000000000000000000, 0.000000000000000000, 0.000000000000000000 ) ) ;
#14351=CARTESIAN_POINT ( 'NONE',  ( -3.252988965690000178, -72.00000000000000000, -30.32986301179999700 ) ) ;
#14352=CARTESIAN_POINT ( 'NONE',  ( -39.48497135293115434, -74.13941005061472822, 7.435983480943145096 ) ) ;
#14354=DIRECTION ( 'NONE',  ( 0.000000000000000000, 0.000000000000000000, -1.000000000000000000 ) ) ;
#14356=CARTESIAN_POINT ( 'NONE',  ( -1.061013842608576230, -66.63438001457079451, -25.83911284170473621 ) ) ;
#14360=DIRECTION ( 'NONE',  ( 1.000000000000000000, 0.000000000000000000, 0.000000000000000000 ) ) ;
#14361=EDGE_CURVE ( 'NONE', #15244, #10596, #7326, .T. ) ;
#14364=DIRECTION ( 'NONE',  ( 0.9144078985680119676, 0.000000000000000000, 0.4047940155640056270 ) ) ;
#14365=CARTESIAN_POINT ( 'NONE',  ( 19.97576656849999921, -36.00000000000000000, -19.97576656849999921 ) ) ;
#14367=CARTESIAN_POINT ( 'NONE',  ( 23.69384752110000036, -72.68281501180000248, -30.54094685289999944 ) ) ;
#14371=VECTOR ( 'NONE', #2533, 1000.000000000000114 ) ;
#14373=CARTESIAN_POINT ( 'NONE',  ( 8.965967837319999134, -34.65022641339999865, -19.90557312019999969 ) ) ;
#14374=FACE_OUTER_BOUND ( 'NONE', #19924, .T. ) ;
#14375=CARTESIAN_POINT ( 'NONE',  ( 40.00000000000000000, -73.50000000000000000, 2.065014825799999939E-15 ) ) ;
#14378=VERTEX_POINT ( 'NONE', #6178 ) ;
#14379=CARTESIAN_POINT ( 'NONE',  ( -1.156101949690000019, -58.35063071660000134, -23.44148674059999848 ) ) ;
#14380=AXIS2_PLACEMENT_3D ( 'NONE', #1729, #10570, #28372 ) ;
#14384=ORIENTED_EDGE ( 'NONE', *, *, #1633, .F. ) ;
#14390=CYLINDRICAL_SURFACE ( 'NONE', #3681, 3.000000000000001332 ) ;
#14391=ORIENTED_EDGE ( 'NONE', *, *, #7478, .T. ) ;
#14392=CARTESIAN_POINT ( 'NONE',  ( 7.611151840291949355, -37.24567261342306068, -21.50381023462963270 ) ) ;
#14395=CARTESIAN_POINT ( 'NONE',  ( -3.296126547070000079, -69.13896873960000278, -27.54013567880000224 ) ) ;
#14396=ORIENTED_EDGE ( 'NONE', *, *, #12465, .F. ) ;
#14399=DIRECTION ( 'NONE',  ( 1.000000000000000000, 0.000000000000000000, 0.000000000000000000 ) ) ;
#14400=CARTESIAN_POINT ( 'NONE',  ( -20.47698326670000313, -61.75818586239999775, 14.68202960460000028 ) ) ;
#14403=CARTESIAN_POINT ( 'NONE',  ( -0.5335602090290000321, -52.63293862049999916, -23.18581005440000098 ) ) ;
#14404=CARTESIAN_POINT ( 'NONE',  ( -2.987826558189999648, -18.62337006899999992, -24.35058490870000014 ) ) ;
#14406=ORIENTED_EDGE ( 'NONE', *, *, #16193, .T. ) ;
#14408=AXIS2_PLACEMENT_3D ( 'NONE', #4526, #13405, #22022 ) ;
#14410=CARTESIAN_POINT ( 'NONE',  ( 36.36887067909999871, -79.00000000000000000, -14.85406736540000061 ) ) ;
#14413=UNCERTAINTY_MEASURE_WITH_UNIT (LENGTH_MEASURE( 1.000000000000000082E-05 ), #1808, 'distance_accuracy_value', 'NONE');
#14416=ORIENTED_EDGE ( 'NONE', *, *, #1109, .F. ) ;
#14418=CARTESIAN_POINT ( 'NONE',  ( 46.40078773993090522, -73.62157574275342142, -3.405080668251522003 ) ) ;
#14420=CARTESIAN_POINT ( 'NONE',  ( -10.91687328849999794, -19.46548165690000332, 19.14227818649999691 ) ) ;
#14421=DIRECTION ( 'NONE',  ( 0.9408314849018030168, 0.000000000000000000, -0.3388747807339287377 ) ) ;
#14425=EDGE_CURVE ( 'NONE', #27919, #26201, #12499, .T. ) ;
#14427=CARTESIAN_POINT ( 'NONE',  ( 38.71640952649999434, -73.65708014139998738, 7.135466514619999145 ) ) ;
#14428=CARTESIAN_POINT ( 'NONE',  ( 25.57115952125134939, -69.12177585505048683, -8.648957911665412723 ) ) ;
#14431=VERTEX_POINT ( 'NONE', #1924 ) ;
#14435=CARTESIAN_POINT ( 'NONE',  ( -9.476764215410000247, -84.00000000000000000, 38.08875739639999836 ) ) ;
#14436=ORIENTED_EDGE ( 'NONE', *, *, #6399, .T. ) ;
#14437=CARTESIAN_POINT ( 'NONE',  ( -1.441012333810000046, -80.05618323510000778, 47.15972982670000135 ) ) ;
#14438=CARTESIAN_POINT ( 'NONE',  ( -1.776356839399999804E-15, -79.50000000000000000, 47.25000000000000000 ) ) ;
#14441=CARTESIAN_POINT ( 'NONE',  ( -36.23922253580000330, -74.00000000000000000, -26.33972759919999973 ) ) ;
#14442=CARTESIAN_POINT ( 'NONE',  ( 10.33697414329999908, -72.00000000000000000, -28.69893982729999848 ) ) ;
#14443=CARTESIAN_POINT ( 'NONE',  ( 30.97095762050000189, -72.31416070160000231, -20.30102759929999934 ) ) ;
#14445=CARTESIAN_POINT ( 'NONE',  ( -14.37578563377381435, -74.06475120341723084, 36.25117000458550365 ) ) ;
#14449=ADVANCED_FACE ( 'NONE', ( #19676 ), #10345, .T. ) ;
#14450=B_SPLINE_CURVE_WITH_KNOTS ( 'NONE', 5,
 ( #1074, #16621, #6099, #3645, #17042, #8282 ),
 .UNSPECIFIED., .F., .F.,
 ( 6, 6 ),
 ( 0.000000000000000000, 1.000000000000000000 ),
 .UNSPECIFIED. ) ;
#14451=CARTESIAN_POINT ( 'NONE',  ( 20.05332756480000000, -35.50840382379999483, -8.956869086990002060 ) ) ;
#14453=CARTESIAN_POINT ( 'NONE',  ( 20.34791740889999900, -35.98209074209999159, -9.112674168019999854 ) ) ;
#14454=CARTESIAN_POINT ( 'NONE',  ( -21.69554430422256175, -79.50000022090000584, -32.70900267937481942 ) ) ;
#14457=DIRECTION ( 'NONE',  ( 0.000000000000000000, -1.000000000000000000, 0.000000000000000000 ) ) ;
#14460=DIRECTION ( 'NONE',  ( -0.9993816408608721114, 0.000000000000000000, 0.03516156865429537204 ) ) ;
#14463=VERTEX_POINT ( 'NONE', #11048 ) ;
#14464=LINE ( 'NONE', #25274, #6757 ) ;
#14468=ORIENTED_EDGE ( 'NONE', *, *, #21838, .F. ) ;
#14469=CARTESIAN_POINT ( 'NONE',  ( 18.85230044180000064, -18.50000000000000000, -8.028472989679999117 ) ) ;
#14472=CARTESIAN_POINT ( 'NONE',  ( -1.000575989186441417, -74.24539519982145919, 47.18104523406701389 ) ) ;
#14473=EDGE_CURVE ( 'NONE', #6167, #17563, #6003, .T. ) ;
#14474=CARTESIAN_POINT ( 'NONE',  ( 21.47211211410000331, -36.57019168810000309, -7.156454249520000310 ) ) ;
#14476=CARTESIAN_POINT ( 'NONE',  ( -11.17082021589999918, -34.59963798429999571, -22.14893711949999755 ) ) ;
#14479=CARTESIAN_POINT ( 'NONE',  ( -22.13232332860000184, -74.50000000000000000, -32.73892504640000567 ) ) ;
#14480=CIRCLE ( 'NONE', #10707, 3.000000000000002665 ) ;
#14484=CARTESIAN_POINT ( 'NONE',  ( 20.39306988279999899, -34.78953926309999645, -8.798269974460000142 ) ) ;
#14486=DIRECTION ( 'NONE',  ( 0.000000000000000000, 1.000000000000000000, 0.000000000000000000 ) ) ;
#14487=CARTESIAN_POINT ( 'NONE',  ( 0.000000000000000000, -80.50000000000000000, 0.000000000000000000 ) ) ;
#14491=ORIENTED_EDGE ( 'NONE', *, *, #13382, .T. ) ;
#14492=CARTESIAN_POINT ( 'NONE',  ( -13.18754275750000104, -69.02891040180000459, -23.50545369980000032 ) ) ;
#14494=CARTESIAN_POINT ( 'NONE',  ( -11.93462531391737791, -19.46927944529031151, 19.09349998647691393 ) ) ;
#14499=CARTESIAN_POINT ( 'NONE',  ( 23.62363097839999782, -73.01595982080000624, -30.63067135909999905 ) ) ;
#14501=CARTESIAN_POINT ( 'NONE',  ( 28.69894246159999796, -72.00000000000000000, -10.33698060819999931 ) ) ;
#14507=ORIENTED_EDGE ( 'NONE', *, *, #21578, .T. ) ;
#14508=EDGE_CURVE ( 'NONE', #22866, #7412, #16245, .T. ) ;
#14511=ADVANCED_FACE ( 'NONE', ( #187 ), #11508, .T. ) ;
#14513=DIRECTION ( 'NONE',  ( 0.9952295494196653491, 0.000000000000000000, -0.09756097560976997873 ) ) ;
#14515=FACE_OUTER_BOUND ( 'NONE', #10768, .T. ) ;
#14518=DIRECTION ( 'NONE',  ( 0.000000000000000000, 1.000000000000000000, 0.000000000000000000 ) ) ;
#14521=CARTESIAN_POINT ( 'NONE',  ( 9.107729735749998667, -35.83389485320000034, -19.55231199680000387 ) ) ;
#14522=CARTESIAN_POINT ( 'NONE',  ( 21.84994998139999822, -44.93330283399999558, -6.931585813899999948 ) ) ;
#14524=CARTESIAN_POINT ( 'NONE',  ( -16.01759400379999931, -69.30633957129998635, 23.18138418170000037 ) ) ;
#14528=CARTESIAN_POINT ( 'NONE',  ( -32.83566817730000054, -74.50000000000000000, -22.22906645950000026 ) ) ;
#14531=DIRECTION ( 'NONE',  ( -1.000000000000000000, 0.000000000000000000, 0.000000000000000000 ) ) ;
#14533=CARTESIAN_POINT ( 'NONE',  ( -3.035021987659999976, -18.62259217289999924, -24.02173570430000282 ) ) ;
#14534=CARTESIAN_POINT ( 'NONE',  ( 36.60600030368150470, -74.15649605208299988, -14.28714990587511124 ) ) ;
#14535=ORIENTED_EDGE ( 'NONE', *, *, #15956, .F. ) ;
#14536=EDGE_CURVE ( 'NONE', #16695, #13357, #23254, .T. ) ;
#14537=CARTESIAN_POINT ( 'NONE',  ( 0.000000000000000000, -19.00000000000000000, 0.000000000000000000 ) ) ;
#14538=FACE_OUTER_BOUND ( 'NONE', #21234, .T. ) ;
#14539=CARTESIAN_POINT ( 'NONE',  ( 36.54355158469999765, -79.59555342380001264, -14.63615714969999893 ) ) ;
#14541=ORIENTED_EDGE ( 'NONE', *, *, #12300, .F. ) ;
#14544=B_SPLINE_SURFACE_WITH_KNOTS ( 'NONE', 5, 5, ( 
 ( #11766, #18781, #11914, #20966, #13958, #3193 ),
 ( #2754, #2905, #7711, #16579, #25471, #13808 ),
 ( #5506, #18485, #5371, #11610, #16437, #27376 ),
 ( #9434, #14395, #5072, #7417, #23146, #23285 ),
 ( #20818, #20523, #591, #18342, #25341, #12051 ),
 ( #7269, #16135, #20676, #25038, #22864, #880 ),
 ( #737, #18632, #16282, #9722, #27529, #1027 ),
 ( #9585, #14254, #25197, #5226, #14110, #23009 ),
 ( #3059, #7574, #5024, #13315, #15497, #9389 ) ),
 .UNSPECIFIED., .F., .F., .F.,
 ( 6, 3, 6 ),
 ( 6, 6 ),
 ( 41.71218049600000199, 49.83411874629999971, 53.81665561330000003 ),
 ( 0.000000000000000000, 2.000000000000000000 ),
 .UNSPECIFIED. ) ;
#14546=CARTESIAN_POINT ( 'NONE',  ( -1.226789154321535680, -79.95994320750210704, 47.14707426476502405 ) ) ;
#14550=AXIS2_PLACEMENT_3D ( 'NONE', #8837, #4634, #293 ) ;
#14553=ORIENTED_EDGE ( 'NONE', *, *, #11802, .F. ) ;
#14555=CARTESIAN_POINT ( 'NONE',  ( 27.49607050420000220, -19.50000000000000000, 1.934818144049999855 ) ) ;
#14556=DIRECTION ( 'NONE',  ( 1.000000000000000000, 0.000000000000000000, 0.000000000000000000 ) ) ;
#14557=ORIENTED_EDGE ( 'NONE', *, *, #26819, .T. ) ;
#14558=CARTESIAN_POINT ( 'NONE',  ( 23.35417726369999869, -57.47855601759999900, -0.5711878298099999363 ) ) ;
#14560=CARTESIAN_POINT ( 'NONE',  ( 47.16844854119278807, -79.40106950755198056, -1.389656841691803590 ) ) ;
#14563=CARTESIAN_POINT ( 'NONE',  ( 8.965966766827932588, -34.65022632772699751, -19.90557426916371497 ) ) ;
#14564=CARTESIAN_POINT ( 'NONE',  ( 8.986258419809999509, -35.50000000000000000, -19.49544308430000328 ) ) ;
#14565=DIRECTION ( 'NONE',  ( -0.7071067811865475727, 0.000000000000000000, -0.7071067811865475727 ) ) ;
#14566=CARTESIAN_POINT ( 'NONE',  ( -2.567353809430000133, -52.57401960349999825, -24.80239345940000106 ) ) ;
#14567=B_SPLINE_CURVE_WITH_KNOTS ( 'NONE', 3,
 ( #22413, #5062, #22258, #15835, #9131, #22566, #6674, #13501, #9280, #4630, #18180, #27077, #13800, #13660, #15983, #22705, #13951, #24746, #26790, #8985, #6972, #2460 ),
 .UNSPECIFIED., .F., .F.,
 ( 4, 2, 1, 1, 1, 2, 2, 2, 1, 1, 1, 2, 2, 4 ),
 ( 0.000000000000000000, 0.1250000000000226208, 0.1875000000000338340, 0.2187500000000397460, 0.2343750000000427991, 0.2421875000000443257, 0.2500000000000458522, 0.3750000000000830447, 0.4375000000000992539, 0.4687500000001053602, 0.4843750000001084133, 0.4921875000001078027, 0.5000000000001071365, 1.000000000000000000 ),
 .UNSPECIFIED. ) ;
#14569=CARTESIAN_POINT ( 'NONE',  ( -2.675072049550000219E-13, -79.50000000000000000, 47.25000000000000000 ) ) ;
#14571=ORIENTED_EDGE ( 'NONE', *, *, #8516, .F. ) ;
#14573=CARTESIAN_POINT ( 'NONE',  ( 36.24656994149999889, -79.00000000000000000, -15.05817610060000078 ) ) ;
#14576=CARTESIAN_POINT ( 'NONE',  ( 32.20446920490000053, -74.00073021550001329, -21.99457402419999852 ) ) ;
#14578=CARTESIAN_POINT ( 'NONE',  ( -14.20278481966783168, -74.02954850625619088, 36.23557363773064566 ) ) ;
#14580=EDGE_CURVE ( 'NONE', #13695, #2130, #27439, .T. ) ;
#14581=DIRECTION ( 'NONE',  ( 1.000000000000000000, 0.000000000000000000, 0.000000000000000000 ) ) ;
#14583=CARTESIAN_POINT ( 'NONE',  ( 9.698193454340000130, -36.00000000010000178, -20.58262106160000116 ) ) ;
#14584=CARTESIAN_POINT ( 'NONE',  ( -40.14660266887646856, -74.07739338315893463, -7.248706349658688097 ) ) ;
#14586=CARTESIAN_POINT ( 'NONE',  ( 21.24969070070000043, -36.48513442969999687, -8.723503615720002102 ) ) ;
#14590=DIRECTION ( 'NONE',  ( -5.788992577199999305E-17, 0.000000000000000000, 1.000000000000000000 ) ) ;
#14596=ORIENTED_EDGE ( 'NONE', *, *, #15609, .F. ) ;
#14599=CARTESIAN_POINT ( 'NONE',  ( 26.38387136229999896, -71.18862645909999287, 10.78376531940000049 ) ) ;
#14601=ORIENTED_EDGE ( 'NONE', *, *, #24534, .F. ) ;
#14602=CARTESIAN_POINT ( 'NONE',  ( 20.63161943080000071, -19.46510050319999863, -7.734358783100000245 ) ) ;
#14604=CARTESIAN_POINT ( 'NONE',  ( -14.67203031310000050, -74.27627443250000283, 36.35843490820000312 ) ) ;
#14607=ORIENTED_EDGE ( 'NONE', *, *, #15360, .F. ) ;
#14608=EDGE_CURVE ( 'NONE', #26756, #5668, #15273, .T. ) ;
#14611=AXIS2_PLACEMENT_3D ( 'NONE', #18360, #611, #22733 ) ;
#14614=CARTESIAN_POINT ( 'NONE',  ( 7.727580379730000004, -65.07443080049999651, -23.93312984690000178 ) ) ;
#14616=CARTESIAN_POINT ( 'NONE',  ( 22.30996026260000065, -58.68498324060000471, 10.16715434780000038 ) ) ;
#14617=ORIENTED_EDGE ( 'NONE', *, *, #17692, .T. ) ;
#14618=B_SPLINE_CURVE_WITH_KNOTS ( 'NONE', 5,
 ( #15587, #7305, #11648, #24486, #17789, #18077 ),
 .UNSPECIFIED., .F., .F.,
 ( 6, 6 ),
 ( 0.000000000000000000, 1.000000000000000000 ),
 .UNSPECIFIED. ) ;
#14622=CARTESIAN_POINT ( 'NONE',  ( 7.836711220800001598, -35.70895110779999726, -21.34303704659999568 ) ) ;
#14623=CARTESIAN_POINT ( 'NONE',  ( 7.246150394359973212, -73.82038814068835109, 39.74699101863826201 ) ) ;
#14624=TOROIDAL_SURFACE ( 'NONE', #12309, 43.34897771020000334, 20.00000000000000000 ) ;
#14626=DIRECTION ( 'NONE',  ( -0.7975023596669910120, 0.000000000000000000, -0.6033158263509930119 ) ) ;
#14629=CARTESIAN_POINT ( 'NONE',  ( 19.14378155729999875, -25.56710285120000137, -9.006608812259999652 ) ) ;
#14633=CARTESIAN_POINT ( 'NONE',  ( 20.33566493080000015, -36.00000000000000000, -9.885503730140001721 ) ) ;
#14635=CARTESIAN_POINT ( 'NONE',  ( 40.00000000000000000, -73.50000000000000000, 2.065014825799999939E-15 ) ) ;
#14636=VERTEX_POINT ( 'NONE', #27710 ) ;
#14637=CARTESIAN_POINT ( 'NONE',  ( 25.33520153630000138, -65.80271596200000772, -10.35056873939999988 ) ) ;
#14639=CARTESIAN_POINT ( 'NONE',  ( -40.00000000000000000, -73.50000000000000000, 3.397282455350000038E-15 ) ) ;
#14641=CARTESIAN_POINT ( 'NONE',  ( 21.89558901659999890, -73.74042638279999551, -31.74625209310000429 ) ) ;
#14642=EDGE_CURVE ( 'NONE', #8148, #20809, #479, .T. ) ;
#14643=ADVANCED_FACE ( 'NONE', ( #18386 ), #26859, .T. ) ;
#14644=CARTESIAN_POINT ( 'NONE',  ( -22.23253203089999985, -69.48726973570001064, 15.83344364000000049 ) ) ;
#14645=CIRCLE ( 'NONE', #17918, 3.750000000000000000 ) ;
#14647=CARTESIAN_POINT ( 'NONE',  ( -12.05063396289999922, -64.89165752090001149, -22.22490323269999735 ) ) ;
#14650=CARTESIAN_POINT ( 'NONE',  ( 9.457230477735794949, -35.99973515773508126, -20.00996444815637432 ) ) ;
#14651=EDGE_CURVE ( 'NONE', #24358, #27117, #20459, .T. ) ;
#14652=CIRCLE ( 'NONE', #21181, 2.000000000000001332 ) ;
#14655=CARTESIAN_POINT ( 'NONE',  ( -2.530235925970000022, -63.52052399810000338, -25.57870722859999901 ) ) ;
#14656=CARTESIAN_POINT ( 'NONE',  ( 33.25000000000000000, -69.50000000000000000, -1.707239799929999782E-15 ) ) ;
#14658=EDGE_CURVE ( 'NONE', #22615, #23918, #13452, .T. ) ;
#14659=AXIS2_PLACEMENT_3D ( 'NONE', #20399, #619, #16164 ) ;
#14660=VERTEX_POINT ( 'NONE', #28112 ) ;
#14661=CARTESIAN_POINT ( 'NONE',  ( -7.498737045662836387, -73.99999999999910472, 38.65106196168373032 ) ) ;
#14662=EDGE_CURVE ( 'NONE', #21398, #5069, #16993, .T. ) ;
#14664=DIRECTION ( 'NONE',  ( 0.4692400087391608854, 0.000000000000000000, -0.8830706733883039172 ) ) ;
#14665=CARTESIAN_POINT ( 'NONE',  ( 9.151216319970000512, -35.87888623290000112, -19.56023227720000079 ) ) ;
#14667=CARTESIAN_POINT ( 'NONE',  ( 38.79561088300408045, -74.00013394014689538, 7.600490370444946464 ) ) ;
#14668=VERTEX_POINT ( 'NONE', #19365 ) ;
#14671=CARTESIAN_POINT ( 'NONE',  ( -32.67765636376323357, -74.21958180435098029, -22.19105059018374249 ) ) ;
#14672=CARTESIAN_POINT ( 'NONE',  ( 36.34100412979999817, -74.29447080869999809, -14.83252444919999924 ) ) ;
#14676=CARTESIAN_POINT ( 'NONE',  ( -3.160010391330000168, -18.50000000000000000, -22.19765357320000376 ) ) ;
#14679=CLOSED_SHELL ( 'NONE', ( #22519, #26991, #6036, #22003, #5902, #17066, #9491, #17163, #25042, #17558, #16054, #23862, #24411, #22990, #19157, #12541, #17660, #14029, #15906, #12616, #14311, #12444, #25086, #13620, #6961, #8605, #25571, #13512, #7260, #13813, #6259, #27606, #28610, #20885, #22926, #13726, #15164, #12712, #28450, #12801, #28580, #533, #4248, #20353, #20949, #15446, #868, #9513, #20138, #23579, #17737, #5541, #1492, #24598, #24033, #21932, #28570, #25157, #19952, #26082, #18648, #8591, #26551, #26299, #1343, #18268, #27428, #15918, #23838, #25294, #1068, #3063, #24248, #20022, #13446, #738, #12548, #28029, #19860, #23240, #28644, #14695, #14944, #20679, #26348, #2823, #16320, #28721, #5561, #5472, #23680, #6218, #14643, #15075, #10249, #13854, #15736, #4661, #1911, #14449, #18578, #25847, #24916, #16318, #18189, #23150, #1539, #15436, #334, #15158, #5447, #10578, #3441, #12386, #28796, #11258, #7935, #21137, #8371, #28034, #25485, #13210, #1097, #16052, #4739, #6585, #27066, #17468, #4204, #12989, #7813, #22317, #27725, #706, #19573, #14060, #18204, #15049, #6365, #15403, #11944, #21290, #26783, #14097, #17742, #18305, #19282, #28091, #10199, #14511, #10164, #17972, #20614, #16916, #28208, #9203, #18676, #19981, #26552, #4787, #3098, #24787, #24851, #9501, #7418, #4126, #10516, #1219, #27266, #9809, #17012, #28584, #2311, #9134, #22213, #1365, #15119, #19271, #11074, #24685, #21324, #18718, #21946, #16647, #20394, #19758, #27316, #4380, #27828, #14132, #1445, #3655, #12451, #1247, #13132, #28269, #8207, #17154, #14321, #12192, #24348, #18067, #15573, #2792, #23534, #14851, #5113, #55, #729, #22653, #18604, #27934, #26193, #12037, #17633, #21972, #9330, #4951, #22715, #11913, #23272, #25348, #23236, #5110, #28508, #27576, #24637, #3773, #25983, #10212, #23851, #10705, #21, #1039, #9930, #4535, #19925, #19856, #24338, #13889, #20342, #3854, #16328, #23682, #3539, #2088, #28062, #11850, #26019, #21675, #9540, #25415, #20504, #21707, #27096, #16938, #24441, #8507, #20100, #25671, #15372, #15355, #5497, #15990, #24474, #23881, #830, #27293, #19184, #27389, #26554, #2581, #10251, #13787, #4495, #10919, #22473, #24012, #5796, #19489, #7066, #21081, #796, #14204, #4779, #1183, #16028, #19571, #11533, #26763, #4543, #17135, #20881, #8862, #25885, #8129, #5695, #15495, #10398, #13183, #10021, #19150, #19343, #25613, #19597, #3316, #5752, #6374, #27431, #18339 ) ) ;
#14680=CARTESIAN_POINT ( 'NONE',  ( -7.215414233289999757, -84.00000000000000000, 40.70731707320000226 ) ) ;
#14681=CARTESIAN_POINT ( 'NONE',  ( -31.64302845809999809, -79.50000000000000000, -31.64302845809999809 ) ) ;
#14682=CARTESIAN_POINT ( 'NONE',  ( 36.24656994149999889, -79.27200282849999269, -15.05817610060000078 ) ) ;
#14684=CARTESIAN_POINT ( 'NONE',  ( -15.00047198269999882, -79.50000000000000000, 39.16845525979999820 ) ) ;
#14685=CIRCLE ( 'NONE', #20287, 2.000000000000001776 ) ;
#14690=CARTESIAN_POINT ( 'NONE',  ( 8.028473304129999377, -18.50000000000000000, -18.85230009969999898 ) ) ;
#14691=EDGE_LOOP ( 'NONE', ( #16988, #18789, #147, #25426 ) ) ;
#14694=DIRECTION ( 'NONE',  ( 0.000000000000000000, -1.000000000000000000, 0.000000000000000000 ) ) ;
#14695=ADVANCED_FACE ( 'NONE', ( #1738 ), #12500, .T. ) ;
#14698=CARTESIAN_POINT ( 'NONE',  ( 9.082471092209999597, -36.23996849139999910, -21.28200090970000247 ) ) ;
#14701=CARTESIAN_POINT ( 'NONE',  ( 25.58194701613479083, -68.15800876155556409, 10.86896338428304709 ) ) ;
#14704=CARTESIAN_POINT ( 'NONE',  ( 14.62430634820000108, -72.00000000000000000, 26.76961320899999919 ) ) ;
#14708=ORIENTED_EDGE ( 'NONE', *, *, #15779, .F. ) ;
#14709=B_SPLINE_CURVE_WITH_KNOTS ( 'NONE', 5,
 ( #25260, #16633, #22930, #27728, #20741, #799 ),
 .UNSPECIFIED., .F., .F.,
 ( 6, 6 ),
 ( 0.000000000000000000, 6.855861996789999857 ),
 .UNSPECIFIED. ) ;
#14710=CARTESIAN_POINT ( 'NONE',  ( 10.33697414329999908, -72.00000000000000000, -28.69893982729999848 ) ) ;
#14711=CARTESIAN_POINT ( 'NONE',  ( -19.15417045299999899, -18.86697026210000061, 14.26418949420000004 ) ) ;
#14716=CARTESIAN_POINT ( 'NONE',  ( 28.92477265019999777, -73.91965247389998694, -26.58576722179999763 ) ) ;
#14717=CARTESIAN_POINT ( 'NONE',  ( -16.56294617018072657, -72.37489744396329172, 23.47174545849500404 ) ) ;
#14722=CARTESIAN_POINT ( 'NONE',  ( 21.53016318250000083, -37.05551862909999983, -8.186295007220000031 ) ) ;
#14724=VERTEX_POINT ( 'NONE', #22576 ) ;
#14726=EDGE_CURVE ( 'NONE', #16034, #13313, #19042, .T. ) ;
#14729=CARTESIAN_POINT ( 'NONE',  ( 7.274533568879999912, -49.11506481659999679, -21.89436955060000045 ) ) ;
#14735=CARTESIAN_POINT ( 'NONE',  ( 39.48689401879786232, -73.68677077069324355, 7.232334316206437741 ) ) ;
#14737=CARTESIAN_POINT ( 'NONE',  ( 20.62158124919999835, -19.15810967940000253, -7.730595680639999578 ) ) ;
#14738=CARTESIAN_POINT ( 'NONE',  ( -14.29690427480000103, -74.09825332389999630, 36.44846386569999908 ) ) ;
#14741=ORIENTED_EDGE ( 'NONE', *, *, #4229, .T. ) ;
#14742=DIRECTION ( 'NONE',  ( 0.000000000000000000, -1.000000000000000000, 0.000000000000000000 ) ) ;
#14743=DIRECTION ( 'NONE',  ( 1.738658080640003812E-17, 0.000000000000000000, -1.000000000000000000 ) ) ;
#14745=CARTESIAN_POINT ( 'NONE',  ( -39.64169929219999489, -73.82505177980000610, -7.260629317050000253 ) ) ;
#14746=CARTESIAN_POINT ( 'NONE',  ( 20.68132854559999956, -58.35623000289999851, 10.95980495770000118 ) ) ;
#14751=CARTESIAN_POINT ( 'NONE',  ( -32.75504890064814845, -74.50000000070001249, -22.14844718283469760 ) ) ;
#14757=AXIS2_PLACEMENT_3D ( 'NONE', #2103, #15766, #26566 ) ;
#14758=CARTESIAN_POINT ( 'NONE',  ( 9.502793637310000818, -50.93917412489999919, -23.34524706979999920 ) ) ;
#14761=CARTESIAN_POINT ( 'NONE',  ( -12.04116395852593691, -49.87586154376180758, -19.70838305107999489 ) ) ;
#14763=ORIENTED_EDGE ( 'NONE', *, *, #21327, .T. ) ;
#14767=CARTESIAN_POINT ( 'NONE',  ( -7.265381620139999441, -73.99590173020000350, 39.73102114399999607 ) ) ;
#14768=CARTESIAN_POINT ( 'NONE',  ( 27.89292634430000106, -72.00000000000000000, 12.34776042340000046 ) ) ;
#14770=CARTESIAN_POINT ( 'NONE',  ( 23.59360194539999966, -74.10313260709999383, -31.26971289790000341 ) ) ;
#14773=DIRECTION ( 'NONE',  ( 0.000000000000000000, -1.000000000000000000, 0.000000000000000000 ) ) ;
#14774=CARTESIAN_POINT ( 'NONE',  ( -12.43380386830000006, -65.01950800350000748, -21.83872194130000111 ) ) ;
#14775=CARTESIAN_POINT ( 'NONE',  ( 7.187003541560001096, -35.30712889009999600, -21.41502073610000068 ) ) ;
#14779=CIRCLE ( 'NONE', #2231, 6.750000000000000000 ) ;
#14780=EDGE_LOOP ( 'NONE', ( #27133, #25441, #26022, #28285 ) ) ;
#14782=CARTESIAN_POINT ( 'NONE',  ( 6.850353625200000351, -36.56979901409999911, -21.56931447779999900 ) ) ;
#14783=AXIS2_PLACEMENT_3D ( 'NONE', #26508, #25357, #9599 ) ;
#14784=CARTESIAN_POINT ( 'NONE',  ( 9.324355421639999975, -37.67772341970000127, -22.72952601809999962 ) ) ;
#14788=CARTESIAN_POINT ( 'NONE',  ( 19.40204233298638670, -19.49096807709544521, -8.935689512806787249 ) ) ;
#14789=ORIENTED_EDGE ( 'NONE', *, *, #28286, .F. ) ;
#14790=CARTESIAN_POINT ( 'NONE',  ( 21.34291133579999666, -34.88462696900000282, -7.355130963909999764 ) ) ;
#14793=CARTESIAN_POINT ( 'NONE',  ( 7.688401808063399123, -37.38063849119085802, -21.51556169207930225 ) ) ;
#14794=EDGE_LOOP ( 'NONE', ( #24630, #7737, #7378, #24415 ) ) ;
#14796=CARTESIAN_POINT ( 'NONE',  ( -14.07972454189999922, -80.06168576349999455, 36.83675998920000438 ) ) ;
#14797=CIRCLE ( 'NONE', #2261, 23.36116116979999902 ) ;
#14798=CARTESIAN_POINT ( 'NONE',  ( -21.60034894820000062, -79.50000026560000776, -32.77174736439999947 ) ) ;
#14799=CARTESIAN_POINT ( 'NONE',  ( 22.77479935359999885, -18.50000000000000000, 9.339609977220000303 ) ) ;
#14801=CARTESIAN_POINT ( 'NONE',  ( -20.30440251859999989, -57.41946959940000283, 14.68517168900000058 ) ) ;
#14803=B_SPLINE_CURVE_WITH_KNOTS ( 'NONE', 3,
 ( #11983, #2983, #18710, #14325, #27864, #27607, #12123, #7345, #7911, #814, #23219, #5713, #9799, #2831, #18417, #11844, #21041, #16210, #20603, #1098, #27306, #18852, #27739, #7775, #5156, #16648, #9656, #16365, #9525, #11551, #528, #5312, #14201 ),
 .UNSPECIFIED., .F., .F.,
 ( 4, 2, 2, 1, 1, 1, 2, 2, 2, 1, 1, 1, 2, 2, 2, 1, 1, 1, 2, 2, 4 ),
 ( 0.000000000000000000, 0.1249999999997201128, 0.1874999999995801137, 0.2187499999995101141, 0.2343749999994829691, 0.2421874999994777233, 0.2460937499994894084, 0.2499999999995011213, 0.3749999999996395106, 0.4374999999997140621, 0.4687499999997555844, 0.4843749999997764011, 0.4921874999997811750, 0.4999999999997859490, 0.6249999999997878364, 0.6874999999997887246, 0.7187499999997886135, 0.7343749999997895017, 0.7421874999997863931, 0.7499999999997831734, 1.000000000000000000 ),
 .UNSPECIFIED. ) ;
#14806=CARTESIAN_POINT ( 'NONE',  ( -7.250909741841712552, -73.85719096284161367, 39.82033721815452765 ) ) ;
#14808=EDGE_LOOP ( 'NONE', ( #10957, #4427, #17389, #12845 ) ) ;
#14811=CARTESIAN_POINT ( 'NONE',  ( 36.86771591380000501, -80.05866228240000737, -13.93700013870000021 ) ) ;
#14813=AXIS2_PLACEMENT_3D ( 'NONE', #15518, #11295, #2289 ) ;
#14814=VECTOR ( 'NONE', #16175, 1000.000000000000000 ) ;
#14815=FACE_OUTER_BOUND ( 'NONE', #7569, .T. ) ;
#14818=CARTESIAN_POINT ( 'NONE',  ( 46.34744280896714486, -73.59863498251932867, -3.503223591168824314 ) ) ;
#14821=CARTESIAN_POINT ( 'NONE',  ( 21.71672445076383440, -36.72346566043151483, -8.838003624040505102 ) ) ;
#14822=CARTESIAN_POINT ( 'NONE',  ( -7.135467526410000261, -73.50000000000000000, -38.71641004229999794 ) ) ;
#14823=ORIENTED_EDGE ( 'NONE', *, *, #13200, .F. ) ;
#14824=CARTESIAN_POINT ( 'NONE',  ( 7.066909182079999852, -57.47855601759999900, -22.26662627820000040 ) ) ;
#14825=DIRECTION ( 'NONE',  ( 0.5439177849611214199, 0.000000000000000000, -0.8391385125251892285 ) ) ;
#14826=AXIS2_PLACEMENT_3D ( 'NONE', #138, #8987, #18036 ) ;
#14827=CARTESIAN_POINT ( 'NONE',  ( 22.01683849324958331, -37.96202148674316845, -8.793068656874689637 ) ) ;
#14828=CARTESIAN_POINT ( 'NONE',  ( 19.55470396879999839, -26.09861276219999837, 10.64709123559999959 ) ) ;
#14829=CARTESIAN_POINT ( 'NONE',  ( -0.9583274171050000234, -18.50000000000000000, -21.03286107679999972 ) ) ;
#14830=EDGE_LOOP ( 'NONE', ( #11365, #3766, #5647, #2209 ) ) ;
#14835=CARTESIAN_POINT ( 'NONE',  ( 23.35417726369999869, -57.47855601759999900, -0.5711878298099999363 ) ) ;
#14837=CARTESIAN_POINT ( 'NONE',  ( -2.565902251719999860, -54.99674360790000094, -24.86453770889999859 ) ) ;
#14838=TOROIDAL_SURFACE ( 'NONE', #19955, 3.500000000000000000, 0.5000000000000000000 ) ;
#14839=CARTESIAN_POINT ( 'NONE',  ( -1.521130821679999912, -79.83261741180000115, 47.18112646320000181 ) ) ;
#14840=PLANE ( 'NONE',  #25679 ) ;
#14842=CARTESIAN_POINT ( 'NONE',  ( 40.00000000000000000, -84.50000000000000000, -8.798132407700000305E-16 ) ) ;
#14844=EDGE_CURVE ( 'NONE', #17563, #5033, #28789, .T. ) ;
#14849=CARTESIAN_POINT ( 'NONE',  ( 5.988482279510000053E-15, -69.50000000000000000, 40.00000000000000000 ) ) ;
#14851=ADVANCED_FACE ( 'NONE', ( #4794 ), #2677, .T. ) ;
#14852=AXIS2_PLACEMENT_3D ( 'NONE', #3148, #7530, #16386 ) ;
#14853=VERTEX_POINT ( 'NONE', #13814 ) ;
#14855=ORIENTED_EDGE ( 'NONE', *, *, #9401, .F. ) ;
#14856=CARTESIAN_POINT ( 'NONE',  ( 21.27799938559999759, -36.28875681020000599, -8.154524242129999934 ) ) ;
#14857=CARTESIAN_POINT ( 'NONE',  ( -21.99985828019999801, -74.00000000000000000, -31.89935321680000158 ) ) ;
#14858=ORIENTED_EDGE ( 'NONE', *, *, #1683, .F. ) ;
#14862=CARTESIAN_POINT ( 'NONE',  ( 9.063833271400000058, -53.25913232279999932, -22.59227796120000065 ) ) ;
#14863=ORIENTED_EDGE ( 'NONE', *, *, #14056, .T. ) ;
#14865=CARTESIAN_POINT ( 'NONE',  ( 24.10233903080000317, -34.62274519429999486, 1.400979379020000026 ) ) ;
#14866=CARTESIAN_POINT ( 'NONE',  ( 39.81550290694978855, -73.86170940508526428, 7.247654292427061051 ) ) ;
#14867=ORIENTED_EDGE ( 'NONE', *, *, #7429, .T. ) ;
#14868=CARTESIAN_POINT ( 'NONE',  ( -14.63774944959999935, -74.36723410090000641, 36.92911291229999904 ) ) ;
#14870=CARTESIAN_POINT ( 'NONE',  ( -14.74467115470000067, -74.36322263760000340, 36.36119636340000483 ) ) ;
#14871=CARTESIAN_POINT ( 'NONE',  ( 0.000000000000000000, -84.00000000000000000, -40.00000000000000000 ) ) ;
#14872=DIRECTION ( 'NONE',  ( 1.000000000000000000, 0.000000000000000000, 0.000000000000000000 ) ) ;
#14873=EDGE_LOOP ( 'NONE', ( #28120, #19627, #3798, #9437, #14041, #3474 ) ) ;
#14874=CIRCLE ( 'NONE', #986, 39.25000000000000000 ) ;
#14876=DIRECTION ( 'NONE',  ( 0.000000000000000000, -1.000000000000000000, 0.000000000000000000 ) ) ;
#14878=CARTESIAN_POINT ( 'NONE',  ( 9.246558180430000107, -61.84557969829999990, -23.23378279429999793 ) ) ;
#14879=CARTESIAN_POINT ( 'NONE',  ( -12.80327907979999935, -69.29931929910000576, -23.86045200970000124 ) ) ;
#14880=DIRECTION ( 'NONE',  ( 1.000000000000000000, 0.000000000000000000, 0.000000000000000000 ) ) ;
#14881=CARTESIAN_POINT ( 'NONE',  ( -11.41591306159999952, -19.46348310600000175, -18.84564791440000064 ) ) ;
#14882=ORIENTED_EDGE ( 'NONE', *, *, #19158, .T. ) ;
#14886=EDGE_CURVE ( 'NONE', #14636, #2790, #970, .T. ) ;
#14889=CARTESIAN_POINT ( 'NONE',  ( -12.47194051069999965, -65.04696943620000127, 21.82660845869999733 ) ) ;
#14891=CIRCLE ( 'NONE', #10675, 32.39999999999999858 ) ;
#14893=AXIS2_PLACEMENT_3D ( 'NONE', #9318, #7008, #22601 ) ;
#14897=EDGE_LOOP ( 'NONE', ( #27127, #27368, #19197, #7361, #12138 ) ) ;
#14899=DIRECTION ( 'NONE',  ( 1.000000000000000000, 0.000000000000000000, 0.000000000000000000 ) ) ;
#14900=ORIENTED_EDGE ( 'NONE', *, *, #7512, .F. ) ;
#14904=DIRECTION ( 'NONE',  ( 1.000000000000000000, 0.000000000000000000, 0.000000000000000000 ) ) ;
#14907=DIRECTION ( 'NONE',  ( -0.000000000000000000, 1.000000000000000000, 0.000000000000000000 ) ) ;
#14908=EDGE_CURVE ( 'NONE', #22782, #18665, #26382, .T. ) ;
#14914=CARTESIAN_POINT ( 'NONE',  ( -10.57118441995368130, -18.60777261480114575, -22.16921275799352742 ) ) ;
#14916=B_SPLINE_CURVE_WITH_KNOTS ( 'NONE', 3,
 ( #10699, #4323, #8537, #17442, #8671, #2146 ),
 .UNSPECIFIED., .F., .F.,
 ( 4, 2, 4 ),
 ( 0.000000000000000000, 0.5000000000000000000, 1.000000000000000000 ),
 .UNSPECIFIED. ) ;
#14919=CARTESIAN_POINT ( 'NONE',  ( 22.49121776710000020, -37.66961400949999472, -9.214873578599998893 ) ) ;
#14921=ORIENTED_EDGE ( 'NONE', *, *, #1683, .T. ) ;
#14922=CARTESIAN_POINT ( 'NONE',  ( -1.604812631230000175, -64.93834956060000252, -25.19372014690000228 ) ) ;
#14923=CARTESIAN_POINT ( 'NONE',  ( 10.32053900859999906, -36.18404281990000015, -22.30282316619999960 ) ) ;
#14925=CARTESIAN_POINT ( 'NONE',  ( -11.35954001540000036, -74.50000000000000000, 46.75000000000000000 ) ) ;
#14926=CARTESIAN_POINT ( 'NONE',  ( -32.75000000000000000, -73.50000000000000000, 4.241051954069999455E-15 ) ) ;
#14928=CARTESIAN_POINT ( 'NONE',  ( 21.44331570410000154, -35.78513242900000080, -7.217843123729999810 ) ) ;
#14929=CARTESIAN_POINT ( 'NONE',  ( -12.68423258129978315, -57.45864775708258065, 20.28109956509949896 ) ) ;
#14930=ORIENTED_EDGE ( 'NONE', *, *, #10364, .T. ) ;
#14931=CIRCLE ( 'NONE', #19603, 11.00000000000000000 ) ;
#14932=FACE_OUTER_BOUND ( 'NONE', #504, .T. ) ;
#14933=AXIS2_PLACEMENT_3D ( 'NONE', #22119, #13658, #17598 ) ;
#14934=CARTESIAN_POINT ( 'NONE',  ( -17.58882677589999943, -18.50000000000000000, 13.37910508939999943 ) ) ;
#14936=CARTESIAN_POINT ( 'NONE',  ( -32.48620205747189971, -74.10974938391861144, -22.14461327791768142 ) ) ;
#14937=CARTESIAN_POINT ( 'NONE',  ( -19.79578083020000179, -57.47815899190000266, 12.40825019989999767 ) ) ;
#14939=DIRECTION ( 'NONE',  ( 0.2414462220490750377, 0.000000000000000000, -0.9704142011833034598 ) ) ;
#14944=ADVANCED_FACE ( 'NONE', ( #9438 ), #9725, .T. ) ;
#14946=CARTESIAN_POINT ( 'NONE',  ( -14.93121066289999987, -74.50000000000000000, 36.29905574720000061 ) ) ;
#14947=CARTESIAN_POINT ( 'NONE',  ( -32.09407551019999971, -74.00665451570000641, -22.04839896869999905 ) ) ;
#14948=CARTESIAN_POINT ( 'NONE',  ( 7.627568735119999666, -74.00000000000000000, 38.62788659690000515 ) ) ;
#14949=ORIENTED_EDGE ( 'NONE', *, *, #23358, .F. ) ;
#14951=TOROIDAL_SURFACE ( 'NONE', #3366, 3.750000000000000000, 1.000000000000000000 ) ;
#14953=CARTESIAN_POINT ( 'NONE',  ( -2.658799883775093686, -80.38812240490400995, 46.74488113567394976 ) ) ;
#14954=VERTEX_POINT ( 'NONE', #20680 ) ;
#14955=CYLINDRICAL_SURFACE ( 'NONE', #2096, 7.249999999999999112 ) ;
#14958=CARTESIAN_POINT ( 'NONE',  ( 0.000000000000000000, -89.50000000000000000, 0.000000000000000000 ) ) ;
#14959=CARTESIAN_POINT ( 'NONE',  ( -7.219524535890000649, -73.62955962630000784, -39.18053445169999804 ) ) ;
#14960=VERTEX_POINT ( 'NONE', #11918 ) ;
#14962=CARTESIAN_POINT ( 'NONE',  ( -3.610293368829999849, -18.50000000000000000, -24.43613445369999937 ) ) ;
#14964=CARTESIAN_POINT ( 'NONE',  ( 9.510883186780000997, -36.00000000010000178, -20.82957718990000018 ) ) ;
#14966=CIRCLE ( 'NONE', #1984, 4.750000000000000888 ) ;
#14967=CARTESIAN_POINT ( 'NONE',  ( -1.776356839399999804E-15, -79.50000000000000000, 47.25000000000000000 ) ) ;
#14968=EDGE_LOOP ( 'NONE', ( #13435, #15285, #1319 ) ) ;
#14973=CARTESIAN_POINT ( 'NONE',  ( -2.360777964760000458, -53.80651132049999319, -24.23647548509999794 ) ) ;
#14982=CARTESIAN_POINT ( 'NONE',  ( -14.48905496503022583, -70.53876985267483235, 23.53798342341141492 ) ) ;
#14987=CARTESIAN_POINT ( 'NONE',  ( -6.705637591229999472, -74.00000000000000000, 35.51864961870000315 ) ) ;
#14988=CARTESIAN_POINT ( 'NONE',  ( 20.69709980620000067, -35.75422006420000542, -8.773405848899999526 ) ) ;
#14990=CARTESIAN_POINT ( 'NONE',  ( 20.16934030379999854, -35.86380921170000136, -9.031588964350000026 ) ) ;
#14991=DIRECTION ( 'NONE',  ( 0.000000000000000000, 1.000000000000000000, 0.000000000000000000 ) ) ;
#14992=VERTEX_POINT ( 'NONE', #26435 ) ;
#14996=DIRECTION ( 'NONE',  ( 0.000000000000000000, -1.000000000000000000, 0.000000000000000000 ) ) ;
#15001=CARTESIAN_POINT ( 'NONE',  ( 22.27593118400000094, -19.46147658920000012, 0.5502460698960000007 ) ) ;
#15002=CARTESIAN_POINT ( 'NONE',  ( 24.87884979860000101, -67.58705842039999823, 10.90550133649999864 ) ) ;
#15004=ORIENTED_EDGE ( 'NONE', *, *, #8663, .T. ) ;
#15005=CARTESIAN_POINT ( 'NONE',  ( -40.28432270880000488, -74.37142462010000088, 7.256994698139999755 ) ) ;
#15006=EDGE_CURVE ( 'NONE', #4268, #28156, #22801, .T. ) ;
#15008=DIRECTION ( 'NONE',  ( 1.000000000000000000, 0.000000000000000000, 0.000000000000000000 ) ) ;
#15011=ORIENTED_EDGE ( 'NONE', *, *, #23622, .F. ) ;
#15012=CARTESIAN_POINT ( 'NONE',  ( 26.61465533970000052, -68.28989644159999273, 0.1578866888799999868 ) ) ;
#15014=CARTESIAN_POINT ( 'NONE',  ( 9.111815586569999681, -58.91975330950000256, -22.76485177850000241 ) ) ;
#15015=CARTESIAN_POINT ( 'NONE',  ( -13.17060624760000032, -68.28989248250000799, -23.12789913420000332 ) ) ;
#15016=CARTESIAN_POINT ( 'NONE',  ( 20.64374742240000060, -57.47815889169999792, 10.93951826979999886 ) ) ;
#15018=ORIENTED_EDGE ( 'NONE', *, *, #13648, .F. ) ;
#15024=B_SPLINE_CURVE_WITH_KNOTS ( 'NONE', 5,
 ( #11045, #19961, #24490, #24793, #9176, #27126, #15434, #9478, #17940 ),
 .UNSPECIFIED., .F., .F.,
 ( 6, 3, 6 ),
 ( 0.000000000000000000, 0.3290135943971881360, 1.000000000000000000 ),
 .UNSPECIFIED. ) ;
#15026=ORIENTED_EDGE ( 'NONE', *, *, #13684, .T. ) ;
#15033=DIRECTION ( 'NONE',  ( -7.486357007659999211E-17, 0.000000000000000000, 1.000000000000000000 ) ) ;
#15036=EDGE_CURVE ( 'NONE', #20989, #24745, #24661, .T. ) ;
#15037=DIRECTION ( 'NONE',  ( 0.000000000000000000, -1.000000000000000000, 0.000000000000000000 ) ) ;
#15041=VECTOR ( 'NONE', #9916, 1000.000000000000000 ) ;
#15044=CIRCLE ( 'NONE', #7187, 2.000000000000000888 ) ;
#15046=DIRECTION ( 'NONE',  ( -1.000000000000000000, 0.000000000000000000, -1.224606353820000075E-16 ) ) ;
#15048=CARTESIAN_POINT ( 'NONE',  ( 19.24256498990000352, -18.50000000000000000, -7.923762209979999582 ) ) ;
#15049=ADVANCED_FACE ( 'NONE', ( #12196 ), #26499, .F. ) ;
#15050=FACE_OUTER_BOUND ( 'NONE', #6876, .T. ) ;
#15052=CARTESIAN_POINT ( 'NONE',  ( -18.82843809638912447, -19.48034373446246548, 13.69127826824404615 ) ) ;
#15054=CARTESIAN_POINT ( 'NONE',  ( 7.506539852059999518, -35.02344201600000417, -21.30237675789999940 ) ) ;
#15055=CARTESIAN_POINT ( 'NONE',  ( -19.73459501710000197, -19.50000000000000000, 14.41863426819999994 ) ) ;
#15056=ORIENTED_EDGE ( 'NONE', *, *, #11125, .T. ) ;
#15057=CARTESIAN_POINT ( 'NONE',  ( 7.780770465739999864, -18.50000000000000000, -19.47999901649999543 ) ) ;
#15058=CARTESIAN_POINT ( 'NONE',  ( 22.72952646779999952, -37.67772343429999893, -9.324355546680001439 ) ) ;
#15059=CARTESIAN_POINT ( 'NONE',  ( -1.195589003429999853, -62.93490527480000196, -24.29973956710000138 ) ) ;
#15061=CARTESIAN_POINT ( 'NONE',  ( 10.88627897289999957, -36.00000000000000000, -22.06017285100000080 ) ) ;
#15063=CARTESIAN_POINT ( 'NONE',  ( -19.80901448590000058, -53.80651132049999319, 14.16273143270000112 ) ) ;
#15067=EDGE_LOOP ( 'NONE', ( #16844, #27803, #2449, #1643 ) ) ;
#15070=ORIENTED_EDGE ( 'NONE', *, *, #22012, .T. ) ;
#15072=CARTESIAN_POINT ( 'NONE',  ( -37.29988270759999835, -74.00000000000000000, -26.69328098980000163 ) ) ;
#15073=AXIS2_PLACEMENT_3D ( 'NONE', #26128, #28445, #16961 ) ;
#15074=CARTESIAN_POINT ( 'NONE',  ( 40.70731707320000226, -74.50000000000000000, 7.215414233289999757 ) ) ;
#15075=ADVANCED_FACE ( 'NONE', ( #2551 ), #15926, .F. ) ;
#15076=CARTESIAN_POINT ( 'NONE',  ( 22.32094435669999655, -18.62259217289999924, 9.382461709760001156 ) ) ;
#15077=CARTESIAN_POINT ( 'NONE',  ( -32.71776494810505653, -74.25643782585186159, -22.20071764928750468 ) ) ;
#15079=VERTEX_POINT ( 'NONE', #9522 ) ;
#15081=CARTESIAN_POINT ( 'NONE',  ( -36.23922253580000330, -80.00000000000000000, -26.33972759919999973 ) ) ;
#15083=CARTESIAN_POINT ( 'NONE',  ( 1.678657213230000024E-14, -74.00000000000000000, 7.838174553849999450E-15 ) ) ;
#15087=CARTESIAN_POINT ( 'NONE',  ( -22.59314464595784955, -79.98715482475118677, -32.67653664314131845 ) ) ;
#15089=AXIS2_PLACEMENT_3D ( 'NONE', #16634, #7189, #18695 ) ;
#15091=CARTESIAN_POINT ( 'NONE',  ( 27.49607050420000220, -67.46050995630001523, 1.934818144049999855 ) ) ;
#15093=CARTESIAN_POINT ( 'NONE',  ( -12.47289874709933244, -69.87861895799714773, -24.46965691794827791 ) ) ;
#15096=CARTESIAN_POINT ( 'NONE',  ( 46.12101806169999918, -73.64067649049998465, -3.912894910599999942 ) ) ;
#15097=ORIENTED_EDGE ( 'NONE', *, *, #1032, .F. ) ;
#15098=DIRECTION ( 'NONE',  ( 0.000000000000000000, -1.000000000000000000, 0.000000000000000000 ) ) ;
#15099=CARTESIAN_POINT ( 'NONE',  ( 19.54737287369999876, -35.65078480380000059, -9.004240688089998557 ) ) ;
#15104=CARTESIAN_POINT ( 'NONE',  ( 4.426600958609999879E-15, -84.50000000000000000, 43.75000000000000000 ) ) ;
#15108=DIRECTION ( 'NONE',  ( 0.000000000000000000, -1.000000000000000000, 0.000000000000000000 ) ) ;
#15109=FACE_OUTER_BOUND ( 'NONE', #4235, .T. ) ;
#15111=CARTESIAN_POINT ( 'NONE',  ( -2.572593885869999930, -45.95049971630000130, -24.95132982360000184 ) ) ;
#15113=DIRECTION ( 'NONE',  ( 0.000000000000000000, -1.000000000000000000, 0.000000000000000000 ) ) ;
#15118=CARTESIAN_POINT ( 'NONE',  ( -40.00000000000000000, -69.50000000000000000, 2.464695114669999848E-15 ) ) ;
#15119=ADVANCED_FACE ( 'NONE', ( #4869 ), #525, .T. ) ;
#15121=CARTESIAN_POINT ( 'NONE',  ( -11.35954001540000036, -79.50000000000000000, 46.75000000000000000 ) ) ;
#15127=CARTESIAN_POINT ( 'NONE',  ( 21.43682400119999798, -36.68968512050000186, -8.001561263239999278 ) ) ;
#15130=EDGE_LOOP ( 'NONE', ( #25173, #28661, #18209, #16445, #2934 ) ) ;
#15133=CARTESIAN_POINT ( 'NONE',  ( -3.105596691226790274, -66.68383445268185028, -27.13055080113027628 ) ) ;
#15134=DIRECTION ( 'NONE',  ( 0.3687499999999814260, 0.000000000000000000, -0.9295286103719527793 ) ) ;
#15135=CARTESIAN_POINT ( 'NONE',  ( -13.17786140689999819, -69.76368794990000310, -23.89400643789999990 ) ) ;
#15137=CARTESIAN_POINT ( 'NONE',  ( -10.93050817210000147, -18.61782386119999799, -18.68920581670000303 ) ) ;
#15140=ORIENTED_EDGE ( 'NONE', *, *, #5783, .F. ) ;
#15141=DIRECTION ( 'NONE',  ( 0.000000000000000000, -1.000000000000000000, 0.000000000000000000 ) ) ;
#15142=CARTESIAN_POINT ( 'NONE',  ( 24.95344409500000182, -42.20269670429999564, 1.384270800949999991 ) ) ;
#15143=CARTESIAN_POINT ( 'NONE',  ( 24.47298445130000033, -67.79480919600000277, 11.04024604620000005 ) ) ;
#15145=ORIENTED_EDGE ( 'NONE', *, *, #11672, .T. ) ;
#15146=CARTESIAN_POINT ( 'NONE',  ( -38.68350751799999898, -73.93831497249999529, 7.318372426699999878 ) ) ;
#15147=CARTESIAN_POINT ( 'NONE',  ( -10.20110288159999890, -74.50000000000000000, -41.00000000000000000 ) ) ;
#15149=DIRECTION ( 'NONE',  ( 1.000000000000000000, 0.000000000000000000, 0.000000000000000000 ) ) ;
#15151=CARTESIAN_POINT ( 'NONE',  ( -38.62788659690000515, -74.00000000000000000, 7.627568735119999666 ) ) ;
#15153=CARTESIAN_POINT ( 'NONE',  ( 8.756289919979998615, -61.98517989029999598, -22.88741420530000070 ) ) ;
#15155=CARTESIAN_POINT ( 'NONE',  ( 20.87897399470000082, -58.35063071660000134, 10.71952971249999997 ) ) ;
#15156=CARTESIAN_POINT ( 'NONE',  ( -11.46863446409999909, -57.40875703270000230, -22.62382275130000053 ) ) ;
#15158=ADVANCED_FACE ( 'NONE', ( #18859 ), #819, .T. ) ;
#15161=ORIENTED_EDGE ( 'NONE', *, *, #1413, .T. ) ;
#15163=CARTESIAN_POINT ( 'NONE',  ( 21.05681896020000110, -18.50000000000000000, -0.02359534709730000054 ) ) ;
#15164=ADVANCED_FACE ( 'NONE', ( #12130, #28016 ), #21312, .T. ) ;
#15166=ORIENTED_EDGE ( 'NONE', *, *, #3216, .F. ) ;
#15168=B_SPLINE_SURFACE_WITH_KNOTS ( 'NONE', 5, 5, ( 
 ( #1788, #12407, #6287, #12546, #1657, #10632, #10359, #23786, #14614 ),
 ( #28160, #21319, #5997, #25842, #5864, #28289, #8321, #12972, #1375 ),
 ( #19546, #10222, #19134, #14878, #15153, #3825, #8061, #24063, #4102 ),
 ( #3966, #8193, #21885, #28434, #16951, #1936, #3683, #21461, #1515 ),
 ( #17223, #26114, #6141, #15014, #23928, #8468, #49, #28578, #22477 ),
 ( #17663, #8894, #9190, #4689, #19688, #26547, #4251, #20130, #2083 ) ),
 .UNSPECIFIED., .F., .F., .F.,
 ( 6, 6 ),
 ( 6, 3, 6 ),
 ( 54.79316133020000024, 65.31895168009999963 ),
 ( 0.000000000000000000, 1.000000000000000000, 2.000000000000000000 ),
 .UNSPECIFIED. ) ;
#15171=PRESENTATION_STYLE_ASSIGNMENT (( #12425 ) ) ;
#15173=ORIENTED_EDGE ( 'NONE', *, *, #7173, .T. ) ;
#15177=FACE_OUTER_BOUND ( 'NONE', #9609, .T. ) ;
#15178=CARTESIAN_POINT ( 'NONE',  ( 23.71521856880000101, -60.21977178070000036, -9.629174062080000596 ) ) ;
#15180=DIRECTION ( 'NONE',  ( 0.9382669785645009197, 0.000000000000000000, -0.3459119496858159559 ) ) ;
#15181=CARTESIAN_POINT ( 'NONE',  ( 18.85230044170000241, -18.50000000000000000, -8.028472989549999994 ) ) ;
#15185=CARTESIAN_POINT ( 'NONE',  ( 7.923301502570000210, -34.91901258349999893, -21.18066442289999785 ) ) ;
#15186=DIRECTION ( 'NONE',  ( 0.000000000000000000, 1.000000000000000000, 0.000000000000000000 ) ) ;
#15193=EDGE_LOOP ( 'NONE', ( #1991, #5750, #9044, #22531 ) ) ;
#15194=CARTESIAN_POINT ( 'NONE',  ( -0.5459402786740000790, -58.79569603810000444, -23.43709083150000083 ) ) ;
#15199=CARTESIAN_POINT ( 'NONE',  ( -19.96385611919999903, -52.58489974430013802, 14.40794232450000045 ) ) ;
#15204=CARTESIAN_POINT ( 'NONE',  ( 21.29161486119999580, -35.09212000590000002, -7.585065879760000129 ) ) ;
#15206=CARTESIAN_POINT ( 'NONE',  ( 7.256982118339999843, -74.37144044059999715, -40.28438195579999359 ) ) ;
#15210=CARTESIAN_POINT ( 'NONE',  ( -9.593141833260000695, -18.50000000000000000, -19.59102626760000376 ) ) ;
#15211=AXIS2_PLACEMENT_3D ( 'NONE', #133, #2302, #4035 ) ;
#15212=CARTESIAN_POINT ( 'NONE',  ( 20.87089110420000182, -18.61940624680000056, 9.000567795900000334 ) ) ;
#15213=DIRECTION ( 'NONE',  ( 1.000000000000000000, 0.000000000000000000, 0.000000000000000000 ) ) ;
#15218=CARTESIAN_POINT ( 'NONE',  ( -7.197231212906468834, -73.55557714109660594, 39.12476203138809439 ) ) ;
#15220=ORIENTED_EDGE ( 'NONE', *, *, #27116, .F. ) ;
#15222=AXIS2_PLACEMENT_3D ( 'NONE', #17519, #6593, #4544 ) ;
#15223=CARTESIAN_POINT ( 'NONE',  ( -32.32657687519999712, -74.05570514439999386, -21.80503578329999925 ) ) ;
#15224=FACE_OUTER_BOUND ( 'NONE', #26888, .T. ) ;
#15227=CARTESIAN_POINT ( 'NONE',  ( 19.54973049059999823, -35.76277645470000266, -9.056828148970000214 ) ) ;
#15228=CARTESIAN_POINT ( 'NONE',  ( -22.53893512686634537, -80.06168502835437550, -32.36019063177454314 ) ) ;
#15229=EDGE_CURVE ( 'NONE', #10466, #14636, #13944, .T. ) ;
#15230=EDGE_LOOP ( 'NONE', ( #6564, #10701, #18593, #15018 ) ) ;
#15231=CIRCLE ( 'NONE', #4088, 11.00000000000000000 ) ;
#15233=FACE_OUTER_BOUND ( 'NONE', #10892, .T. ) ;
#15234=ORIENTED_EDGE ( 'NONE', *, *, #9895, .F. ) ;
#15236=CARTESIAN_POINT ( 'NONE',  ( 46.33376634150000228, -73.97423400449999065, -4.091715457210000295 ) ) ;
#15239=DIRECTION ( 'NONE',  ( 0.000000000000000000, -1.000000000000000000, 0.000000000000000000 ) ) ;
#15241=CARTESIAN_POINT ( 'NONE',  ( 8.637923669450000119, -37.95659433029999974, -21.89902260000000211 ) ) ;
#15243=CARTESIAN_POINT ( 'NONE',  ( -3.383950074269999941, -18.50000000000000000, -22.79034367919999937 ) ) ;
#15244=VERTEX_POINT ( 'NONE', #4922 ) ;
#15245=CARTESIAN_POINT ( 'NONE',  ( -26.69328098980000163, -80.00000000000000000, -35.88566914520000495 ) ) ;
#15247=CARTESIAN_POINT ( 'NONE',  ( 23.61566649627895487, -60.59571579695727195, -0.5691236615726964487 ) ) ;
#15249=CARTESIAN_POINT ( 'NONE',  ( 27.49607050420000220, -67.46050995630001523, 1.934818144049999855 ) ) ;
#15251=DIRECTION ( 'NONE',  ( 0.000000000000000000, -1.000000000000000000, 0.000000000000000000 ) ) ;
#15253=VECTOR ( 'NONE', #4575, 1000.000000000000000 ) ;
#15254=CARTESIAN_POINT ( 'NONE',  ( 10.08508256729999886, -64.24504434620000382, -24.78974309399999854 ) ) ;
#15259=DIRECTION ( 'NONE',  ( 1.000000000000000000, 0.000000000000000000, 0.000000000000000000 ) ) ;
#15264=CARTESIAN_POINT ( 'NONE',  ( 7.120909764619999412E-15, -73.00000000000000000, 40.00000000000000000 ) ) ;
#15265=EDGE_CURVE ( 'NONE', #8148, #23453, #14567, .T. ) ;
#15266=ORIENTED_EDGE ( 'NONE', *, *, #2484, .F. ) ;
#15269=CARTESIAN_POINT ( 'NONE',  ( 20.42801697140000172, -35.85629042629999219, -8.882126403010001781 ) ) ;
#15270=CARTESIAN_POINT ( 'NONE',  ( 7.685455900877268931, -18.85523520683459964, -20.50116745598906220 ) ) ;
#15271=ORIENTED_EDGE ( 'NONE', *, *, #18934, .T. ) ;
#15273=CIRCLE ( 'NONE', #24635, 7.250000000000000000 ) ;
#15274=AXIS2_PLACEMENT_3D ( 'NONE', #18450, #7377, #16241 ) ;
#15276=DIRECTION ( 'NONE',  ( 0.7071067811865475727, 0.000000000000000000, -0.7071067811865475727 ) ) ;
#15282=CARTESIAN_POINT ( 'NONE',  ( 23.04132486059999962, -42.26701801500000499, 0.3804478350989999869 ) ) ;
#15283=CARTESIAN_POINT ( 'NONE',  ( 23.84115441240000166, -68.12125821070000598, 11.66698334899999878 ) ) ;
#15284=CARTESIAN_POINT ( 'NONE',  ( 39.13694367177480160, -73.55869875168333749, 7.198781031945556741 ) ) ;
#15285=ORIENTED_EDGE ( 'NONE', *, *, #5714, .F. ) ;
#15288=CARTESIAN_POINT ( 'NONE',  ( 0.000000000000000000, -77.00000000000000000, -40.00000000000000000 ) ) ;
#15289=ORIENTED_EDGE ( 'NONE', *, *, #16657, .F. ) ;
#15291=CIRCLE ( 'NONE', #2785, 1.999999999999998224 ) ;
#15293=CARTESIAN_POINT ( 'NONE',  ( 24.55236475814571406, -74.19409854689706663, -30.49148208431322971 ) ) ;
#15294=CARTESIAN_POINT ( 'NONE',  ( -41.00000000000000000, -74.50000000000000000, -10.20110288159999890 ) ) ;
#15296=CARTESIAN_POINT ( 'NONE',  ( -11.07869211709999924, -49.85663837269999732, -20.93251907349999641 ) ) ;
#15298=AXIS2_PLACEMENT_3D ( 'NONE', #5604, #17092, #7932 ) ;
#15306=ORIENTED_EDGE ( 'NONE', *, *, #4377, .F. ) ;
#15308=CARTESIAN_POINT ( 'NONE',  ( 22.97338017759999929, -18.50000000000000000, 2.313460506620000245 ) ) ;
#15311=CARTESIAN_POINT ( 'NONE',  ( 19.82451678549999841, -19.46527880160000024, -8.815774675060000121 ) ) ;
#15312=CARTESIAN_POINT ( 'NONE',  ( -7.318372426699999878, -73.93831497249999529, -38.68350751799999898 ) ) ;
#15314=ORIENTED_EDGE ( 'NONE', *, *, #21014, .T. ) ;
#15315=CARTESIAN_POINT ( 'NONE',  ( 27.26688910437447433, -72.05982473802319532, -11.73839635661862779 ) ) ;
#15317=ORIENTED_EDGE ( 'NONE', *, *, #21706, .T. ) ;
#15318=FACE_OUTER_BOUND ( 'NONE', #10990, .T. ) ;
#15320=CONICAL_SURFACE ( 'NONE', #27483, 21.99999999999999645, 0.03490658503990158590 ) ;
#15321=AXIS2_PLACEMENT_3D ( 'NONE', #16272, #12043, #25609 ) ;
#15324=CARTESIAN_POINT ( 'NONE',  ( 22.85308509809999933, -18.50000000000000000, 2.011281980869999764 ) ) ;
#15325=DIRECTION ( 'NONE',  ( 0.000000000000000000, -1.000000000000000000, 0.000000000000000000 ) ) ;
#15327=VERTEX_POINT ( 'NONE', #22999 ) ;
#15329=CARTESIAN_POINT ( 'NONE',  ( -13.60716892229999964, -18.50000000000000000, 19.16900036430000043 ) ) ;
#15331=B_SPLINE_CURVE_WITH_KNOTS ( 'NONE', 3,
 ( #9351, #1087, #20742, #13730, #9639, #18253, #25261, #18546, #27442, #14177, #23071, #3116, #11968, #20886, #10597, #8033, #8438, #5968, #23757, #21163, #5702, #27850, #14584, #23486, #23343, #18970, #10465, #7900, #16777, #6112, #3799, #23615 ),
 .UNSPECIFIED., .F., .F.,
 ( 4, 2, 1, 1, 1, 2, 2, 2, 1, 1, 1, 2, 2, 2, 1, 1, 1, 1, 2, 2, 4 ),
 ( 0.000000000000000000, 0.1249999999999596434, 0.1874999999999354128, 0.2187499999999232558, 0.2343749999999195366, 0.2421874999999176770, 0.2499999999999158173, 0.3749999999999181211, 0.4374999999999232281, 0.4687499999999258371, 0.4843749999999192868, 0.4921874999999237277, 0.4999999999999282796, 0.6249999999999982236, 0.6875000000000333067, 0.7187500000000596190, 0.7343750000000742739, 0.7421875000000782707, 0.7460937500000784928, 0.7500000000000788258, 1.000000000000000000 ),
 .UNSPECIFIED. ) ;
#15333=CARTESIAN_POINT ( 'NONE',  ( -12.02996277529999958, -67.03347986180000362, -24.13052248920000054 ) ) ;
#15334=FACE_OUTER_BOUND ( 'NONE', #6064, .T. ) ;
#15335=CARTESIAN_POINT ( 'NONE',  ( 7.585065630090000788, -35.09211962219999492, -21.29161487800000074 ) ) ;
#15338=CARTESIAN_POINT ( 'NONE',  ( -10.37349633357829148, -18.49999964046208945, -22.33837851017446852 ) ) ;
#15341=AXIS2_PLACEMENT_3D ( 'NONE', #9508, #18411, #27299 ) ;
#15344=CARTESIAN_POINT ( 'NONE',  ( -13.85849003780000110, -57.40875665010000262, 21.24403944460000204 ) ) ;
#15346=CARTESIAN_POINT ( 'NONE',  ( -19.57724474209999954, -53.84184168659999870, 12.63913840070000028 ) ) ;
#15347=FACE_OUTER_BOUND ( 'NONE', #5812, .T. ) ;
#15350=CARTESIAN_POINT ( 'NONE',  ( 21.45961748159999871, -35.74888769769999897, -7.120077148630000075 ) ) ;
#15351=CARTESIAN_POINT ( 'NONE',  ( 7.440489808669999761, -74.12477399289998914, -39.45579440659999904 ) ) ;
#15352=VERTEX_POINT ( 'NONE', #25466 ) ;
#15353=CARTESIAN_POINT ( 'NONE',  ( -10.20110288159999890, -74.00000000000000000, 41.00000000000000000 ) ) ;
#15355=ADVANCED_FACE ( 'NONE', ( #25333 ), #9291, .T. ) ;
#15356=CARTESIAN_POINT ( 'NONE',  ( 19.94171510720000029, -39.36519097769999576, 10.90497833400000083 ) ) ;
#15359=AXIS2_PLACEMENT_3D ( 'NONE', #18656, #25364, #27254 ) ;
#15360=EDGE_CURVE ( 'NONE', #2790, #27403, #6197, .T. ) ;
#15364=CARTESIAN_POINT ( 'NONE',  ( 19.97576656849999921, -36.00000000000000000, -19.97576656849999921 ) ) ;
#15366=FACE_OUTER_BOUND ( 'NONE', #3811, .T. ) ;
#15369=CARTESIAN_POINT ( 'NONE',  ( -7.218759893172350672, -73.62114148037002792, 39.32637163715104833 ) ) ;
#15370=CARTESIAN_POINT ( 'NONE',  ( -40.70731707320000226, -74.50000000000000000, -7.215414233289999757 ) ) ;
#15372=ADVANCED_FACE ( 'NONE', ( #21101 ), #13000, .F. ) ;
#15373=FACE_OUTER_BOUND ( 'NONE', #9054, .T. ) ;
#15374=CARTESIAN_POINT ( 'NONE',  ( -22.22906643760000023, -79.50000000000000000, -32.83566815539999340 ) ) ;
#15376=DIRECTION ( 'NONE',  ( 1.000000000000000000, 0.000000000000000000, 0.000000000000000000 ) ) ;
#15381=ORIENTED_EDGE ( 'NONE', *, *, #26512, .T. ) ;
#15382=AXIS2_PLACEMENT_3D ( 'NONE', #23033, #25365, #11637 ) ;
#15384=ORIENTED_EDGE ( 'NONE', *, *, #3504, .F. ) ;
#15387=ORIENTED_EDGE ( 'NONE', *, *, #28312, .F. ) ;
#15403=ADVANCED_FACE ( 'NONE', ( #5218 ), #7831, .F. ) ;
#15404=TOROIDAL_SURFACE ( 'NONE', #9380, 30.50381168839999901, 2.000000000000000000 ) ;
#15405=CARTESIAN_POINT ( 'NONE',  ( 6.717799458580000049, -84.50000000000000000, -40.65853658540000026 ) ) ;
#15406=CARTESIAN_POINT ( 'NONE',  ( -18.03086174180000256, -18.61827554290000108, 12.74382289080000064 ) ) ;
#15408=VECTOR ( 'NONE', #2186, 1000.000000000000114 ) ;
#15411=CARTESIAN_POINT ( 'NONE',  ( 9.099148368520435071, -57.44066836785145114, -22.71963871380157585 ) ) ;
#15413=CARTESIAN_POINT ( 'NONE',  ( 22.04985193179999925, -18.50000000000000000, 8.586826782579999318 ) ) ;
#15414=CYLINDRICAL_SURFACE ( 'NONE', #10341, 7.250000000000004441 ) ;
#15422=ORIENTED_EDGE ( 'NONE', *, *, #11303, .T. ) ;
#15423=CARTESIAN_POINT ( 'NONE',  ( -13.46276276162894625, -19.23820061190542319, 20.39865906485581704 ) ) ;
#15424=DIRECTION ( 'NONE',  ( 1.000000000000000000, 0.000000000000000000, 0.000000000000000000 ) ) ;
#15433=CARTESIAN_POINT ( 'NONE',  ( -10.73461461720000010, -18.50000000000000000, -18.44891755279999757 ) ) ;
#15434=CARTESIAN_POINT ( 'NONE',  ( 25.04292896270000313, -70.80052042889998631, 11.98325363630000062 ) ) ;
#15436=ADVANCED_FACE ( 'NONE', ( #25749 ), #21367, .T. ) ;
#15438=CARTESIAN_POINT ( 'NONE',  ( 24.82569795559999903, -49.81670839440000265, 1.385523269080000119 ) ) ;
#15439=CARTESIAN_POINT ( 'NONE',  ( 23.84247938200000050, -66.23852357979998828, 10.90989094220000055 ) ) ;
#15442=DIRECTION ( 'NONE',  ( 0.000000000000000000, 1.000000000000000000, 0.000000000000000000 ) ) ;
#15444=CARTESIAN_POINT ( 'NONE',  ( -40.00000000000000000, -74.00000000000000000, 3.466919520389999841E-15 ) ) ;
#15446=ADVANCED_FACE ( 'NONE', ( #26172, #6340 ), #23693, .T. ) ;
#15447=CARTESIAN_POINT ( 'NONE',  ( 27.57043804909999807, -69.70329313409999372, 1.768595993289999946 ) ) ;
#15450=DIRECTION ( 'NONE',  ( 0.09756097560976997873, 0.000000000000000000, -0.9952295494196653491 ) ) ;
#15451=CARTESIAN_POINT ( 'NONE',  ( -12.41806785860000062, -68.06111301600000729, -23.59935346929999866 ) ) ;
#15454=CARTESIAN_POINT ( 'NONE',  ( 28.31887119405866216, -72.09394576601212634, 1.343104835225076066 ) ) ;
#15455=FACE_OUTER_BOUND ( 'NONE', #8312, .T. ) ;
#15460=EDGE_LOOP ( 'NONE', ( #19485, #22565, #15834 ) ) ;
#15463=VERTEX_POINT ( 'NONE', #10683 ) ;
#15464=CARTESIAN_POINT ( 'NONE',  ( 26.81987566912476240, -72.54457018766687781, -10.76610228402119773 ) ) ;
#15465=VECTOR ( 'NONE', #9169, 1000.000000000000000 ) ;
#15469=CARTESIAN_POINT ( 'NONE',  ( 9.067969494719999801, -35.79825198000000341, -19.85338805880000024 ) ) ;
#15470=AXIS2_PLACEMENT_3D ( 'NONE', #6611, #10802, #17535 ) ;
#15474=FACE_OUTER_BOUND ( 'NONE', #8205, .T. ) ;
#15475=CARTESIAN_POINT ( 'NONE',  ( -38.71641001238787538, -73.63089972761061119, -7.135467692469587675 ) ) ;
#15479=CARTESIAN_POINT ( 'NONE',  ( 28.70651795192725686, -71.31133772027507689, 2.849249339242819090 ) ) ;
#15481=EDGE_CURVE ( 'NONE', #20759, #26341, #26458, .T. ) ;
#15483=B_SPLINE_SURFACE_WITH_KNOTS ( 'NONE', 5, 5, ( 
 ( #560, #9404, #24274, #26611, #19893, #4313 ),
 ( #22097, #8812, #11290, #2285, #20050, #113 ),
 ( #20197, #27870, #1236, #1651, #7240, #21184 ),
 ( #10487, #12683, #16802, #23637, #10353, #11733 ),
 ( #3676, #16253, #27342, #14738, #7917, #25006 ),
 ( #707, #5196, #5041, #9559, #23778, #25695 ),
 ( #5722, #22832, #10075, #16106, #13931, #25835 ),
 ( #1510, #14604, #5990, #23509, #3546, #21592 ),
 ( #5857, #14870, #25966, #19264, #28153, #12537 ),
 ( #2877, #21455, #12401, #19400, #18990, #20649 ),
 ( #23365, #21313, #8186, #3819, #18458, #1367 ),
 ( #7388, #25163, #3409, #14078, #12274, #10214 ) ),
 .UNSPECIFIED., .F., .F., .F.,
 ( 6, 3, 3, 6 ),
 ( 6, 6 ),
 ( 1.565586965149999839E-10, 0.8942904027689999591, 1.389395125490000105, 1.857837794129999942 ),
 ( 0.000000000000000000, 0.5000000000000000000 ),
 .UNSPECIFIED. ) ;
#15484=AXIS2_PLACEMENT_3D ( 'NONE', #1379, #10225, #28026 ) ;
#15486=CARTESIAN_POINT ( 'NONE',  ( -12.07244877390000148, -67.46051290640001241, -24.77968394139999830 ) ) ;
#15493=TOROIDAL_SURFACE ( 'NONE', #24354, 38.75000000000000000, 0.5000000000000000000 ) ;
#15495=ADVANCED_FACE ( 'NONE', ( #10537 ), #7336, .T. ) ;
#15496=CARTESIAN_POINT ( 'NONE',  ( -13.70187040939999967, -57.41946935120000006, 20.98050596210000052 ) ) ;
#15497=CARTESIAN_POINT ( 'NONE',  ( -1.347567224549999887, -65.01950563030000296, -25.09408215860000269 ) ) ;
#15499=CARTESIAN_POINT ( 'NONE',  ( -20.08102625940000507, -57.43018266629999857, 14.46712152350000125 ) ) ;
#15503=VECTOR ( 'NONE', #404, 1000.000000000000000 ) ;
#15508=EDGE_CURVE ( 'NONE', #5350, #20540, #3728, .T. ) ;
#15510=CARTESIAN_POINT ( 'NONE',  ( 22.61645189879999762, -32.66150190460000147, 10.07608658779999899 ) ) ;
#15514=CARTESIAN_POINT ( 'NONE',  ( 19.45586016849999922, -18.85467989400000022, 10.05010111100000003 ) ) ;
#15515=CARTESIAN_POINT ( 'NONE',  ( -32.71604765022082972, -79.95000206843607771, -22.50489820171189592 ) ) ;
#15518=CARTESIAN_POINT ( 'NONE',  ( -41.00000000000000000, -84.00000000000000000, -10.20110288159999890 ) ) ;
#15519=CARTESIAN_POINT ( 'NONE',  ( 8.988996100299999625, -34.66800400750000222, -19.43643858049999906 ) ) ;
#15521=CARTESIAN_POINT ( 'NONE',  ( 22.20230814393099550, -19.49660179756074996, 9.763414323654941995 ) ) ;
#15522=CARTESIAN_POINT ( 'NONE',  ( -40.70731707320000226, -74.50000000000000000, -7.215414233289999757 ) ) ;
#15525=VECTOR ( 'NONE', #4608, 1000.000000000000114 ) ;
#15526=DIRECTION ( 'NONE',  ( 0.000000000000000000, -1.000000000000000000, 0.000000000000000000 ) ) ;
#15532=CARTESIAN_POINT ( 'NONE',  ( 24.87134706483404401, -38.85105898717574036, 1.395915593889689665 ) ) ;
#15535=ORIENTED_EDGE ( 'NONE', *, *, #22960, .T. ) ;
#15539=ORIENTED_EDGE ( 'NONE', *, *, #9610, .T. ) ;
#15542=CARTESIAN_POINT ( 'NONE',  ( 46.52944179779999700, -74.00708935479998729, -3.668904617159999937 ) ) ;
#15546=FACE_OUTER_BOUND ( 'NONE', #23437, .T. ) ;
#15554=CARTESIAN_POINT ( 'NONE',  ( -21.73289126959999962, -74.33689811570000927, -32.66619185449999918 ) ) ;
#15558=CARTESIAN_POINT ( 'NONE',  ( 7.315281843798212336, -74.28334043001960652, -40.00441865863449209 ) ) ;
#15559=VERTEX_POINT ( 'NONE', #17861 ) ;
#15560=CARTESIAN_POINT ( 'NONE',  ( -7.325370793560000315, -19.50000000000000000, -24.94672208400000102 ) ) ;
#15562=CARTESIAN_POINT ( 'NONE',  ( 7.066909182079999852, -57.47855601759999900, -22.26662627820000040 ) ) ;
#15563=DIRECTION ( 'NONE',  ( 0.000000000000000000, 1.000000000000000000, 0.000000000000000000 ) ) ;
#15564=DIRECTION ( 'NONE',  ( 0.000000000000000000, 0.000000000000000000, 1.000000000000000000 ) ) ;
#15568=B_SPLINE_CURVE_WITH_KNOTS ( 'NONE', 5,
 ( #22648, #2690, #14868, #3544, #25965, #3272, #12272, #966, #16943, #25546, #5989, #10211 ),
 .UNSPECIFIED., .F., .F.,
 ( 6, 3, 3, 6 ),
 ( 0.000000000000000000, 0.2521440085671421416, 0.5186391376505576911, 1.000000000000000000 ),
 .UNSPECIFIED. ) ;
#15570=CIRCLE ( 'NONE', #4418, 6.749999999999999112 ) ;
#15571=EDGE_CURVE ( 'NONE', #10144, #2030, #26023, .T. ) ;
#15572=DIRECTION ( 'NONE',  ( 0.000000000000000000, -1.000000000000000000, 0.000000000000000000 ) ) ;
#15573=ADVANCED_FACE ( 'NONE', ( #19016 ), #25439, .F. ) ;
#15574=ORIENTED_EDGE ( 'NONE', *, *, #17899, .F. ) ;
#15577=ORIENTED_EDGE ( 'NONE', *, *, #13034, .F. ) ;
#15578=DIRECTION ( 'NONE',  ( 1.000000000000000000, 0.000000000000000000, 0.000000000000000000 ) ) ;
#15579=DIRECTION ( 'NONE',  ( 1.000000000000000000, 0.000000000000000000, 0.000000000000000000 ) ) ;
#15584=ORIENTED_EDGE ( 'NONE', *, *, #13110, .F. ) ;
#15587=CARTESIAN_POINT ( 'NONE',  ( 23.35417726369999869, -57.47855601759999900, -0.5711878298099999363 ) ) ;
#15589=DIRECTION ( 'NONE',  ( 1.000000000000000000, 0.000000000000000000, 0.000000000000000000 ) ) ;
#15590=CARTESIAN_POINT ( 'NONE',  ( -11.34376786329999831, -18.85523522049999912, -18.72653253400000040 ) ) ;
#15591=CARTESIAN_POINT ( 'NONE',  ( -12.09704001540000107, -74.50000000000000000, 47.10905722069999513 ) ) ;
#15595=CARTESIAN_POINT ( 'NONE',  ( 0.000000000000000000, -65.07443093669999712, 0.000000000000000000 ) ) ;
#15597=ORIENTED_EDGE ( 'NONE', *, *, #16653, .T. ) ;
#15598=CARTESIAN_POINT ( 'NONE',  ( -20.45998242170000125, -52.56313962710000709, 14.78974999389999923 ) ) ;
#15602=CARTESIAN_POINT ( 'NONE',  ( 27.81679767680000026, -70.78636603370000557, 1.651879667569999821 ) ) ;
#15604=CARTESIAN_POINT ( 'NONE',  ( 26.46383138103869470, -74.36567512596400320, -28.96817324696392859 ) ) ;
#15605=CARTESIAN_POINT ( 'NONE',  ( 21.58746088380000216, -36.00000000000000000, -10.99658662490000083 ) ) ;
#15606=CARTESIAN_POINT ( 'NONE',  ( -11.05123306399999983, -49.83808240359999786, -21.57293782270000193 ) ) ;
#15607=DIRECTION ( 'NONE',  ( -1.135974695539999883E-15, 0.000000000000000000, -1.000000000000000000 ) ) ;
#15608=DIRECTION ( 'NONE',  ( -0.9952295494196657932, 0.000000000000000000, -0.09756097560976527416 ) ) ;
#15609=EDGE_CURVE ( 'NONE', #11090, #1612, #14228, .T. ) ;
#15612=CARTESIAN_POINT ( 'NONE',  ( 7.315286554507971495, -74.28332971671856910, 40.00438978216653396 ) ) ;
#15615=LINE ( 'NONE', #4990, #14371 ) ;
#15617=EDGE_CURVE ( 'NONE', #20540, #24483, #24638, .T. ) ;
#15618=CARTESIAN_POINT ( 'NONE',  ( 23.24501621210006874, -19.48040731474316445, 1.335160801108107309 ) ) ;
#15621=CARTESIAN_POINT ( 'NONE',  ( 26.81408956065956062, -72.66570736699186739, -10.40602720322819508 ) ) ;
#15622=CARTESIAN_POINT ( 'NONE',  ( 9.115928523210000023, -35.98566164980000082, -20.35866484339999616 ) ) ;
#15623=CARTESIAN_POINT ( 'NONE',  ( 21.21808891099999883, -34.59820414320000026, -7.670974023059999425 ) ) ;
#15626=FACE_OUTER_BOUND ( 'NONE', #462, .T. ) ;
#15627=CARTESIAN_POINT ( 'NONE',  ( -12.22851712105154220, -19.47229981159569334, 19.17184709748261540 ) ) ;
#15630=ORIENTED_EDGE ( 'NONE', *, *, #24442, .F. ) ;
#15632=CARTESIAN_POINT ( 'NONE',  ( 28.53389931306142913, -70.75059817112114047, 2.680123202356653245 ) ) ;
#15638=CARTESIAN_POINT ( 'NONE',  ( -14.25726283530000060, -18.50000000000000000, 19.69500409140000130 ) ) ;
#15640=CARTESIAN_POINT ( 'NONE',  ( 36.29172713509999681, -75.00000018049999539, -14.94947828099999931 ) ) ;
#15643=CARTESIAN_POINT ( 'NONE',  ( -14.36794459300000071, -65.11374573150000344, 21.98892381860000000 ) ) ;
#15648=CARTESIAN_POINT ( 'NONE',  ( -19.88433733760000166, -55.05574748869999979, 12.10004687989999894 ) ) ;
#15652=EDGE_LOOP ( 'NONE', ( #12924, #20510, #17780, #22239 ) ) ;
#15653=CARTESIAN_POINT ( 'NONE',  ( -7.318372426699999878, -73.93831497249999529, -38.68350751799999898 ) ) ;
#15654=CARTESIAN_POINT ( 'NONE',  ( 29.28066344122883535, -74.33029147470158193, -26.09360328796791961 ) ) ;
#15655=CARTESIAN_POINT ( 'NONE',  ( 7.268564243840000216, -74.08838618790001362, -39.96405812909999611 ) ) ;
#15657=CARTESIAN_POINT ( 'NONE',  ( 8.472395020760000506, -37.95144078679999922, -21.79230213740000011 ) ) ;
#15658=CARTESIAN_POINT ( 'NONE',  ( 28.69894246159999796, -72.00000000000000000, -10.33698060819999931 ) ) ;
#15660=CARTESIAN_POINT ( 'NONE',  ( 22.47717647029999810, -39.30675845300000049, 9.993032863299999846 ) ) ;
#15663=CARTESIAN_POINT ( 'NONE',  ( 20.16274462490000019, -18.85622860559999836, 9.471810047709999125 ) ) ;
#15664=CARTESIAN_POINT ( 'NONE',  ( 8.888943361349999961, -68.13650396850000845, -25.01879546389999831 ) ) ;
#15666=B_SPLINE_SURFACE_WITH_KNOTS ( 'NONE', 5, 5, ( 
 ( #16254, #25164, #5197, #13781, #20650, #18159 ),
 ( #16406, #2727, #5482, #9560, #11884, #849 ),
 ( #27058, #561, #7100, #24867, #11582, #18314 ),
 ( #5042, #22833, #18608, #2878, #708, #5758 ),
 ( #21771, #1546, #14644, #23541, #12720, #26152 ),
 ( #8088, #8219, #10522, #21348, #3577, #21632 ),
 ( #6175, #9979, #26000, #1682, #12437, #28187 ),
 ( #10389, #1407, #17111, #7814, #28323, #12308 ),
 ( #19436, #18893, #17255, #19028, #5893, #8354 ) ),
 .UNSPECIFIED., .F., .F., .F.,
 ( 6, 3, 6 ),
 ( 6, 6 ),
 ( 5.946593705439999766, 13.87007241820000125, 18.04675716799999918 ),
 ( 0.000000000000000000, 2.000000000000000000 ),
 .UNSPECIFIED. ) ;
#15667=VERTEX_POINT ( 'NONE', #22972 ) ;
#15669=DIRECTION ( 'NONE',  ( -0.9704142011833034598, 0.000000000000000000, 0.2414462220490750932 ) ) ;
#15671=CARTESIAN_POINT ( 'NONE',  ( 9.475766568499999210, -36.00000000000000000, -19.97576656850000276 ) ) ;
#15672=CARTESIAN_POINT ( 'NONE',  ( 23.08464880861777146, -62.66433083247308389, -7.365532055905221753 ) ) ;
#15675=ORIENTED_EDGE ( 'NONE', *, *, #18102, .T. ) ;
#15678=AXIS2_PLACEMENT_3D ( 'NONE', #9917, #27720, #16767 ) ;
#15679=DIRECTION ( 'NONE',  ( 0.000000000000000000, -1.000000000000000000, 0.000000000000000000 ) ) ;
#15680=CARTESIAN_POINT ( 'NONE',  ( 24.70618715508873109, -32.10667435201317943, 1.410068405398430924 ) ) ;
#15682=B_SPLINE_CURVE_WITH_KNOTS ( 'NONE', 3,
 ( #12456, #25469, #5500, #28073, #21369, #14392, #10270, #19183, #5911, #14793, #23695, #21943, #17569, #24121, #19743, #15657 ),
 .UNSPECIFIED., .F., .F.,
 ( 4, 2, 2, 1, 1, 1, 1, 2, 2, 4 ),
 ( 0.000000000000000000, 0.2500000000001303402, 0.3750000000002007838, 0.4375000000002303158, 0.4687500000002451372, 0.4843750000002524647, 0.4921875000002564615, 0.4960937500002529088, 0.5000000000002493561, 1.000000000000000000 ),
 .UNSPECIFIED. ) ;
#15683=ORIENTED_EDGE ( 'NONE', *, *, #22711, .T. ) ;
#15684=VERTEX_POINT ( 'NONE', #1260 ) ;
#15686=CARTESIAN_POINT ( 'NONE',  ( -13.12175661516558911, -71.04369398208616815, -24.58936394580375406 ) ) ;
#15690=CARTESIAN_POINT ( 'NONE',  ( -22.48295016580000194, -80.00863955980000242, -32.56379889600000155 ) ) ;
#15691=CIRCLE ( 'NONE', #3174, 10.00000000000000000 ) ;
#15698=CARTESIAN_POINT ( 'NONE',  ( -2.617290931510000362, -61.32329206099999652, -25.60467908629999911 ) ) ;
#15699=CARTESIAN_POINT ( 'NONE',  ( -39.18053445169999804, -73.62955962630000784, 7.219524535890000649 ) ) ;
#15700=CARTESIAN_POINT ( 'NONE',  ( -22.13232332860000184, -74.41849501830000690, -32.73892504640000567 ) ) ;
#15701=CARTESIAN_POINT ( 'NONE',  ( -0.8479692466189999722, -57.47815920199999340, -23.34776748810000058 ) ) ;
#15703=CARTESIAN_POINT ( 'NONE',  ( 7.426814492070000107, -35.28814190290000141, -21.34788074219999743 ) ) ;
#15704=FACE_OUTER_BOUND ( 'NONE', #15193, .T. ) ;
#15705=CARTESIAN_POINT ( 'NONE',  ( -18.59146871949999991, -19.47458110719999880, 13.41216391400000063 ) ) ;
#15706=VERTEX_POINT ( 'NONE', #10096 ) ;
#15709=CARTESIAN_POINT ( 'NONE',  ( 20.36016146999999776, -74.00000000000000000, -32.97008227039999895 ) ) ;
#15714=AXIS2_PLACEMENT_3D ( 'NONE', #24992, #544, #18588 ) ;
#15719=EDGE_LOOP ( 'NONE', ( #20602, #21225, #21789, #9546 ) ) ;
#15721=CARTESIAN_POINT ( 'NONE',  ( 9.024080808563812894, -19.23820059856630138, -18.94592219493823038 ) ) ;
#15722=MANIFOLD_SOLID_BREP ( 'Body', #14679 ) ;
#15724=CARTESIAN_POINT ( 'NONE',  ( 30.51745573710000059, -72.51545259190000081, -23.74117753099999817 ) ) ;
#15725=B_SPLINE_SURFACE_WITH_KNOTS ( 'NONE', 5, 5, ( 
 ( #19462, #14799, #5916, #28350, #8381, #17286 ),
 ( #13039, #26178, #15076, #23985, #17002, #21950 ),
 ( #19610, #12607, #23699, #1853, #4019, #21516 ),
 ( #1575, #10415, #19333, #12881, #21797, #28493 ),
 ( #8531, #6348, #15212, #1997, #13189, #4759 ),
 ( #9259, #6802, #13780, #15663, #24566, #20489 ),
 ( #26911, #17871, #18158, #2587, #11434, #2140 ),
 ( #27201, #20337, #6651, #15514, #270, #27057 ),
 ( #15962, #11131, #22681, #9112, #7099, #4461 ) ),
 .UNSPECIFIED., .F., .F., .F.,
 ( 6, 3, 6 ),
 ( 6, 6 ),
 ( 0.000000000000000000, 2.252774941560000244, 5.576981603820000188 ),
 ( 0.000000000000000000, 1.000000000000000000 ),
 .UNSPECIFIED. ) ;
#15728=DIRECTION ( 'NONE',  ( 0.000000000000000000, 1.000000000000000000, 0.000000000000000000 ) ) ;
#15730=CARTESIAN_POINT ( 'NONE',  ( -10.93437420129999893, -19.18584095090000119, -21.85842446839999909 ) ) ;
#15731=CARTESIAN_POINT ( 'NONE',  ( 21.59599020914462386, -37.77569117438354596, -8.026336239905948133 ) ) ;
#15736=ADVANCED_FACE ( 'NONE', ( #10650 ), #11873, .T. ) ;
#15742=EDGE_LOOP ( 'NONE', ( #16947, #5815 ) ) ;
#15748=CARTESIAN_POINT ( 'NONE',  ( 4.534235129290000123E-15, -69.00000000000000000, -36.25000000000000000 ) ) ;
#15749=EDGE_CURVE ( 'NONE', #18911, #19124, #23609, .T. ) ;
#15750=EDGE_CURVE ( 'NONE', #4330, #27046, #6888, .T. ) ;
#15753=AXIS2_PLACEMENT_3D ( 'NONE', #6527, #19913, #4042 ) ;
#15755=AXIS2_PLACEMENT_3D ( 'NONE', #17006, #21248, #23438 ) ;
#15756=VERTEX_POINT ( 'NONE', #28307 ) ;
#15759=AXIS2_PLACEMENT_3D ( 'NONE', #6163, #4420, #10939 ) ;
#15762=CARTESIAN_POINT ( 'NONE',  ( 7.472970580910000216, -74.00000000000000000, 38.65569705749999940 ) ) ;
#15764=CARTESIAN_POINT ( 'NONE',  ( 22.05085473011402186, -19.46454039567884564, -0.1739277095649396365 ) ) ;
#15765=ORIENTED_EDGE ( 'NONE', *, *, #12301, .F. ) ;
#15766=DIRECTION ( 'NONE',  ( 0.000000000000000000, -1.000000000000000000, 0.000000000000000000 ) ) ;
#15767=FACE_OUTER_BOUND ( 'NONE', #3885, .T. ) ;
#15768=CARTESIAN_POINT ( 'NONE',  ( 8.470925167420000790, -36.97944905069999777, -21.53314064279999940 ) ) ;
#15769=CARTESIAN_POINT ( 'NONE',  ( 21.31604162444098804, -34.85188264325164198, -7.422259252942775554 ) ) ;
#15771=CARTESIAN_POINT ( 'NONE',  ( 23.98860504829999840, -18.86819686409999974, 1.664881634730000171 ) ) ;
#15779=EDGE_CURVE ( 'NONE', #8106, #13332, #16950, .T. ) ;
#15780=AXIS2_PLACEMENT_3D ( 'NONE', #22309, #17943, #9178 ) ;
#15783=CARTESIAN_POINT ( 'NONE',  ( 21.88811475929999872, -37.33710342420000217, -8.645795876960001181 ) ) ;
#15784=CARTESIAN_POINT ( 'NONE',  ( -12.05825490610000195, -67.66818692689999182, -24.37625710889999908 ) ) ;
#15788=EDGE_CURVE ( 'NONE', #26473, #1175, #10239, .T. ) ;
#15791=CARTESIAN_POINT ( 'NONE',  ( -13.58047762579999862, -66.16285484500001246, 21.97899781390000129 ) ) ;
#15792=CARTESIAN_POINT ( 'NONE',  ( -13.44714549129999881, -61.83339493489999938, 20.99574822410000152 ) ) ;
#15793=CARTESIAN_POINT ( 'NONE',  ( 7.247546674742445738, -74.11886065931342671, 40.20585889373907662 ) ) ;
#15798=B_SPLINE_CURVE_WITH_KNOTS ( 'NONE', 5,
 ( #823, #11552, #7209, #9666, #13899, #18573, #12134, #25421, #9950 ),
 .UNSPECIFIED., .F., .F.,
 ( 6, 3, 6 ),
 ( 0.000000000000000000, 0.5000000000000000000, 1.000000000000000000 ),
 .UNSPECIFIED. ) ;
#15802=CARTESIAN_POINT ( 'NONE',  ( -7.279135155890000597, -73.90050421709999284, -39.59102417159999021 ) ) ;
#15804=EDGE_LOOP ( 'NONE', ( #9942, #21272, #1316, #27901 ) ) ;
#15805=CARTESIAN_POINT ( 'NONE',  ( 0.000000000000000000, -72.82938648530000592, 0.000000000000000000 ) ) ;
#15806=ORIENTED_EDGE ( 'NONE', *, *, #26685, .F. ) ;
#15808=CARTESIAN_POINT ( 'NONE',  ( 21.75855414729999993, -19.41837863929999841, 9.513576305009999956 ) ) ;
#15812=EDGE_CURVE ( 'NONE', #28497, #9424, #26887, .T. ) ;
#15813=CARTESIAN_POINT ( 'NONE',  ( 20.57008778049999975, -58.79569913830000161, 11.24574759670000113 ) ) ;
#15814=CARTESIAN_POINT ( 'NONE',  ( 10.72517777600000066, -69.13421244780001018, -25.99822748240000081 ) ) ;
#15816=ORIENTED_EDGE ( 'NONE', *, *, #15360, .T. ) ;
#15817=CARTESIAN_POINT ( 'NONE',  ( -10.20110288159999890, -84.00000000000000000, 41.00000000000000000 ) ) ;
#15820=CARTESIAN_POINT ( 'NONE',  ( 20.74876991574076968, -19.47341637985504192, 9.495871454077789764 ) ) ;
#15822=CARTESIAN_POINT ( 'NONE',  ( -40.70731707320000226, -74.50000000000000000, -7.215414233289999757 ) ) ;
#15825=EDGE_CURVE ( 'NONE', #178, #7860, #3601, .T. ) ;
#15829=DIRECTION ( 'NONE',  ( 1.000000000000000000, 0.000000000000000000, 0.000000000000000000 ) ) ;
#15830=CARTESIAN_POINT ( 'NONE',  ( 0.000000000000000000, -77.00000000000000000, -40.00000000000000000 ) ) ;
#15832=EDGE_LOOP ( 'NONE', ( #11145, #587, #2700, #2973, #24136, #6744, #24699 ) ) ;
#15833=CYLINDRICAL_SURFACE ( 'NONE', #14933, 7.250000000000004441 ) ;
#15834=ORIENTED_EDGE ( 'NONE', *, *, #21022, .F. ) ;
#15835=CARTESIAN_POINT ( 'NONE',  ( -23.03458422004786854, -71.75398255365567479, 16.25737041499285951 ) ) ;
#15837=CARTESIAN_POINT ( 'NONE',  ( 47.03569028360000459, -74.19054636589999063, -1.774065497670000102 ) ) ;
#15841=CARTESIAN_POINT ( 'NONE',  ( -22.46797589350000024, -80.18584073460000639, -32.25831116089999995 ) ) ;
#15844=CARTESIAN_POINT ( 'NONE',  ( 8.514971421829999443, -37.95267571699999820, -21.81705067669999920 ) ) ;
#15846=DIRECTION ( 'NONE',  ( 0.000000000000000000, 1.000000000000000000, 0.000000000000000000 ) ) ;
#15849=EDGE_CURVE ( 'NONE', #22782, #25354, #1955, .T. ) ;
#15852=CARTESIAN_POINT ( 'NONE',  ( -21.60034937969999902, -74.39508596250000494, -32.77174707999999725 ) ) ;
#15855=CARTESIAN_POINT ( 'NONE',  ( -7.521798597035361134, -73.99983172279489452, 38.87042118007536118 ) ) ;
#15856=CARTESIAN_POINT ( 'NONE',  ( -18.44071070329999884, -19.46458168459999882, 12.28140447959999904 ) ) ;
#15859=DIRECTION ( 'NONE',  ( 0.000000000000000000, -1.000000000000000000, 0.000000000000000000 ) ) ;
#15860=CARTESIAN_POINT ( 'NONE',  ( 8.408939714870001580, -35.33620304669999257, -20.95510900379999697 ) ) ;
#15863=CARTESIAN_POINT ( 'NONE',  ( 22.45957212889999965, -52.58489974409999945, 10.08523539449999973 ) ) ;
#15864=CIRCLE ( 'NONE', #2850, 3.000000000000000888 ) ;
#15869=CARTESIAN_POINT ( 'NONE',  ( 24.42476877459999685, -57.44036991850000362, 1.191907264949999989 ) ) ;
#15870=CIRCLE ( 'NONE', #7053, 3.750000000000000000 ) ;
#15871=DIRECTION ( 'NONE',  ( 0.000000000000000000, -1.000000000000000000, 0.000000000000000000 ) ) ;
#15872=VERTEX_POINT ( 'NONE', #14633 ) ;
#15874=DIRECTION ( 'NONE',  ( 0.000000000000000000, -1.000000000000000000, 0.000000000000000000 ) ) ;
#15876=CARTESIAN_POINT ( 'NONE',  ( 28.91458899939999938, -72.00000000000000000, 3.086557976320000396 ) ) ;
#15879=CARTESIAN_POINT ( 'NONE',  ( 27.75394116159999669, -74.50000000000000000, -27.75394116159999669 ) ) ;
#15884=AXIS2_PLACEMENT_3D ( 'NONE', #17510, #26395, #8188 ) ;
#15885=CARTESIAN_POINT ( 'NONE',  ( 21.74745445608735039, -37.94920488029457317, -8.395240280012213674 ) ) ;
#15892=ORIENTED_EDGE ( 'NONE', *, *, #3932, .F. ) ;
#15896=ORIENTED_EDGE ( 'NONE', *, *, #1331, .T. ) ;
#15899=CARTESIAN_POINT ( 'NONE',  ( -18.48358769389999878, -19.46501104080000033, 12.15083731070000184 ) ) ;
#15900=CARTESIAN_POINT ( 'NONE',  ( 26.06532122270797203, -74.32759098968446665, -29.30452812900732340 ) ) ;
#15901=CARTESIAN_POINT ( 'NONE',  ( 20.33566493080000015, -36.00000000000000000, -9.885503730140001721 ) ) ;
#15902=CARTESIAN_POINT ( 'NONE',  ( -14.80839208230898407, -74.26929999394664605, 36.28872789036408619 ) ) ;
#15906=ADVANCED_FACE ( 'NONE', ( #28727 ), #27355, .T. ) ;
#15908=CARTESIAN_POINT ( 'NONE',  ( 23.98460332450000010, -18.50000000000000000, 2.503291441710000065 ) ) ;
#15912=CARTESIAN_POINT ( 'NONE',  ( 7.268571389559999929, -74.08839659379999887, 39.96417052329999819 ) ) ;
#15914=B_SPLINE_SURFACE_WITH_KNOTS ( 'NONE', 5, 5, ( 
 ( #6570, #184, #26249, #15590, #28562, #8597 ),
 ( #21867, #15433, #15137, #28415, #24489, #24047 ),
 ( #4386, #4085, #17792, #17499, #24345, #26385 ),
 ( #13255, #26682, #4523, #6413, #12811, #22306 ),
 ( #9034, #21721, #12954, #1918, #2504, #332 ),
 ( #25236, #2944, #16325, #5119, #778, #24792 ),
 ( #4830, #3094, #482, #26834, #18383, #16174 ),
 ( #6866, #27270, #24937, #7166, #16032, #24643 ),
 ( #11359, #18523, #11504, #2652, #15730, #22905 ) ),
 .UNSPECIFIED., .F., .F., .F.,
 ( 6, 3, 6 ),
 ( 6, 6 ),
 ( 5.892872301239999241E-16, 2.251105814059999766, 5.576980695549999645 ),
 ( 0.000000000000000000, 1.000000000000000000 ),
 .UNSPECIFIED. ) ;
#15915=CARTESIAN_POINT ( 'NONE',  ( 21.44286899589999962, -36.30033507760000333, -7.882324037790000126 ) ) ;
#15916=CARTESIAN_POINT ( 'NONE',  ( 26.83947876876618821, -72.50065199416241057, -10.87728020417079833 ) ) ;
#15917=CARTESIAN_POINT ( 'NONE',  ( 7.799278058849999695, -37.54433185199999912, -21.53604737210000053 ) ) ;
#15918=ADVANCED_FACE ( 'NONE', ( #2538 ), #17678, .T. ) ;
#15921=AXIS2_PLACEMENT_3D ( 'NONE', #3159, #21209, #1916 ) ;
#15922=CARTESIAN_POINT ( 'NONE',  ( 23.97709848270000066, -18.50000000000000000, 2.237158816650000048 ) ) ;
#15924=DIRECTION ( 'NONE',  ( 1.000000000000000000, 0.000000000000000000, 0.000000000000000000 ) ) ;
#15925=ORIENTED_EDGE ( 'NONE', *, *, #26947, .F. ) ;
#15926=CYLINDRICAL_SURFACE ( 'NONE', #3711, 0.4999999999999982236 ) ;
#15927=AXIS2_PLACEMENT_3D ( 'NONE', #8905, #9352, #11527 ) ;
#15928=CARTESIAN_POINT ( 'NONE',  ( 27.49607050420000220, -67.46050995630001523, 1.934818144049999855 ) ) ;
#15931=CARTESIAN_POINT ( 'NONE',  ( 26.46310988749999993, -64.24504445130001784, 1.532420830840000026 ) ) ;
#15932=CARTESIAN_POINT ( 'NONE',  ( 40.00000000000000000, -84.50000000000000000, 4.463096558990000197E-15 ) ) ;
#15933=FACE_OUTER_BOUND ( 'NONE', #11893, .T. ) ;
#15935=CARTESIAN_POINT ( 'NONE',  ( 36.29172688410000092, -74.90632999339999287, -14.94947910089999965 ) ) ;
#15936=CARTESIAN_POINT ( 'NONE',  ( -22.41809188630069727, -79.89426907611134254, -32.75488367496921427 ) ) ;
#15937=CARTESIAN_POINT ( 'NONE',  ( -14.25684790429999893, -62.95263723189999183, 21.84526217519999847 ) ) ;
#15939=CARTESIAN_POINT ( 'NONE',  ( -12.03461033140000147, -62.10472517099999834, 20.80665457679999975 ) ) ;
#15940=DIRECTION ( 'NONE',  ( 1.000000000000000000, 0.000000000000000000, 0.000000000000000000 ) ) ;
#15942=CARTESIAN_POINT ( 'NONE',  ( 26.85539570426266920, -72.18744871742090652, 10.61487170321338347 ) ) ;
#15945=CARTESIAN_POINT ( 'NONE',  ( 20.27618985420000186, -36.00000000000000000, -9.807089787700000727 ) ) ;
#15949=EDGE_LOOP ( 'NONE', ( #11567, #28332, #17639 ) ) ;
#15950=CARTESIAN_POINT ( 'NONE',  ( -7.215414233289999757, -74.50000000000000000, -40.70731707320000226 ) ) ;
#15954=EDGE_CURVE ( 'NONE', #4525, #6019, #24955, .T. ) ;
#15956=EDGE_CURVE ( 'NONE', #18344, #14992, #7800, .T. ) ;
#15960=CARTESIAN_POINT ( 'NONE',  ( -16.67828388959999941, -74.50000000000000000, 44.75374114529999758 ) ) ;
#15961=DIRECTION ( 'NONE',  ( 1.000000000000000000, 0.000000000000000000, 0.000000000000000000 ) ) ;
#15962=CARTESIAN_POINT ( 'NONE',  ( 18.48933855830000184, -18.50000000000000000, 10.02928721039999971 ) ) ;
#15965=ORIENTED_EDGE ( 'NONE', *, *, #17367, .T. ) ;
#15966=CIRCLE ( 'NONE', #10746, 2.000000000000000888 ) ;
#15967=DIRECTION ( 'NONE',  ( 0.000000000000000000, 0.000000000000000000, -1.000000000000000000 ) ) ;
#15970=CARTESIAN_POINT ( 'NONE',  ( 20.88115893480090790, -19.47504441211762227, 9.474803371222611403 ) ) ;
#15971=CARTESIAN_POINT ( 'NONE',  ( 22.75601413952083263, -61.35865215156498920, -7.240038726238430478 ) ) ;
#15972=ORIENTED_EDGE ( 'NONE', *, *, #23619, .F. ) ;
#15973=DIRECTION ( 'NONE',  ( 0.000000000000000000, 1.000000000000000000, 0.000000000000000000 ) ) ;
#15974=VERTEX_POINT ( 'NONE', #4269 ) ;
#15980=EDGE_CURVE ( 'NONE', #300, #26675, #23174, .T. ) ;
#15983=CARTESIAN_POINT ( 'NONE',  ( -22.55319281656417729, -69.29687318610271518, 14.97856516669103399 ) ) ;
#15984=CARTESIAN_POINT ( 'NONE',  ( 21.06416788030000120, -36.18018306559999786, -9.332951880679999590 ) ) ;
#15985=CARTESIAN_POINT ( 'NONE',  ( 47.13359351679999776, -74.47757638999999585, -1.343551159269999795 ) ) ;
#15989=CARTESIAN_POINT ( 'NONE',  ( -11.66011925523032922, -62.65979579072126882, 21.24220495570105882 ) ) ;
#15990=ADVANCED_FACE ( 'NONE', ( #13436 ), #18966, .T. ) ;
#15991=SPHERICAL_SURFACE ( 'NONE', #1964, 1.000000000000000000 ) ;
#15996=CARTESIAN_POINT ( 'NONE',  ( 36.39554599249999711, -74.16575166410000008, -14.53417042330000086 ) ) ;
#15999=CARTESIAN_POINT ( 'NONE',  ( -39.89387480210000092, -74.19145785139998850, 7.305170733980000719 ) ) ;
#16001=CARTESIAN_POINT ( 'NONE',  ( -21.99985828019999801, -74.00000000000000000, -31.89935321680000158 ) ) ;
#16002=EDGE_LOOP ( 'NONE', ( #59, #10135, #14823, #5748 ) ) ;
#16005=CARTESIAN_POINT ( 'NONE',  ( -17.41808129929999893, -18.50000000000000000, 12.13953735139999957 ) ) ;
#16006=ORIENTED_EDGE ( 'NONE', *, *, #4464, .T. ) ;
#16008=CARTESIAN_POINT ( 'NONE',  ( 23.22783021959999772, -61.45046333410000017, 10.43375156039999929 ) ) ;
#16009=CARTESIAN_POINT ( 'NONE',  ( 7.670972941899999675, -34.59820487809999889, -21.21808928440000130 ) ) ;
#16012=ORIENTED_EDGE ( 'NONE', *, *, #4842, .F. ) ;
#16016=CARTESIAN_POINT ( 'NONE',  ( -11.84271430029999905, -64.58097566740001128, -22.96390433080000193 ) ) ;
#16017=CARTESIAN_POINT ( 'NONE',  ( 36.91823499837838085, -79.75463803037827404, -14.40641522487323023 ) ) ;
#16021=EDGE_CURVE ( 'NONE', #7301, #7043, #14174, .T. ) ;
#16022=FACE_OUTER_BOUND ( 'NONE', #14224, .T. ) ;
#16028=ADVANCED_FACE ( 'NONE', ( #11687 ), #2215, .F. ) ;
#16030=DIRECTION ( 'NONE',  ( 0.000000000000000000, -1.000000000000000000, 0.000000000000000000 ) ) ;
#16032=CARTESIAN_POINT ( 'NONE',  ( -10.66364198750000014, -19.17999199609999650, -21.54557793210000227 ) ) ;
#16033=CARTESIAN_POINT ( 'NONE',  ( 21.52462730065835572, -37.46071944955636468, -7.740090088892075393 ) ) ;
#16034=VERTEX_POINT ( 'NONE', #11978 ) ;
#16037=CARTESIAN_POINT ( 'NONE',  ( 40.21639064484389081, -74.12723354410567822, 7.246819345891047703 ) ) ;
#16038=VERTEX_POINT ( 'NONE', #956 ) ;
#16040=CARTESIAN_POINT ( 'NONE',  ( 38.08875739639999836, -82.25000000000000000, -9.476764215410000247 ) ) ;
#16045=EDGE_CURVE ( 'NONE', #26105, #5689, #1322, .T. ) ;
#16048=CARTESIAN_POINT ( 'NONE',  ( 25.26718046270000073, -19.50000000000000000, 6.129403842640000377 ) ) ;
#16050=CARTESIAN_POINT ( 'NONE',  ( -14.61005163810492391, -74.14612126337357267, 36.27173304699432066 ) ) ;
#16051=CARTESIAN_POINT ( 'NONE',  ( -19.35716652280000005, -18.50000000000000000, 15.34467299940000018 ) ) ;
#16052=ADVANCED_FACE ( 'NONE', ( #809 ), #7641, .T. ) ;
#16054=ADVANCED_FACE ( 'NONE', ( #1093 ), #4999, .T. ) ;
#16055=PLANE ( 'NONE',  #8593 ) ;
#16057=CARTESIAN_POINT ( 'NONE',  ( -10.20110288159999890, -80.50000000000000000, 41.00000000000000000 ) ) ;
#16060=CARTESIAN_POINT ( 'NONE',  ( 7.732662040940000203, -18.50000000000000000, -19.49253883449999947 ) ) ;
#16061=CARTESIAN_POINT ( 'NONE',  ( 19.55068592539999983, -35.72724453810000256, -9.038647860560001135 ) ) ;
#16062=DIRECTION ( 'NONE',  ( 0.000000000000000000, 1.000000000000000000, 0.000000000000000000 ) ) ;
#16063=CARTESIAN_POINT ( 'NONE',  ( -5.679770007689999289, -74.50000000000000000, 46.75000000000000000 ) ) ;
#16064=CARTESIAN_POINT ( 'NONE',  ( 8.724064349480000757, -36.49187789639999835, -21.25496272479999860 ) ) ;
#16066=ORIENTED_EDGE ( 'NONE', *, *, #191, .T. ) ;
#16068=DIRECTION ( 'NONE',  ( 0.2414462220490750377, 0.000000000000000000, -0.9704142011833034598 ) ) ;
#16073=DIRECTION ( 'NONE',  ( 0.000000000000000000, -1.000000000000000000, 0.000000000000000000 ) ) ;
#16077=AXIS2_PLACEMENT_3D ( 'NONE', #17937, #7015, #15276 ) ;
#16078=DIRECTION ( 'NONE',  ( 0.000000000000000000, -1.000000000000000000, 0.000000000000000000 ) ) ;
#16079=CARTESIAN_POINT ( 'NONE',  ( 22.58640054960000043, -44.88560226349999738, -9.205819528950000219 ) ) ;
#16083=CARTESIAN_POINT ( 'NONE',  ( 36.47289884999999998, -75.00000018510000643, -14.78463685610000056 ) ) ;
#16087=CARTESIAN_POINT ( 'NONE',  ( -13.31744303520000017, -66.93384306320000121, 22.33243309759999917 ) ) ;
#16088=CARTESIAN_POINT ( 'NONE',  ( 9.020398574519999713, -35.69157542760000013, -19.55164510480000217 ) ) ;
#16089=CARTESIAN_POINT ( 'NONE',  ( 40.00000000000000000, -80.50000000000000000, -7.105427357599999217E-15 ) ) ;
#16090=CARTESIAN_POINT ( 'NONE',  ( 21.79230218349999859, -37.95144078439999902, -8.472395100330000872 ) ) ;
#16095=VERTEX_POINT ( 'NONE', #22787 ) ;
#16096=CARTESIAN_POINT ( 'NONE',  ( 27.75394116159999669, -74.50000000000000000, -27.75394116159999669 ) ) ;
#16100=ORIENTED_EDGE ( 'NONE', *, *, #17324, .F. ) ;
#16104=AXIS2_PLACEMENT_3D ( 'NONE', #26400, #24807, #15450 ) ;
#16106=CARTESIAN_POINT ( 'NONE',  ( -14.47017326849999996, -74.22762369209999633, 36.54526597599999604 ) ) ;
#16107=FACE_OUTER_BOUND ( 'NONE', #12071, .T. ) ;
#16109=ORIENTED_EDGE ( 'NONE', *, *, #3589, .F. ) ;
#16110=CARTESIAN_POINT ( 'NONE',  ( -12.22686266070000194, -70.24095241330000761, -25.02007459860000083 ) ) ;
#16111=DIRECTION ( 'NONE',  ( -6.123031769110000420E-17, 0.000000000000000000, 1.000000000000000000 ) ) ;
#16114=CARTESIAN_POINT ( 'NONE',  ( -39.54203581779999865, -73.97629583739998793, -7.314380513039999698 ) ) ;
#16116=EDGE_CURVE ( 'NONE', #4525, #10505, #21753, .T. ) ;
#16123=CARTESIAN_POINT ( 'NONE',  ( 9.571688886909999638, -37.07368284070000186, -22.92823879609999693 ) ) ;
#16126=ORIENTED_EDGE ( 'NONE', *, *, #25804, .F. ) ;
#16128=CARTESIAN_POINT ( 'NONE',  ( 23.03829042120000281, -45.73899999920000425, 10.32398954119999956 ) ) ;
#16129=CARTESIAN_POINT ( 'NONE',  ( 11.06094107680000072, -36.00000000000000000, -21.69991213999999857 ) ) ;
#16131=CARTESIAN_POINT ( 'NONE',  ( 7.168130346672493936, -73.50999119020875128, -38.90877162602799189 ) ) ;
#16132=CARTESIAN_POINT ( 'NONE',  ( -11.18243144779999909, -57.47855601759999900, 20.51090144570000007 ) ) ;
#16135=CARTESIAN_POINT ( 'NONE',  ( -2.791011762119999684, -66.02175891730000501, -26.44799069369999955 ) ) ;
#16136=CARTESIAN_POINT ( 'NONE',  ( -14.55867152370000106, -64.24504444460001196, 22.15151623919999935 ) ) ;
#16137=ORIENTED_EDGE ( 'NONE', *, *, #28715, .T. ) ;
#16138=CARTESIAN_POINT ( 'NONE',  ( 36.32450519430000213, -74.54297176320000062, -14.86961496900000057 ) ) ;
#16139=B_SPLINE_CURVE_WITH_KNOTS ( 'NONE', 3,
 ( #25712, #9675, #687, #9537, #7528, #20919, #10643, #8620, #26129, #19702, #25851, #6009, #23525, #19556, #3561, #24074, #4114, #12557, #12836 ),
 .UNSPECIFIED., .F., .F.,
 ( 4, 2, 2, 2, 2, 2, 1, 2, 2, 4 ),
 ( 0.000000000000000000, 0.2499999999999938938, 0.3749999999999893419, 0.4374999999999886757, 0.4999999999999878986, 0.6249999999999861222, 0.6874999999999836797, 0.7187499999999837907, 0.7499999999999839018, 1.000000000000000000 ),
 .UNSPECIFIED. ) ;
#16141=CARTESIAN_POINT ( 'NONE',  ( 25.78766439909999875, -63.04983560140001231, 1.379138088530000195 ) ) ;
#16142=CARTESIAN_POINT ( 'NONE',  ( -5.679770007689999289, -74.50000000000000000, 47.25000000000000000 ) ) ;
#16145=FACE_OUTER_BOUND ( 'NONE', #21257, .T. ) ;
#16154=ORIENTED_EDGE ( 'NONE', *, *, #25951, .F. ) ;
#16155=CARTESIAN_POINT ( 'NONE',  ( 23.03829042120000281, -52.56313962710000709, 10.32398954119999956 ) ) ;
#16158=CARTESIAN_POINT ( 'NONE',  ( -12.11470824010000058, -19.46971262549999793, 19.05681609440000202 ) ) ;
#16159=CARTESIAN_POINT ( 'NONE',  ( -11.79008835590000004, -62.95225063429998613, -23.26928841850000040 ) ) ;
#16160=DIRECTION ( 'NONE',  ( 0.2588190451029837025, 0.000000000000000000, -0.9659258262889443003 ) ) ;
#16161=DIRECTION ( 'NONE',  ( 3.383536836950000192E-16, 0.000000000000000000, -1.000000000000000000 ) ) ;
#16164=DIRECTION ( 'NONE',  ( -0.7071067811865457964, 0.000000000000000000, -0.7071067811865492381 ) ) ;
#16166=CARTESIAN_POINT ( 'NONE',  ( -13.16051759379999986, -19.41822420549999961, 19.76723058829999857 ) ) ;
#16170=EDGE_LOOP ( 'NONE', ( #23279, #16883, #28606, #15816, #11348 ) ) ;
#16172=CARTESIAN_POINT ( 'NONE',  ( -10.48904628653374793, -19.47230014276397370, -20.17613036516116409 ) ) ;
#16174=CARTESIAN_POINT ( 'NONE',  ( -10.47740691559999959, -19.48537698630000037, -21.16038778040000068 ) ) ;
#16175=DIRECTION ( 'NONE',  ( 0.000000000000000000, 1.000000000000000000, 0.000000000000000000 ) ) ;
#16177=CARTESIAN_POINT ( 'NONE',  ( -32.75733295119999866, -79.93903531290000331, -22.41678657819999998 ) ) ;
#16180=ORIENTED_EDGE ( 'NONE', *, *, #8631, .T. ) ;
#16187=CIRCLE ( 'NONE', #28274, 0.5000000000000027756 ) ;
#16189=CARTESIAN_POINT ( 'NONE',  ( -19.42841453280000152, -39.32886505740000160, 13.99550717529999844 ) ) ;
#16191=LINE ( 'NONE', #27142, #13576 ) ;
#16192=CARTESIAN_POINT ( 'NONE',  ( -14.91714650195326186, -74.40777954432446961, 36.29798897348343445 ) ) ;
#16193=EDGE_CURVE ( 'NONE', #8180, #9163, #6269, .T. ) ;
#16194=CARTESIAN_POINT ( 'NONE',  ( 25.14693906469999973, -65.07443093669999712, -0.3759466479219999990 ) ) ;
#16195=CIRCLE ( 'NONE', #19904, 3.749999999999996447 ) ;
#16196=VERTEX_POINT ( 'NONE', #12951 ) ;
#16198=CARTESIAN_POINT ( 'NONE',  ( 21.65402597960000008, -37.28545205309999488, -8.393872059200001345 ) ) ;
#16200=ORIENTED_EDGE ( 'NONE', *, *, #4198, .F. ) ;
#16202=CARTESIAN_POINT ( 'NONE',  ( 7.627404847670000265, -18.50000000000000000, -19.58026728520000148 ) ) ;
#16203=TOROIDAL_SURFACE ( 'NONE', #19909, 10.50000000000000000, 0.5000000000000000000 ) ;
#16205=CARTESIAN_POINT ( 'NONE',  ( -18.14849333036523760, -18.49999996075505848, 11.13143091276801044 ) ) ;
#16207=CARTESIAN_POINT ( 'NONE',  ( 8.980667191809999395, -36.11584072189999972, -20.70603881730000140 ) ) ;
#16210=CARTESIAN_POINT ( 'NONE',  ( -39.86740956975740602, -73.89318255927805978, 7.248796347619867575 ) ) ;
#16214=CARTESIAN_POINT ( 'NONE',  ( -2.166872423674899739, -19.47370675684711472, -22.73566057691103381 ) ) ;
#16216=CARTESIAN_POINT ( 'NONE',  ( -2.041929835609999966, -39.34784663180000308, -23.26788540500000124 ) ) ;
#16220=DIRECTION ( 'NONE',  ( 1.000000000000000000, 0.000000000000000000, 0.000000000000000000 ) ) ;
#16221=CARTESIAN_POINT ( 'NONE',  ( 22.17287314020000011, -57.47832541620000057, -7.362282719720000479 ) ) ;
#16223=SPHERICAL_SURFACE ( 'NONE', #24383, 2.000000000000000000 ) ;
#16224=VERTEX_POINT ( 'NONE', #20521 ) ;
#16227=CARTESIAN_POINT ( 'NONE',  ( -32.83566817450000030, -79.50000000000000000, -22.22906645670000003 ) ) ;
#16230=CARTESIAN_POINT ( 'NONE',  ( -14.22861622210000121, -68.06112402509999981, 22.55404109870000084 ) ) ;
#16231=CARTESIAN_POINT ( 'NONE',  ( 7.828355059359999757, -35.91213417740000580, -21.38475576599999783 ) ) ;
#16232=CARTESIAN_POINT ( 'NONE',  ( 36.32249705850000510, -79.79205832529999043, -14.87545865919999954 ) ) ;
#16233=CARTESIAN_POINT ( 'NONE',  ( -0.8452062098759994813, -52.63280639819944184, -23.17863372589996729 ) ) ;
#16236=EDGE_CURVE ( 'NONE', #21652, #1569, #22082, .T. ) ;
#16241=DIRECTION ( 'NONE',  ( 1.000000000000000000, 0.000000000000000000, 0.000000000000000000 ) ) ;
#16245=CIRCLE ( 'NONE', #3690, 19.99999999999999645 ) ;
#16249=CIRCLE ( 'NONE', #3694, 25.14975229270000057 ) ;
#16250=CARTESIAN_POINT ( 'NONE',  ( 47.25000000000000000, -79.00000000000000000, -6.875000000000000000 ) ) ;
#16253=CARTESIAN_POINT ( 'NONE',  ( -14.35888481029999930, -74.08594823550001252, 36.31399993319999453 ) ) ;
#16254=CARTESIAN_POINT ( 'NONE',  ( -21.35785820959999981, -65.07443093669999712, 13.27974662679999973 ) ) ;
#16257=CARTESIAN_POINT ( 'NONE',  ( -12.12177392010000077, -71.84927287379998972, -25.80509671639999780 ) ) ;
#16258=CARTESIAN_POINT ( 'NONE',  ( 8.988997220999999982, -34.66800423669999276, -19.43643757559999941 ) ) ;
#16259=DIRECTION ( 'NONE',  ( 0.5503273727321511544, 0.000000000000000000, 0.8349489701902315097 ) ) ;
#16260=DIRECTION ( 'NONE',  ( -0.7071067811865474617, 0.000000000000000000, 0.7071067811865474617 ) ) ;
#16261=CARTESIAN_POINT ( 'NONE',  ( -38.70548920639999579, -73.81415963839999961, -7.196176986149999344 ) ) ;
#16265=AXIS2_PLACEMENT_3D ( 'NONE', #27798, #27940, #28465 ) ;
#16266=CARTESIAN_POINT ( 'NONE',  ( -1.156004284370000024, -57.47571004099999925, -23.39939383540000151 ) ) ;
#16270=VERTEX_POINT ( 'NONE', #13397 ) ;
#16271=EDGE_CURVE ( 'NONE', #13154, #21711, #24578, .T. ) ;
#16272=CARTESIAN_POINT ( 'NONE',  ( 36.70830968599999977, -79.25000000000000000, -15.25000000000000000 ) ) ;
#16274=CARTESIAN_POINT ( 'NONE',  ( 46.69678069119999719, -74.07637432209999417, -3.237587372219999704 ) ) ;
#16276=CARTESIAN_POINT ( 'NONE',  ( 7.244980372382691769, -74.16605908736325148, -40.26982517619838831 ) ) ;
#16277=CARTESIAN_POINT ( 'NONE',  ( -12.24789267329999909, -65.07443093669999712, 21.96586363990000024 ) ) ;
#16279=ORIENTED_EDGE ( 'NONE', *, *, #9091, .T. ) ;
#16281=CARTESIAN_POINT ( 'NONE',  ( 46.25000000000000000, -79.00000000000000000, -13.75000000000000000 ) ) ;
#16282=CARTESIAN_POINT ( 'NONE',  ( -2.417371786180000370, -65.72572872239999242, -25.90137666380000070 ) ) ;
#16283=EDGE_CURVE ( 'NONE', #12443, #15684, #23551, .T. ) ;
#16284=AXIS2_PLACEMENT_3D ( 'NONE', #12024, #3444, #7819 ) ;
#16285=CARTESIAN_POINT ( 'NONE',  ( -15.68772883089999937, -69.50482905820000212, 23.03878850240000276 ) ) ;
#16286=EDGE_LOOP ( 'NONE', ( #5239, #21823, #10440, #4660 ) ) ;
#16288=VECTOR ( 'NONE', #8373, 1000.000000000000000 ) ;
#16289=CARTESIAN_POINT ( 'NONE',  ( -14.59919365920000089, -79.49999999012054275, 36.80099835649999562 ) ) ;
#16291=DIRECTION ( 'NONE',  ( 0.000000000000000000, -1.000000000000000000, 0.000000000000000000 ) ) ;
#16292=CARTESIAN_POINT ( 'NONE',  ( 36.28164458690000060, -74.50000000000000000, -14.97346873880000118 ) ) ;
#16295=CARTESIAN_POINT ( 'NONE',  ( -1.565549855109999777, -18.61786835250000038, -21.74208210369999961 ) ) ;
#16299=CARTESIAN_POINT ( 'NONE',  ( 22.94569809939999772, -61.52579421249999569, 10.37789087800000054 ) ) ;
#16300=CARTESIAN_POINT ( 'NONE',  ( 34.06016921999999880, -74.00000000000000000, -4.978042818679999648 ) ) ;
#16302=DIRECTION ( 'NONE',  ( 0.4794255386042040601, 0.000000000000000000, 0.8775825618903720926 ) ) ;
#16303=ORIENTED_EDGE ( 'NONE', *, *, #20063, .T. ) ;
#16304=CARTESIAN_POINT ( 'NONE',  ( 47.25000000000000000, -79.00000000000000000, -7.718270467189999824E-13 ) ) ;
#16305=CARTESIAN_POINT ( 'NONE',  ( -12.11761160510000046, -19.16174953630000033, 19.04753198859999941 ) ) ;
#16308=CARTESIAN_POINT ( 'NONE',  ( 23.73263625450000092, -64.92652906329999496, -8.873745374080000303 ) ) ;
#16310=CIRCLE ( 'NONE', #13018, 0.5000000000000004441 ) ;
#16311=ORIENTED_EDGE ( 'NONE', *, *, #27465, .T. ) ;
#16312=CIRCLE ( 'NONE', #2366, 8.999999999999998224 ) ;
#16313=DIRECTION ( 'NONE',  ( 0.01673171000360159852, -0.9993908270190947629, 0.03062718972490289376 ) ) ;
#16318=ADVANCED_FACE ( 'NONE', ( #3464 ), #2925, .T. ) ;
#16320=ADVANCED_FACE ( 'NONE', ( #21947 ), #21513, .F. ) ;
#16321=ORIENTED_EDGE ( 'NONE', *, *, #15617, .F. ) ;
#16322=CARTESIAN_POINT ( 'NONE',  ( 39.23631979950000215, -73.50064222359999633, 7.229366192799999702 ) ) ;
#16323=CARTESIAN_POINT ( 'NONE',  ( -10.81241633620959774, -19.46574764917406242, -19.41094217333082383 ) ) ;
#16325=CARTESIAN_POINT ( 'NONE',  ( -10.00361297630000124, -18.62004679909999894, -20.76967538030000071 ) ) ;
#16328=ADVANCED_FACE ( 'NONE', ( #2135 ), #20709, .T. ) ;
#16332=CARTESIAN_POINT ( 'NONE',  ( 46.25000000000000000, -74.00000000000000000, -13.75000000000000000 ) ) ;
#16333=ORIENTED_EDGE ( 'NONE', *, *, #11904, .T. ) ;
#16336=CARTESIAN_POINT ( 'NONE',  ( -19.81272040990000249, -52.63293862049999916, 12.05498172269999912 ) ) ;
#16337=DIRECTION ( 'NONE',  ( -0.3687499999999814260, 0.000000000000000000, 0.9295286103719527793 ) ) ;
#16338=ORIENTED_EDGE ( 'NONE', *, *, #6470, .T. ) ;
#16339=AXIS2_PLACEMENT_3D ( 'NONE', #2454, #15679, #4625 ) ;
#16342=CARTESIAN_POINT ( 'NONE',  ( -19.29069590680000346, -45.99312545570000310, 12.83330259409999918 ) ) ;
#16345=CARTESIAN_POINT ( 'NONE',  ( -14.85724926008588120, -74.31785917165720434, 36.29292894000464997 ) ) ;
#16347=CARTESIAN_POINT ( 'NONE',  ( 26.08584741079999958, -65.97406652829999985, 1.199274931579999981 ) ) ;
#16349=EDGE_LOOP ( 'NONE', ( #28425, #13934, #3359, #27065 ) ) ;
#16350=CARTESIAN_POINT ( 'NONE',  ( 36.70830968599999977, -79.25000000000000000, -14.75000000000000000 ) ) ;
#16354=AXIS2_PLACEMENT_3D ( 'NONE', #10666, #19859, #20010 ) ;
#16355=CARTESIAN_POINT ( 'NONE',  ( 7.215414233289999757, -74.50000000000000000, 40.70731707320000226 ) ) ;
#16359=AXIS2_PLACEMENT_3D ( 'NONE', #15264, #15572, #24182 ) ;
#16361=DIRECTION ( 'NONE',  ( 5.788992577199957397E-17, 0.000000000000000000, -1.000000000000000000 ) ) ;
#16363=ORIENTED_EDGE ( 'NONE', *, *, #23619, .T. ) ;
#16365=CARTESIAN_POINT ( 'NONE',  ( -39.34253424958686907, -73.62781383917049993, 7.220129148632251415 ) ) ;
#16368=VERTEX_POINT ( 'NONE', #9399 ) ;
#16369=CARTESIAN_POINT ( 'NONE',  ( -2.442775742550781448, -19.48034373447696765, -23.15154483919690165 ) ) ;
#16371=CARTESIAN_POINT ( 'NONE',  ( -2.440432358250000267, -32.69575302460000188, -23.63442551149999815 ) ) ;
#16374=DIRECTION ( 'NONE',  ( 1.000000000000000000, 0.000000000000000000, 8.881784197000000500E-17 ) ) ;
#16375=CARTESIAN_POINT ( 'NONE',  ( 23.29174250550000025, -49.04525650219999733, -9.486381418089997908 ) ) ;
#16377=CARTESIAN_POINT ( 'NONE',  ( -1.776356839399999804E-15, -80.50000000000000000, 3.552713678799999214E-14 ) ) ;
#16381=CARTESIAN_POINT ( 'NONE',  ( -32.65351228499999792, -74.41869006989999491, -21.85723935310000243 ) ) ;
#16382=CARTESIAN_POINT ( 'NONE',  ( -32.69645379630000548, -79.50000000000076739, -21.71458329359999695 ) ) ;
#16383=CARTESIAN_POINT ( 'NONE',  ( -14.19188855770000046, -80.00000000000000000, 37.13021410070000883 ) ) ;
#16384=CARTESIAN_POINT ( 'NONE',  ( 20.95510892579999762, -35.33620225780000368, -8.408939989400000314 ) ) ;
#16386=DIRECTION ( 'NONE',  ( 1.000000000000000000, 0.000000000000000000, 0.000000000000000000 ) ) ;
#16387=CARTESIAN_POINT ( 'NONE',  ( 21.24216623919999947, -36.23976085479999654, -9.027383814959998531 ) ) ;
#16392=SURFACE_STYLE_FILL_AREA ( #7535 ) ;
#16396=AXIS2_PLACEMENT_3D ( 'NONE', #10458, #6549, #28394 ) ;
#16397=DIRECTION ( 'NONE',  ( 0.000000000000000000, -1.000000000000000000, 0.000000000000000000 ) ) ;
#16399=EDGE_CURVE ( 'NONE', #7945, #3493, #3912, .T. ) ;
#16400=B_SPLINE_CURVE_WITH_KNOTS ( 'NONE', 3,
 ( #9391, #20473, #253, #7083, #390, #836 ),
 .UNSPECIFIED., .F., .F.,
 ( 4, 2, 4 ),
 ( 0.000000000000000000, 0.5000000000000000000, 1.000000000000000000 ),
 .UNSPECIFIED. ) ;
#16402=B_SPLINE_CURVE_WITH_KNOTS ( 'NONE', 5,
 ( #27265, #625, #5534, #13846, #16469, #20714 ),
 .UNSPECIFIED., .F., .F.,
 ( 6, 6 ),
 ( 0.000000000000000000, 6.855861996820000748 ),
 .UNSPECIFIED. ) ;
#16403=CARTESIAN_POINT ( 'NONE',  ( -7.250077434679999655, -74.05347990799999991, 40.00006844429999830 ) ) ;
#16405=CARTESIAN_POINT ( 'NONE',  ( -7.243843118864345954, -74.18716007590187189, -40.29875214189355859 ) ) ;
#16406=CARTESIAN_POINT ( 'NONE',  ( -21.69477569840000086, -66.11096492830000670, 13.63249283160000047 ) ) ;
#16408=B_SPLINE_SURFACE_WITH_KNOTS ( 'NONE', 4, 5, ( 
 ( #1282, #19040, #28066, #8102, #16991, #8946, #24409, #28758, #8655 ),
 ( #21935, #13317, #15346, #26169, #6193, #15063, #4302, #4445, #19736 ),
 ( #15648, #10827, #8797, #4009, #6785, #23972, #28623, #24551, #12867 ),
 ( #26312, #6335, #26596, #8519, #26453, #21784, #1837, #17710, #22221 ),
 ( #10680, #11111, #24262, #10966, #24115, #17560, #15499, #13022, #2268 ) ),
 .UNSPECIFIED., .F., .F., .F.,
 ( 5, 5 ),
 ( 6, 3, 6 ),
 ( 0.000000000000000000, 6.855861996759999855 ),
 ( 0.000000000000000000, 1.000000000000000000, 2.000000000000000000 ),
 .UNSPECIFIED. ) ;
#16410=CARTESIAN_POINT ( 'NONE',  ( 0.000000000000000000, -42.50000000000000000, 0.000000000000000000 ) ) ;
#16411=CARTESIAN_POINT ( 'NONE',  ( 8.516252544429999460, -25.51643856499999785, -20.42955993270000192 ) ) ;
#16412=DIRECTION ( 'NONE',  ( 0.000000000000000000, 0.000000000000000000, 1.000000000000000000 ) ) ;
#16413=DIRECTION ( 'NONE',  ( 1.000000000000000000, 0.000000000000000000, 0.000000000000000000 ) ) ;
#16420=CARTESIAN_POINT ( 'NONE',  ( -1.450026333500000097, -57.90606206700000058, -23.52488548770000065 ) ) ;
#16423=ORIENTED_EDGE ( 'NONE', *, *, #19109, .T. ) ;
#16424=EDGE_CURVE ( 'NONE', #2868, #2641, #11723, .T. ) ;
#16425=CIRCLE ( 'NONE', #5737, 0.4999999999999967804 ) ;
#16427=FACE_OUTER_BOUND ( 'NONE', #17782, .T. ) ;
#16428=FACE_OUTER_BOUND ( 'NONE', #2663, .T. ) ;
#16429=ORIENTED_EDGE ( 'NONE', *, *, #18744, .T. ) ;
#16430=CARTESIAN_POINT ( 'NONE',  ( 7.244343739429285556, -74.17816432833343754, -40.28633210784942520 ) ) ;
#16431=CARTESIAN_POINT ( 'NONE',  ( -11.38279485941639635, -60.73290390095194624, 20.83642922985102075 ) ) ;
#16432=B_SPLINE_CURVE_WITH_KNOTS ( 'NONE', 5,
 ( #11647, #27703, #771, #5260, #3224, #9616 ),
 .UNSPECIFIED., .F., .F.,
 ( 6, 6 ),
 ( 0.000000000000000000, 1.000000000000000000 ),
 .UNSPECIFIED. ) ;
#16434=CARTESIAN_POINT ( 'NONE',  ( -14.60044964929999978, -79.81260323630000642, 36.96978765280000090 ) ) ;
#16437=CARTESIAN_POINT ( 'NONE',  ( -2.513036490069999740, -70.69114014160000181, -27.60015579919999951 ) ) ;
#16438=AXIS2_PLACEMENT_3D ( 'NONE', #8177, #14996, #10613 ) ;
#16439=CARTESIAN_POINT ( 'NONE',  ( -14.17294541280000075, -69.11954792669999392, 22.97751744570000199 ) ) ;
#16440=VERTEX_POINT ( 'NONE', #13325 ) ;
#16443=CARTESIAN_POINT ( 'NONE',  ( 25.32712258629999980, -57.40875702469999453, 1.379782075540000097 ) ) ;
#16444=CARTESIAN_POINT ( 'NONE',  ( -21.27071965929999564, -64.35840737889999730, 15.42050345319999849 ) ) ;
#16445=ORIENTED_EDGE ( 'NONE', *, *, #13809, .F. ) ;
#16447=CARTESIAN_POINT ( 'NONE',  ( -2.657761925540000014, -19.49504784870000051, -24.02235578410000372 ) ) ;
#16450=CARTESIAN_POINT ( 'NONE',  ( -13.93182733059999912, -18.50000000000000000, 19.17753782289999975 ) ) ;
#16454=CARTESIAN_POINT ( 'NONE',  ( 8.986258411359999698, -35.50000000000000000, -19.49544327779999975 ) ) ;
#16456=CARTESIAN_POINT ( 'NONE',  ( -3.669439427402429121, -72.55114739963670445, -28.40640588287540069 ) ) ;
#16457=ORIENTED_EDGE ( 'NONE', *, *, #4606, .T. ) ;
#16462=CARTESIAN_POINT ( 'NONE',  ( 9.334872109610000362E-16, -74.00000000000000000, -2.419703924680000090E-15 ) ) ;
#16463=EDGE_LOOP ( 'NONE', ( #15004, #11106, #19036, #13516 ) ) ;
#16464=CARTESIAN_POINT ( 'NONE',  ( -14.71190774867310047, -74.49999999999998579, 36.44656183965725660 ) ) ;
#16465=CARTESIAN_POINT ( 'NONE',  ( 47.07637643990781129, -74.27648884675060970, -1.578698681290582106 ) ) ;
#16468=ORIENTED_EDGE ( 'NONE', *, *, #22851, .F. ) ;
#16469=CARTESIAN_POINT ( 'NONE',  ( -2.582553463740000055, -56.43963366239999857, -25.20892743809999814 ) ) ;
#16473=CARTESIAN_POINT ( 'NONE',  ( 40.70731707320000226, -74.50000000000000000, 7.215414233289999757 ) ) ;
#16477=CARTESIAN_POINT ( 'NONE',  ( 46.81085661582252300, -79.82853832540322969, -3.128125291494992410 ) ) ;
#16479=CARTESIAN_POINT ( 'NONE',  ( -32.70621743230000078, -79.83488737980000849, -22.19846261920000074 ) ) ;
#16483=ORIENTED_EDGE ( 'NONE', *, *, #25330, .T. ) ;
#16484=AXIS2_PLACEMENT_3D ( 'NONE', #9627, #20728, #787 ) ;
#16485=DIRECTION ( 'NONE',  ( -0.7414456417930912480, 0.000000000000000000, -0.6710129359900827151 ) ) ;
#16487=ORIENTED_EDGE ( 'NONE', *, *, #6604, .F. ) ;
#16490=DIRECTION ( 'NONE',  ( 0.7414456417930908039, 0.000000000000000000, 0.6710129359900831592 ) ) ;
#16493=EDGE_CURVE ( 'NONE', #7301, #10820, #717, .T. ) ;
#16494=CARTESIAN_POINT ( 'NONE',  ( 23.00257633000000013, -58.88644793239999586, -9.320358454550000005 ) ) ;
#16497=CARTESIAN_POINT ( 'NONE',  ( -38.08875739639999836, -74.50000000000000000, 9.476764215410000247 ) ) ;
#16500=EDGE_LOOP ( 'NONE', ( #23188, #5490, #12455, #7986 ) ) ;
#16502=CARTESIAN_POINT ( 'NONE',  ( 19.72252123670000401, -35.98036830730000446, -9.327645202300001159 ) ) ;
#16505=CARTESIAN_POINT ( 'NONE',  ( -3.807886452449999570, -80.00000000000000000, 46.75000000000000000 ) ) ;
#16508=CIRCLE ( 'NONE', #8110, 3.500000000000003109 ) ;
#16510=DIRECTION ( 'NONE',  ( 0.000000000000000000, -1.000000000000000000, 0.000000000000000000 ) ) ;
#16515=CARTESIAN_POINT ( 'NONE',  ( 26.62370195360000125, -72.37489743489999228, 10.79038948700000056 ) ) ;
#16519=CARTESIAN_POINT ( 'NONE',  ( 20.20034866289999798, -19.47487085739999912, -8.528768463580000514 ) ) ;
#16522=DIRECTION ( 'NONE',  ( 0.9704142011833033488, 0.000000000000000000, -0.2414462220490755373 ) ) ;
#16525=CARTESIAN_POINT ( 'NONE',  ( 22.71123055929999879, -49.06719615680000146, -9.238026508709999973 ) ) ;
#16530=CARTESIAN_POINT ( 'NONE',  ( -32.68577570540000465, -74.40224539360001188, -21.72078879429999887 ) ) ;
#16533=EDGE_CURVE ( 'NONE', #2786, #20017, #5036, .T. ) ;
#16535=CARTESIAN_POINT ( 'NONE',  ( 9.038647664420000893, -35.72724364799999819, -19.55068599180000177 ) ) ;
#16536=CARTESIAN_POINT ( 'NONE',  ( 36.44456167670000468, -80.16838065170000505, -14.57571988100000127 ) ) ;
#16537=AXIS2_PLACEMENT_3D ( 'NONE', #19309, #27543, #1828 ) ;
#16538=B_SPLINE_CURVE_WITH_KNOTS ( 'NONE', 5,
 ( #2057, #26375, #15270, #12663, #22008, #10897 ),
 .UNSPECIFIED., .F., .F.,
 ( 6, 6 ),
 ( 0.000000000000000000, 1.000000000000000000 ),
 .UNSPECIFIED. ) ;
#16543=ORIENTED_EDGE ( 'NONE', *, *, #6726, .T. ) ;
#16544=CARTESIAN_POINT ( 'NONE',  ( 32.97008024890000399, -74.00000000000000000, -20.36016474349999683 ) ) ;
#16545=CARTESIAN_POINT ( 'NONE',  ( -12.19871226703897804, -59.03921358009454678, -19.98711032788098763 ) ) ;
#16549=CARTESIAN_POINT ( 'NONE',  ( -7.462548272780000325, -74.10728787440000076, 39.37382359230000617 ) ) ;
#16550=CARTESIAN_POINT ( 'NONE',  ( -10.00000000000000000, -19.00000000000000000, 1.224606353819999829E-15 ) ) ;
#16552=DIRECTION ( 'NONE',  ( 0.000000000000000000, 1.000000000000000000, 0.000000000000000000 ) ) ;
#16553=CARTESIAN_POINT ( 'NONE',  ( 25.25824993130000351, -73.10684313109999266, -29.82725550210000165 ) ) ;
#16556=CARTESIAN_POINT ( 'NONE',  ( 0.000000000000000000, -18.50000000000000000, 0.000000000000000000 ) ) ;
#16558=DIRECTION ( 'NONE',  ( 0.000000000000000000, -1.000000000000000000, 0.000000000000000000 ) ) ;
#16561=EDGE_CURVE ( 'NONE', #27225, #13659, #17419, .T. ) ;
#16565=CARTESIAN_POINT ( 'NONE',  ( -0.5421338679160000451, -57.91805294160000273, -23.37022173519999768 ) ) ;
#16566=CARTESIAN_POINT ( 'NONE',  ( 10.42651188819999852, -36.18510625669999570, -22.68565687619999949 ) ) ;
#16570=ORIENTED_EDGE ( 'NONE', *, *, #18432, .F. ) ;
#16573=ORIENTED_EDGE ( 'NONE', *, *, #5182, .T. ) ;
#16576=CARTESIAN_POINT ( 'NONE',  ( -11.23686253208929919, -59.05314867388291589, 20.60269805518056074 ) ) ;
#16579=CARTESIAN_POINT ( 'NONE',  ( -3.236746276329999894, -71.55793241529998738, -28.02041562209999981 ) ) ;
#16580=CARTESIAN_POINT ( 'NONE',  ( 32.75000000000000000, -73.50000000000000000, -2.303043639999999983E-16 ) ) ;
#16581=ORIENTED_EDGE ( 'NONE', *, *, #21870, .F. ) ;
#16584=CARTESIAN_POINT ( 'NONE',  ( 26.46311779310000034, -64.24504203739999753, 1.532421101449999989 ) ) ;
#16586=ORIENTED_EDGE ( 'NONE', *, *, #20660, .T. ) ;
#16589=CARTESIAN_POINT ( 'NONE',  ( -3.651945809410000354, -18.50000000000000000, -23.59378895079999694 ) ) ;
#16594=DIRECTION ( 'NONE',  ( 0.000000000000000000, -1.000000000000000000, 0.000000000000000000 ) ) ;
#16596=CARTESIAN_POINT ( 'NONE',  ( 36.59060436630000623, -79.19020236199999374, -14.75000000000000000 ) ) ;
#16599=CARTESIAN_POINT ( 'NONE',  ( -12.15229178470000093, -18.85738388180000058, 18.91927663179999897 ) ) ;
#16600=CARTESIAN_POINT ( 'NONE',  ( -0.8893110448141080537, -79.83729532519589611, 47.19525132417524560 ) ) ;
#16602=CARTESIAN_POINT ( 'NONE',  ( -14.61042918459367357, -74.50000000000000000, 36.68561768139541357 ) ) ;
#16603=CARTESIAN_POINT ( 'NONE',  ( 47.25000000000000000, -75.00000000000000000, -1.242228542250000064E-12 ) ) ;
#16605=CARTESIAN_POINT ( 'NONE',  ( -13.34665425529999894, -19.40595393460000295, 20.06920644170000045 ) ) ;
#16606=ORIENTED_EDGE ( 'NONE', *, *, #993, .T. ) ;
#16608=DIRECTION ( 'NONE',  ( 1.000000000000000000, 0.000000000000000000, 0.000000000000000000 ) ) ;
#16610=CARTESIAN_POINT ( 'NONE',  ( 39.92825895559999339, -74.14144493690000104, 7.283540599280000194 ) ) ;
#16611=DIRECTION ( 'NONE',  ( 0.000000000000000000, 1.000000000000000000, 0.000000000000000000 ) ) ;
#16612=CARTESIAN_POINT ( 'NONE',  ( -11.62982413452877317, -61.04161776321530652, -22.93818510518001830 ) ) ;
#16613=DIRECTION ( 'NONE',  ( 1.000000000000000000, 0.000000000000000000, 0.000000000000000000 ) ) ;
#16615=CARTESIAN_POINT ( 'NONE',  ( -32.54924051920000494, -80.01920155719999173, -22.21939872999999821 ) ) ;
#16620=CARTESIAN_POINT ( 'NONE',  ( -2.271147603640000234, -79.96785398299999770, 47.05359239509999725 ) ) ;
#16621=CARTESIAN_POINT ( 'NONE',  ( -12.76533973971643476, -68.20220985960887106, -23.31270125210677335 ) ) ;
#16622=ORIENTED_EDGE ( 'NONE', *, *, #21838, .T. ) ;
#16624=B_SPLINE_CURVE_WITH_KNOTS ( 'NONE', 3,
 ( #9883, #23166, #14271, #897 ),
 .UNSPECIFIED., .F., .F.,
 ( 4, 4 ),
 ( 0.000000000000000000, 1.000000000000000000 ),
 .UNSPECIFIED. ) ;
#16627=CARTESIAN_POINT ( 'NONE',  ( 31.27011777710000118, -74.10309036889998424, -23.59316291639999719 ) ) ;
#16628=CARTESIAN_POINT ( 'NONE',  ( -16.85275212698199709, -72.18744872196315043, 23.44936106519583774 ) ) ;
#16630=CARTESIAN_POINT ( 'NONE',  ( 25.42047192209999906, -65.65894985479999946, 0.2065551165869999872 ) ) ;
#16631=CARTESIAN_POINT ( 'NONE',  ( -10.85837829980000002, -19.46429346509999903, 19.17438121190000189 ) ) ;
#16632=EDGE_LOOP ( 'NONE', ( #4388, #11208, #6117, #28788 ) ) ;
#16633=CARTESIAN_POINT ( 'NONE',  ( 20.37615251160000085, -53.60206220650000120, 11.14673842929999914 ) ) ;
#16634=CARTESIAN_POINT ( 'NONE',  ( -41.00000000000000000, -84.50000000000000000, -10.20110288159999890 ) ) ;
#16636=CARTESIAN_POINT ( 'NONE',  ( 20.21146652389999687, -35.98398933269999844, -9.285965084309999895 ) ) ;
#16640=B_SPLINE_SURFACE_WITH_KNOTS ( 'NONE', 5, 5, ( 
 ( #6835, #24760, #2621, #15146, #24054, #4493 ),
 ( #13368, #15699, #13673, #9002, #2474, #26106 ),
 ( #19538, #24605, #4796, #22272, #22578, #28281 ),
 ( #17910, #6132, #444, #2320, #15999, #21591 ),
 ( #13519, #11470, #20086, #22428, #11328, #15005 ),
 ( #28426, #20375, #9294, #18196, #20233, #27091 ) ),
 .UNSPECIFIED., .F., .F., .F.,
 ( 6, 6 ),
 ( 6, 6 ),
 ( 2.788355763089999773, 6.107000906349999703 ),
 ( 0.000000000000000000, 0.5000000000000000000 ),
 .UNSPECIFIED. ) ;
#16643=CARTESIAN_POINT ( 'NONE',  ( -17.93028678539999987, -18.50000000000000000, 10.99759328500000066 ) ) ;
#16644=CARTESIAN_POINT ( 'NONE',  ( 9.357772773659998933, -44.87455296190000098, -22.87094945020000125 ) ) ;
#16645=DIRECTION ( 'NONE',  ( 1.000000000000000000, 0.000000000000000000, 1.224606353820001308E-16 ) ) ;
#16646=ORIENTED_EDGE ( 'NONE', *, *, #2860, .T. ) ;
#16647=ADVANCED_FACE ( 'NONE', ( #22349 ), #73, .F. ) ;
#16648=CARTESIAN_POINT ( 'NONE',  ( -39.39373284327518832, -73.64797963447830398, 7.224658177534047709 ) ) ;
#16652=CARTESIAN_POINT ( 'NONE',  ( 19.17432176879999872, -18.50000000000000000, -8.311993326940001481 ) ) ;
#16653=EDGE_CURVE ( 'NONE', #27454, #22316, #22792, .T. ) ;
#16655=CARTESIAN_POINT ( 'NONE',  ( -2.557496217909999814, -32.68478243010000028, -23.95624216479999902 ) ) ;
#16656=DIRECTION ( 'NONE',  ( 1.000000000000000000, 0.000000000000000000, 0.000000000000000000 ) ) ;
#16657=EDGE_CURVE ( 'NONE', #25992, #7997, #9211, .T. ) ;
#16658=CARTESIAN_POINT ( 'NONE',  ( -38.71641004229999794, -73.50000000000000000, 7.135467526410000261 ) ) ;
#16661=CARTESIAN_POINT ( 'NONE',  ( -38.62788938250000115, -74.00000000000000000, -7.627566167509999495 ) ) ;
#16662=CARTESIAN_POINT ( 'NONE',  ( -10.69289422250000143, -27.02040600870000020, -21.42405574569999871 ) ) ;
#16663=ORIENTED_EDGE ( 'NONE', *, *, #7469, .F. ) ;
#16670=CARTESIAN_POINT ( 'NONE',  ( 7.218875474177777640, -73.62261561668250920, 39.32889484839974870 ) ) ;
#16672=CARTESIAN_POINT ( 'NONE',  ( 40.00000000000000000, -69.00000000000000000, 3.566319567039999839E-15 ) ) ;
#16674=EDGE_LOOP ( 'NONE', ( #17595, #13729, #15683, #2564, #7486, #4863, #27409, #24264, #11141, #18476, #14262, #28383, #2830, #2913, #7117, #27635, #28311, #11353, #20992, #14468, #9654, #2274, #26118, #22600, #15271, #14239, #27975, #17084, #18323, #5583, #18940, #4976, #27014, #25108, #3377, #10926, #4408 ) ) ;
#16675=CARTESIAN_POINT ( 'NONE',  ( 30.67829226190271186, -74.17388968317500542, -24.28831386657427416 ) ) ;
#16678=ORIENTED_EDGE ( 'NONE', *, *, #6094, .F. ) ;
#16682=CARTESIAN_POINT ( 'NONE',  ( -7.378478634080000376, -74.05312334699999610, 39.40347957289999670 ) ) ;
#16683=DIRECTION ( 'NONE',  ( -0.4047940155640055160, 0.000000000000000000, 0.9144078985680119676 ) ) ;
#16686=CARTESIAN_POINT ( 'NONE',  ( 20.35087214540000033, -74.00000000000000000, -32.65606037229999714 ) ) ;
#16690=CARTESIAN_POINT ( 'NONE',  ( -13.76821744699999961, -50.22312506960000178, 21.09213694800000027 ) ) ;
#16692=CARTESIAN_POINT ( 'NONE',  ( 7.734541327699999691, -19.43020093410000015, -20.63024918810000230 ) ) ;
#16693=CARTESIAN_POINT ( 'NONE',  ( -17.79218750000000071, -74.00000000000000000, 44.84975545040000355 ) ) ;
#16695=VERTEX_POINT ( 'NONE', #11249 ) ;
#16696=CARTESIAN_POINT ( 'NONE',  ( 10.20110288159999890, -74.50000000000000000, 41.00000000000000000 ) ) ;
#16697=B_SPLINE_CURVE_WITH_KNOTS ( 'NONE', 3,
 ( #16661, #18723, #25556, #27620, #14338, #20619, #27471, #18575 ),
 .UNSPECIFIED., .F., .F.,
 ( 4, 2, 2, 4 ),
 ( 0.000000000000000000, 0.2499999999999987788, 0.4999999999999975575, 1.000000000000000000 ),
 .UNSPECIFIED. ) ;
#16698=ORIENTED_EDGE ( 'NONE', *, *, #19034, .F. ) ;
#16701=CIRCLE ( 'NONE', #15753, 0.5000000000000004441 ) ;
#16702=CARTESIAN_POINT ( 'NONE',  ( 10.59598273719999995, -36.06131723410000234, -22.18468985750000044 ) ) ;
#16704=CARTESIAN_POINT ( 'NONE',  ( 37.60355029590000697, -84.00000000000000000, 9.356041104380000917 ) ) ;
#16705=AXIS2_PLACEMENT_3D ( 'NONE', #5890, #21767, #14904 ) ;
#16706=AXIS2_PLACEMENT_3D ( 'NONE', #15817, #2003, #10844 ) ;
#16708=CARTESIAN_POINT ( 'NONE',  ( -20.03576987106655238, -32.72519964002148640, 14.54909399142346160 ) ) ;
#16709=VECTOR ( 'NONE', #20792, 1000.000000000000000 ) ;
#16714=EDGE_LOOP ( 'NONE', ( #12569, #2720, #21855, #5571 ) ) ;
#16716=CARTESIAN_POINT ( 'NONE',  ( 9.046504331389998654, -35.76492331110000578, -19.84904996739999916 ) ) ;
#16717=EDGE_CURVE ( 'NONE', #8180, #7391, #17882, .T. ) ;
#16719=EDGE_CURVE ( 'NONE', #12333, #26756, #14464, .T. ) ;
#16720=CARTESIAN_POINT ( 'NONE',  ( -22.05955109964234495, -74.01432994044633062, -32.14328720598611255 ) ) ;
#16725=CARTESIAN_POINT ( 'NONE',  ( 24.03655833510000051, -62.10499660389999832, 0.01904210411250000304 ) ) ;
#16726=CARTESIAN_POINT ( 'NONE',  ( -19.90875640260000168, -60.57913428290000013, 12.83012088510000126 ) ) ;
#16727=VERTEX_POINT ( 'NONE', #9516 ) ;
#16728=AXIS2_PLACEMENT_3D ( 'NONE', #2291, #120, #16412 ) ;
#16730=CARTESIAN_POINT ( 'NONE',  ( -3.351256578809999720, -18.50000000000000000, -24.02084876199999997 ) ) ;
#16731=CARTESIAN_POINT ( 'NONE',  ( 36.75634433000346490, -74.48625131260783405, -14.60844170371495210 ) ) ;
#16732=ORIENTED_EDGE ( 'NONE', *, *, #1278, .F. ) ;
#16734=AXIS2_PLACEMENT_3D ( 'NONE', #28146, #8181, #17067 ) ;
#16736=CARTESIAN_POINT ( 'NONE',  ( 36.69050691090000527, -80.32091633570000511, -13.94376034409999932 ) ) ;
#16737=CARTESIAN_POINT ( 'NONE',  ( 36.72991148340000223, -74.73026516779999895, -14.71529450729999944 ) ) ;
#16741=CARTESIAN_POINT ( 'NONE',  ( -0.8115734779096079876, -79.80847618003535615, 47.20451980215236887 ) ) ;
#16743=CARTESIAN_POINT ( 'NONE',  ( 46.75000000000000000, -69.00000000000000000, 4.603792064249999600E-16 ) ) ;
#16750=AXIS2_PLACEMENT_3D ( 'NONE', #14684, #12216, #3759 ) ;
#16755=CARTESIAN_POINT ( 'NONE',  ( 46.91594090715152277, -79.74893011108233054, -2.749115903323809729 ) ) ;
#16761=FACE_OUTER_BOUND ( 'NONE', #6137, .T. ) ;
#16763=CARTESIAN_POINT ( 'NONE',  ( -0.7692311531319999673, -79.63780243000000780, 47.25012955910000301 ) ) ;
#16767=DIRECTION ( 'NONE',  ( 0.4794255386042036715, 0.000000000000000000, 0.8775825618903724257 ) ) ;
#16775=CARTESIAN_POINT ( 'NONE',  ( -6.705637591229999472, -74.00000000000000000, 33.51864961869999604 ) ) ;
#16776=ORIENTED_EDGE ( 'NONE', *, *, #7944, .T. ) ;
#16777=CARTESIAN_POINT ( 'NONE',  ( -40.28633210810852461, -74.17816432860024634, -7.244343739419030648 ) ) ;
#16778=B_SPLINE_CURVE_WITH_KNOTS ( 'NONE', 5,
 ( #27789, #870, #20957, #16708, #13798, #22703 ),
 .UNSPECIFIED., .F., .F.,
 ( 6, 6 ),
 ( 0.000000000000000000, 1.000000000000000000 ),
 .UNSPECIFIED. ) ;
#16779=CARTESIAN_POINT ( 'NONE',  ( 21.75765532779999845, -37.94971352660000008, -8.412785021810000430 ) ) ;
#16789=DIRECTION ( 'NONE',  ( 0.7071067811865475727, 0.000000000000000000, 0.7071067811865475727 ) ) ;
#16791=AXIS2_PLACEMENT_3D ( 'NONE', #10071, #14192, #7506 ) ;
#16794=VECTOR ( 'NONE', #22706, 1000.000000000000000 ) ;
#16798=CARTESIAN_POINT ( 'NONE',  ( 23.08916810359999872, -41.88175146140000038, -9.424942062580001334 ) ) ;
#16799=ORIENTED_EDGE ( 'NONE', *, *, #11843, .F. ) ;
#16802=CARTESIAN_POINT ( 'NONE',  ( -14.16028365999999927, -74.03779068149999887, 36.32206337349999359 ) ) ;
#16805=CARTESIAN_POINT ( 'NONE',  ( -1.328852201560088764, -74.17182873519007558, 47.12723346842092553 ) ) ;
#16808=CARTESIAN_POINT ( 'NONE',  ( 7.010390260919999428E-15, -79.00000000000000000, 36.25000000000000000 ) ) ;
#16809=CARTESIAN_POINT ( 'NONE',  ( 20.57008619019999784, -58.79569603810000444, 11.24574726549999859 ) ) ;
#16810=EDGE_LOOP ( 'NONE', ( #14930, #8539, #19481, #6160, #26800, #17291, #26760, #19171 ) ) ;
#16811=EDGE_CURVE ( 'NONE', #23252, #17023, #14803, .T. ) ;
#16813=CARTESIAN_POINT ( 'NONE',  ( 47.17407167555492720, -74.61367352086737981, -1.124626421616047534 ) ) ;
#16818=DIRECTION ( 'NONE',  ( 0.000000000000000000, 1.000000000000000000, 0.000000000000000000 ) ) ;
#16820=B_SPLINE_CURVE_WITH_KNOTS ( 'NONE', 3,
 ( #2798, #15885, #13554, #11652, #7167, #24938, #7018, #22462, #20412, #15731, #2505, #20117, #24644, #8880, #4831, #16033, #11360, #22755, #483, #9326, #4524, #20263, #4673 ),
 .UNSPECIFIED., .F., .F.,
 ( 4, 2, 2, 1, 1, 2, 2, 2, 1, 1, 1, 2, 2, 4 ),
 ( 0.000000000000000000, 0.1249999999999429623, 0.1874999999999153177, 0.2187499999999028555, 0.2343749999998963329, 0.2421874999998903932, 0.2499999999998844813, 0.3749999999998625544, 0.4374999999998507860, 0.4687499999998409606, 0.4843749999998399614, 0.4921874999998397948, 0.4999999999998395728, 1.000000000000000000 ),
 .UNSPECIFIED. ) ;
#16823=DIRECTION ( 'NONE',  ( 0.000000000000000000, 1.000000000000000000, 0.000000000000000000 ) ) ;
#16826=CARTESIAN_POINT ( 'NONE',  ( 20.98512250110000110, -28.53090651930000021, -7.691805548749999666 ) ) ;
#16831=ORIENTED_EDGE ( 'NONE', *, *, #1523, .F. ) ;
#16832=CARTESIAN_POINT ( 'NONE',  ( 7.215414233289999757, -74.50000000000000000, -40.70731707320000226 ) ) ;
#16836=CIRCLE ( 'NONE', #28000, 0.5000000000000004441 ) ;
#16837=CARTESIAN_POINT ( 'NONE',  ( 23.65471649550000066, -72.84996959090000246, -30.57903112150000169 ) ) ;
#16841=CARTESIAN_POINT ( 'NONE',  ( -18.63062389896092341, -19.46426558511086569, 11.76718335430204299 ) ) ;
#16843=DIRECTION ( 'NONE',  ( 0.4794255386042036160, 0.000000000000000000, 0.8775825618903723147 ) ) ;
#16844=ORIENTED_EDGE ( 'NONE', *, *, #12974, .T. ) ;
#16845=CARTESIAN_POINT ( 'NONE',  ( -10.61287167059999881, -19.46510050329999686, 19.30934957549999709 ) ) ;
#16846=ORIENTED_EDGE ( 'NONE', *, *, #7558, .F. ) ;
#16848=EDGE_CURVE ( 'NONE', #12521, #10474, #2102, .T. ) ;
#16849=CARTESIAN_POINT ( 'NONE',  ( -0.9714544087850000009, -64.02328494229999478, -24.65515989760000082 ) ) ;
#16850=CARTESIAN_POINT ( 'NONE',  ( 9.393614098460000505, -37.68584072819999875, -22.97877291129999833 ) ) ;
#16853=AXIS2_PLACEMENT_3D ( 'NONE', #27149, #8755, #17674 ) ;
#16855=EDGE_CURVE ( 'NONE', #3210, #10257, #23947, .T. ) ;
#16856=CARTESIAN_POINT ( 'NONE',  ( 19.19205617106166883, -19.49520357620059130, -9.000935570425328436 ) ) ;
#16859=CARTESIAN_POINT ( 'NONE',  ( -7.250053749315869212, -74.39269056244653200, -40.35493623770417315 ) ) ;
#16861=CARTESIAN_POINT ( 'NONE',  ( 8.386162616670347347, -68.18701404723893233, -25.21061241927545638 ) ) ;
#16862=CARTESIAN_POINT ( 'NONE',  ( 7.913872602619999697, -36.43558290860000426, -21.40167476739999941 ) ) ;
#16863=CARTESIAN_POINT ( 'NONE',  ( 22.26662627820000040, -57.47855601759999900, -7.066909182079999852 ) ) ;
#16865=CARTESIAN_POINT ( 'NONE',  ( -18.97570897180000316, -18.50000000000000000, 15.16944231589999958 ) ) ;
#16866=ORIENTED_EDGE ( 'NONE', *, *, #6039, .T. ) ;
#16869=CARTESIAN_POINT ( 'NONE',  ( -32.11921425309235190, -74.01249333572259559, -22.05455054358708011 ) ) ;
#16873=CIRCLE ( 'NONE', #21091, 22.03370205219999889 ) ;
#16877=CARTESIAN_POINT ( 'NONE',  ( 18.91112499396685465, -18.62337005498731912, -8.654031818350992111 ) ) ;
#16879=ORIENTED_EDGE ( 'NONE', *, *, #14277, .F. ) ;
#16881=CARTESIAN_POINT ( 'NONE',  ( 8.988996100299999625, -34.66800400750000222, -19.43643858049999906 ) ) ;
#16882=CARTESIAN_POINT ( 'NONE',  ( 36.31537122139999951, -79.49793013650000262, -14.89204469480000093 ) ) ;
#16883=ORIENTED_EDGE ( 'NONE', *, *, #15229, .T. ) ;
#16885=CARTESIAN_POINT ( 'NONE',  ( 36.76353006592368899, -79.41291915633111387, -14.66093257292968310 ) ) ;
#16887=CARTESIAN_POINT ( 'NONE',  ( -0.8571442907775489450, -79.82540267843101844, 47.19917229225826816 ) ) ;
#16889=ORIENTED_EDGE ( 'NONE', *, *, #12479, .F. ) ;
#16892=AXIS2_PLACEMENT_3D ( 'NONE', #7607, #22900, #27122 ) ;
#16895=CIRCLE ( 'NONE', #5744, 1.000000000000000222 ) ;
#16899=CARTESIAN_POINT ( 'NONE',  ( -21.60034897659999942, -79.81702851609999527, -32.77174746360000057 ) ) ;
#16900=CARTESIAN_POINT ( 'NONE',  ( -11.62450342175550055, -60.96820961890185231, -22.92682159015150134 ) ) ;
#16901=CARTESIAN_POINT ( 'NONE',  ( 25.40476796700415107, -67.67676320189275430, 10.87793065395078074 ) ) ;
#16907=CARTESIAN_POINT ( 'NONE',  ( -2.491468434920000252, -55.00753887619999460, -24.55868524289999755 ) ) ;
#16909=VERTEX_POINT ( 'NONE', #5452 ) ;
#16912=DIRECTION ( 'NONE',  ( 0.000000000000000000, 1.000000000000000000, 0.000000000000000000 ) ) ;
#16914=CARTESIAN_POINT ( 'NONE',  ( -14.25438161831525363, -74.03830041542175877, 36.24026857307444516 ) ) ;
#16916=ADVANCED_FACE ( 'NONE', ( #822 ), #11700, .T. ) ;
#16918=EDGE_CURVE ( 'NONE', #19506, #8148, #14652, .T. ) ;
#16919=EDGE_LOOP ( 'NONE', ( #13288, #20798, #21241, #14900 ) ) ;
#16921=CARTESIAN_POINT ( 'NONE',  ( 21.34788073790000240, -35.28814185829999417, -7.426814485570000457 ) ) ;
#16923=CARTESIAN_POINT ( 'NONE',  ( 41.00000000000000000, -80.50000000000000000, -10.20110288159999890 ) ) ;
#16924=DIRECTION ( 'NONE',  ( 1.000000000000000000, 0.000000000000000000, 0.000000000000000000 ) ) ;
#16935=DIRECTION ( 'NONE',  ( 0.000000000000000000, -1.000000000000000000, 0.000000000000000000 ) ) ;
#16936=VERTEX_POINT ( 'NONE', #20905 ) ;
#16938=ADVANCED_FACE ( 'NONE', ( #20615 ), #18857, .F. ) ;
#16939=FACE_OUTER_BOUND ( 'NONE', #3988, .T. ) ;
#16940=CARTESIAN_POINT ( 'NONE',  ( 25.62591688519999877, -71.82672919469999329, 11.84408135179999988 ) ) ;
#16943=CARTESIAN_POINT ( 'NONE',  ( -14.10481785270000010, -74.02367878169998505, 36.45432549239999531 ) ) ;
#16944=CARTESIAN_POINT ( 'NONE',  ( 25.26718046270000073, -19.50000000000000000, 6.129403842640000377 ) ) ;
#16946=DIRECTION ( 'NONE',  ( 0.000000000000000000, 1.000000000000000000, 0.000000000000000000 ) ) ;
#16947=ORIENTED_EDGE ( 'NONE', *, *, #15812, .F. ) ;
#16949=DIRECTION ( 'NONE',  ( 0.7071067811865475727, 0.000000000000000000, 0.7071067811865475727 ) ) ;
#16950=B_SPLINE_CURVE_WITH_KNOTS ( 'NONE', 3,
 ( #1674, #8624, #3567, #25858 ),
 .UNSPECIFIED., .F., .F.,
 ( 4, 4 ),
 ( 0.000000000000000000, 1.000000000000000000 ),
 .UNSPECIFIED. ) ;
#16951=CARTESIAN_POINT ( 'NONE',  ( 8.664772570080000236, -60.49464403009999813, -22.56734825659999899 ) ) ;
#16952=CARTESIAN_POINT ( 'NONE',  ( -39.07223452339999170, -73.87252278329999911, -7.323177335889999640 ) ) ;
#16953=CARTESIAN_POINT ( 'NONE',  ( 23.15286878230000056, -57.80430419099999995, 10.38290477119999977 ) ) ;
#16955=VERTEX_POINT ( 'NONE', #9810 ) ;
#16956=EDGE_CURVE ( 'NONE', #3048, #25813, #7067, .T. ) ;
#16961=DIRECTION ( 'NONE',  ( 1.000000000000000000, 0.000000000000000000, 0.000000000000000000 ) ) ;
#16966=CARTESIAN_POINT ( 'NONE',  ( -1.598721155459999804E-14, -84.00000000000000000, 7.105427357599999217E-15 ) ) ;
#16967=CARTESIAN_POINT ( 'NONE',  ( -17.94180966909999597, -74.00000000000000000, 18.81731824139999887 ) ) ;
#16968=EDGE_LOOP ( 'NONE', ( #15056, #25755, #15384, #33 ) ) ;
#16973=EDGE_CURVE ( 'NONE', #28710, #17905, #18280, .T. ) ;
#16974=CARTESIAN_POINT ( 'NONE',  ( -7.250938816910000639, -73.85300527940000848, 39.81408737849999824 ) ) ;
#16976=CARTESIAN_POINT ( 'NONE',  ( 9.334872109610000362E-16, -74.00000000000000000, -2.419703924680000090E-15 ) ) ;
#16979=DIRECTION ( 'NONE',  ( 1.000000000000000000, 0.000000000000000000, 0.000000000000000000 ) ) ;
#16982=CARTESIAN_POINT ( 'NONE',  ( -18.59805086797023321, -19.47341637985122631, 13.22102611671206240 ) ) ;
#16983=CARTESIAN_POINT ( 'NONE',  ( 7.793340607010000198, -34.75995359360000236, -21.18684990219999875 ) ) ;
#16985=ORIENTED_EDGE ( 'NONE', *, *, #26230, .T. ) ;
#16988=ORIENTED_EDGE ( 'NONE', *, *, #13728, .T. ) ;
#16989=CARTESIAN_POINT ( 'NONE',  ( -2.080583965950000280, -64.78279487710000240, -25.39005782320000293 ) ) ;
#16991=CARTESIAN_POINT ( 'NONE',  ( -19.51583823489999858, -52.61368720150000655, 13.56962763329999966 ) ) ;
#16992=ORIENTED_EDGE ( 'NONE', *, *, #26119, .F. ) ;
#16993=B_SPLINE_CURVE_WITH_KNOTS ( 'NONE', 5,
 ( #4051, #23735, #25926, #17036, #28240, #21273 ),
 .UNSPECIFIED., .F., .F.,
 ( 6, 6 ),
 ( 0.000000000000000000, 1.000000000000000000 ),
 .UNSPECIFIED. ) ;
#16994=CARTESIAN_POINT ( 'NONE',  ( -40.00000000000000000, -69.00000000000000000, 3.236300116779999679E-15 ) ) ;
#16995=DIRECTION ( 'NONE',  ( 1.000000000000000000, 0.000000000000000000, 0.000000000000000000 ) ) ;
#16997=DIRECTION ( 'NONE',  ( 0.9620138697098239433, 0.000000000000000000, 0.2730005759809492893 ) ) ;
#16998=ORIENTED_EDGE ( 'NONE', *, *, #5356, .T. ) ;
#17000=CARTESIAN_POINT ( 'NONE',  ( -17.48567531570000000, -18.50000000000000000, 12.33326151890000055 ) ) ;
#17001=EDGE_CURVE ( 'NONE', #26473, #27727, #9065, .T. ) ;
#17002=CARTESIAN_POINT ( 'NONE',  ( 22.13380541979999805, -19.18187901349999791, 9.708259679350000226 ) ) ;
#17003=CARTESIAN_POINT ( 'NONE',  ( -15.42363691649999957, -67.46051717960000360, 22.84488648889999851 ) ) ;
#17005=ORIENTED_EDGE ( 'NONE', *, *, #9744, .T. ) ;
#17006=CARTESIAN_POINT ( 'NONE',  ( -1.776356839399999804E-15, -89.50000000000000000, 0.000000000000000000 ) ) ;
#17009=CARTESIAN_POINT ( 'NONE',  ( -7.227961103978413959, -73.66549258102378417, 39.43512252455204248 ) ) ;
#17011=ORIENTED_EDGE ( 'NONE', *, *, #2998, .T. ) ;
#17012=ADVANCED_FACE ( 'NONE', ( #23228 ), #28021, .T. ) ;
#17013=AXIS2_PLACEMENT_3D ( 'NONE', #7164, #16030, #20717 ) ;
#17014=FACE_OUTER_BOUND ( 'NONE', #19089, .T. ) ;
#17015=CARTESIAN_POINT ( 'NONE',  ( -31.89935321680000158, -74.00000000000000000, -21.99985828019999801 ) ) ;
#17016=CARTESIAN_POINT ( 'NONE',  ( 36.68904416859999884, -80.12912447070000610, -14.08963035319999868 ) ) ;
#17017=ORIENTED_EDGE ( 'NONE', *, *, #9071, .F. ) ;
#17019=VECTOR ( 'NONE', #7321, 1000.000000000000114 ) ;
#17023=VERTEX_POINT ( 'NONE', #16658 ) ;
#17025=DIRECTION ( 'NONE',  ( 0.000000000000000000, -1.000000000000000000, 0.000000000000000000 ) ) ;
#17028=CARTESIAN_POINT ( 'NONE',  ( 9.476129726560001743, -36.00000000000000000, -20.06309461059999677 ) ) ;
#17029=DIRECTION ( 'NONE',  ( 0.4794255386042036160, 0.000000000000000000, 0.8775825618903723147 ) ) ;
#17033=CARTESIAN_POINT ( 'NONE',  ( 25.32394939313839188, -67.45391685492131728, 10.87937782985497215 ) ) ;
#17034=EDGE_LOOP ( 'NONE', ( #12271, #6265, #9702, #20126 ) ) ;
#17036=CARTESIAN_POINT ( 'NONE',  ( 25.57918037516483523, -64.69849890637429723, 1.120748866632130580 ) ) ;
#17041=DIRECTION ( 'NONE',  ( 0.6710129359900831592, 0.000000000000000000, -0.7414456417930911369 ) ) ;
#17042=CARTESIAN_POINT ( 'NONE',  ( -12.05824591346449459, -67.66818470673190689, -24.37625945436767694 ) ) ;
#17047=CARTESIAN_POINT ( 'NONE',  ( 38.62788938250000115, -74.00000000000000000, 7.627566167509999495 ) ) ;
#17048=CARTESIAN_POINT ( 'NONE',  ( 8.969779973459999667, -35.75711592580000087, -20.13916512639999823 ) ) ;
#17049=CARTESIAN_POINT ( 'NONE',  ( 25.25824993130000351, -73.10684313109999266, -29.82725550210000165 ) ) ;
#17053=CARTESIAN_POINT ( 'NONE',  ( 21.43077048929999862, -35.81319862919999508, -7.299949289889999804 ) ) ;
#17055=CARTESIAN_POINT ( 'NONE',  ( 21.46039065680000135, -36.43422328669999644, -7.619628857949999556 ) ) ;
#17057=EDGE_LOOP ( 'NONE', ( #1155, #8003, #25343, #7680, #19770, #6750, #26031, #17183, #14384 ) ) ;
#17059=DIRECTION ( 'NONE',  ( -1.000000000000000000, -0.000000000000000000, -1.738658080640000114E-17 ) ) ;
#17060=CARTESIAN_POINT ( 'NONE',  ( -0.5726204572655302361, -18.60284036877294156, -21.53722082371633917 ) ) ;
#17062=EDGE_CURVE ( 'NONE', #20989, #28649, #21188, .T. ) ;
#17063=CARTESIAN_POINT ( 'NONE',  ( 6.974892859179999682, -49.11505549650000546, -21.98941332900000134 ) ) ;
#17065=ORIENTED_EDGE ( 'NONE', *, *, #14662, .T. ) ;
#17066=ADVANCED_FACE ( 'NONE', ( #9948 ), #25371, .F. ) ;
#17067=DIRECTION ( 'NONE',  ( -0.09756097560976760563, 0.000000000000000000, -0.9952295494196654602 ) ) ;
#17069=CARTESIAN_POINT ( 'NONE',  ( 39.61603006823808215, -73.75061506092693264, 7.239953483540725543 ) ) ;
#17071=CARTESIAN_POINT ( 'NONE',  ( 18.91112499059999763, -18.62337005500000231, -8.654031818700001821 ) ) ;
#17072=DIRECTION ( 'NONE',  ( 0.000000000000000000, -1.000000000000000000, 0.000000000000000000 ) ) ;
#17073=CARTESIAN_POINT ( 'NONE',  ( -1.281139941660000225, -19.46501104069999855, -22.08267515169999839 ) ) ;
#17074=DIRECTION ( 'NONE',  ( 1.000000000000000000, 0.000000000000000000, 0.000000000000000000 ) ) ;
#17075=ORIENTED_EDGE ( 'NONE', *, *, #24416, .T. ) ;
#17079=CARTESIAN_POINT ( 'NONE',  ( 22.71963733680000175, -57.44066854489999940, -9.099149309629998683 ) ) ;
#17080=CARTESIAN_POINT ( 'NONE',  ( -38.68350846249999364, -73.93831524339999817, -7.318371247189999984 ) ) ;
#17082=AXIS2_PLACEMENT_3D ( 'NONE', #10591, #17186, #8287 ) ;
#17083=CARTESIAN_POINT ( 'NONE',  ( -10.53866346480000082, -19.41822431039999941, -21.28095825400000152 ) ) ;
#17084=ORIENTED_EDGE ( 'NONE', *, *, #5783, .T. ) ;
#17089=B_SPLINE_CURVE_WITH_KNOTS ( 'NONE', 5,
 ( #25442, #19019, #9971, #18884, #14637, #23533 ),
 .UNSPECIFIED., .F., .F.,
 ( 6, 6 ),
 ( -40.74965564189999867, -28.77371845028335073 ),
 .UNSPECIFIED. ) ;
#17090=CARTESIAN_POINT ( 'NONE',  ( 21.21808891099999883, -34.59820414320000026, -7.670974023059999425 ) ) ;
#17092=DIRECTION ( 'NONE',  ( 0.000000000000000000, 1.000000000000000000, 0.000000000000000000 ) ) ;
#17093=ORIENTED_EDGE ( 'NONE', *, *, #21446, .F. ) ;
#17096=AXIS2_PLACEMENT_3D ( 'NONE', #7939, #9968, #18739 ) ;
#17097=CARTESIAN_POINT ( 'NONE',  ( 20.65664752990000252, -31.58327036160000389, -8.509521500050000853 ) ) ;
#17101=CARTESIAN_POINT ( 'NONE',  ( -11.41594931139999858, -19.46510050329999686, -18.84569254350000023 ) ) ;
#17104=EDGE_CURVE ( 'NONE', #11916, #24358, #23506, .T. ) ;
#17108=CARTESIAN_POINT ( 'NONE',  ( 36.50549972238673035, -74.62369757142499793, -14.71598444713541021 ) ) ;
#17109=AXIS2_PLACEMENT_3D ( 'NONE', #13421, #2372, #20135 ) ;
#17111=CARTESIAN_POINT ( 'NONE',  ( -22.70539113190000080, -72.04110636640000109, 17.08947363740000114 ) ) ;
#17113=CARTESIAN_POINT ( 'NONE',  ( -19.23753200850040912, -19.48999941762926369, 14.12819559392180224 ) ) ;
#17116=CARTESIAN_POINT ( 'NONE',  ( 40.70731707320000226, -74.50000000000000000, 7.215414233289999757 ) ) ;
#17117=ORIENTED_EDGE ( 'NONE', *, *, #22270, .F. ) ;
#17118=CARTESIAN_POINT ( 'NONE',  ( 7.491375829749999937, -18.50000000000000000, -19.98345411639999725 ) ) ;
#17119=TOROIDAL_SURFACE ( 'NONE', #15714, 7.750000000000000000, 0.5000000000000000000 ) ;
#17121=CARTESIAN_POINT ( 'NONE',  ( 22.51853742080000131, -36.00000000000000000, -11.01541626720000089 ) ) ;
#17123=EDGE_CURVE ( 'NONE', #26673, #4890, #13043, .T. ) ;
#17124=CARTESIAN_POINT ( 'NONE',  ( -1.448823250100000015, -58.77396426510000538, -23.58892699440000129 ) ) ;
#17125=CARTESIAN_POINT ( 'NONE',  ( 9.214873172669999946, -37.66961404259999568, -22.49121690919999850 ) ) ;
#17130=CARTESIAN_POINT ( 'NONE',  ( -13.70187146129979183, -57.41946977618258074, 20.98050236089959952 ) ) ;
#17135=ADVANCED_FACE ( 'NONE', ( #25551 ), #18753, .T. ) ;
#17136=CIRCLE ( 'NONE', #10589, 3.499999999999999556 ) ;
#17138=CARTESIAN_POINT ( 'NONE',  ( -19.35716652280000005, -18.50000000000000000, 15.34467299940000018 ) ) ;
#17141=CARTESIAN_POINT ( 'NONE',  ( -20.45733727490000220, -60.27256034759999892, 14.77382382620000101 ) ) ;
#17144=CYLINDRICAL_SURFACE ( 'NONE', #2278, 3.749999999999996447 ) ;
#17146=CARTESIAN_POINT ( 'NONE',  ( -0.5672159954309998753, -18.50000000000000000, -21.33394993619999624 ) ) ;
#17151=CARTESIAN_POINT ( 'NONE',  ( 37.07813615679999941, -80.00739956740001446, -13.83267119569999970 ) ) ;
#17153=AXIS2_PLACEMENT_3D ( 'NONE', #16410, #5345, #18754 ) ;
#17154=ADVANCED_FACE ( 'NONE', ( #21736 ), #14216, .T. ) ;
#17157=CARTESIAN_POINT ( 'NONE',  ( -1.451021762614941979, -80.03759595315190722, 47.10371954600015698 ) ) ;
#17159=CARTESIAN_POINT ( 'NONE',  ( -40.00000000000000000, -73.00000000000000000, 2.464695114669999848E-15 ) ) ;
#17160=ORIENTED_EDGE ( 'NONE', *, *, #27284, .F. ) ;
#17161=CARTESIAN_POINT ( 'NONE',  ( 22.56940788859999714, -57.43018266629999857, 10.15711811299999923 ) ) ;
#17162=CARTESIAN_POINT ( 'NONE',  ( 7.215414233289999757, -74.50000000000000000, 40.70731707320000226 ) ) ;
#17163=ADVANCED_FACE ( 'NONE', ( #4399 ), #24427, .F. ) ;
#17164=ORIENTED_EDGE ( 'NONE', *, *, #3412, .T. ) ;
#17166=CARTESIAN_POINT ( 'NONE',  ( -3.577689640331729759, -18.50000000000000000, -25.07857796645360793 ) ) ;
#17168=VERTEX_POINT ( 'NONE', #8743 ) ;
#17170=DIRECTION ( 'NONE',  ( 0.7414446217286146945, 0.000000000000000000, 0.6710140631236514164 ) ) ;
#17172=CARTESIAN_POINT ( 'NONE',  ( -3.649267921049999863, -18.50000000000000000, -24.01816718290000097 ) ) ;
#17174=TOROIDAL_SURFACE ( 'NONE', #8778, 6.750000000000000000, 0.5000000000000000000 ) ;
#17180=CARTESIAN_POINT ( 'NONE',  ( -2.582194743379999657, -56.19735282230000450, -25.20298037470000097 ) ) ;
#17181=CARTESIAN_POINT ( 'NONE',  ( 11.37093174122694528, -72.27543338683032914, -27.00921921794252967 ) ) ;
#17183=ORIENTED_EDGE ( 'NONE', *, *, #22791, .F. ) ;
#17184=CARTESIAN_POINT ( 'NONE',  ( 9.855634485030901004, -64.48636389391205626, -24.31831199924348397 ) ) ;
#17185=CARTESIAN_POINT ( 'NONE',  ( -14.01337423630000067, -80.50000000000000000, 36.66316738249999929 ) ) ;
#17186=DIRECTION ( 'NONE',  ( 0.000000000000000000, 1.000000000000000000, 0.000000000000000000 ) ) ;
#17187=CARTESIAN_POINT ( 'NONE',  ( 18.81756521970000406, -18.50000000000000000, 9.528581421409999308 ) ) ;
#17188=CARTESIAN_POINT ( 'NONE',  ( -13.78473438695133346, -69.07614453243721186, 23.18529913744219328 ) ) ;
#17189=CARTESIAN_POINT ( 'NONE',  ( -40.00000000000000000, -74.00000000000000000, 3.466919520389999841E-15 ) ) ;
#17190=CARTESIAN_POINT ( 'NONE',  ( -11.90444329340000174, -64.24504203739999753, -23.68394282290000064 ) ) ;
#17191=CARTESIAN_POINT ( 'NONE',  ( -22.43272078519999724, -80.50000000000000000, -32.20769377289999369 ) ) ;
#17192=EDGE_CURVE ( 'NONE', #26794, #21398, #12378, .T. ) ;
#17196=CARTESIAN_POINT ( 'NONE',  ( 21.11704720389999679, -35.76753062550000095, -8.346333568960000449 ) ) ;
#17198=CARTESIAN_POINT ( 'NONE',  ( 21.08638048839999968, -36.32484399220000171, -8.697366343609999717 ) ) ;
#17204=CARTESIAN_POINT ( 'NONE',  ( -2.865017121281941748, -64.99739744814985443, -26.59911453002877124 ) ) ;
#17206=CARTESIAN_POINT ( 'NONE',  ( 9.524618309619999224, -53.22700740319999824, -23.40924512820000203 ) ) ;
#17210=CARTESIAN_POINT ( 'NONE',  ( 22.71928070270000077, -19.44965585980000000, 1.104521532629999969 ) ) ;
#17211=CARTESIAN_POINT ( 'NONE',  ( 22.41768028079999908, -65.59529275500000267, 11.91456822289999984 ) ) ;
#17214=FACE_OUTER_BOUND ( 'NONE', #28679, .T. ) ;
#17216=CARTESIAN_POINT ( 'NONE',  ( -1.604812007069718272, -64.93834275522041821, -25.19371719667666198 ) ) ;
#17218=CARTESIAN_POINT ( 'NONE',  ( 5.329070518200000398E-15, -74.50000000000000000, 0.000000000000000000 ) ) ;
#17220=CIRCLE ( 'NONE', #12106, 2.000000000000000000 ) ;
#17222=DIRECTION ( 'NONE',  ( 0.000000000000000000, -1.000000000000000000, 0.000000000000000000 ) ) ;
#17223=CARTESIAN_POINT ( 'NONE',  ( 9.577933644319998052, -58.81640545049999957, -23.56560165069999968 ) ) ;
#17226=CARTESIAN_POINT ( 'NONE',  ( 23.02633534789999814, -60.04642514249999863, 10.32969153620000213 ) ) ;
#17228=VERTEX_POINT ( 'NONE', #15151 ) ;
#17229=B_SPLINE_CURVE_WITH_KNOTS ( 'NONE', 5,
 ( #13413, #341, #26989, #9184, #24802, #13861, #18089, #4839, #13718 ),
 .UNSPECIFIED., .F., .F.,
 ( 6, 3, 6 ),
 ( 0.000000000000000000, 0.3451758947491398444, 1.000000000000000000 ),
 .UNSPECIFIED. ) ;
#17232=EDGE_CURVE ( 'NONE', #13203, #3822, #24897, .T. ) ;
#17233=DIRECTION ( 'NONE',  ( 0.000000000000000000, 1.000000000000000000, 0.000000000000000000 ) ) ;
#17239=AXIS2_PLACEMENT_3D ( 'NONE', #27856, #11835, #14590 ) ;
#17242=CARTESIAN_POINT ( 'NONE',  ( 20.94292112449999976, -31.57154123859999473, -8.118247248619999468 ) ) ;
#17246=CARTESIAN_POINT ( 'NONE',  ( -40.00000000000000000, -82.25000000000000000, 0.000000000000000000 ) ) ;
#17251=CARTESIAN_POINT ( 'NONE',  ( 21.55856599210000013, -18.50000000000000000, 0.6626745995510000542 ) ) ;
#17252=DIRECTION ( 'NONE',  ( 1.000000000000000000, 0.000000000000000000, 0.000000000000000000 ) ) ;
#17255=CARTESIAN_POINT ( 'NONE',  ( -22.76595506760000021, -72.55114968140000542, 17.38101673350000098 ) ) ;
#17257=CARTESIAN_POINT ( 'NONE',  ( -19.73459501710000197, -19.50000000000000000, 14.41863426819999994 ) ) ;
#17261=AXIS2_PLACEMENT_3D ( 'NONE', #22504, #22647, #5003 ) ;
#17264=AXIS2_PLACEMENT_3D ( 'NONE', #15121, #21289, #10189 ) ;
#17266=CIRCLE ( 'NONE', #2853, 6.749999999999999112 ) ;
#17267=ORIENTED_EDGE ( 'NONE', *, *, #24990, .T. ) ;
#17269=CARTESIAN_POINT ( 'NONE',  ( 5.326862811529999898E-15, -69.50000000000000000, -47.25000000000000000 ) ) ;
#17272=CARTESIAN_POINT ( 'NONE',  ( -1.084625078730000025, -65.04696937989999128, -25.11520914390000314 ) ) ;
#17277=ORIENTED_EDGE ( 'NONE', *, *, #10056, .F. ) ;
#17278=DIRECTION ( 'NONE',  ( -0.9295286103719511139, 0.000000000000000000, -0.3687499999999862554 ) ) ;
#17282=DIRECTION ( 'NONE',  ( 0.000000000000000000, -1.000000000000000000, 0.000000000000000000 ) ) ;
#17285=CARTESIAN_POINT ( 'NONE',  ( -22.22906645665673153, -74.41344022149685600, -32.83566817454327946 ) ) ;
#17286=CARTESIAN_POINT ( 'NONE',  ( 22.35420149509999987, -19.50000008899999671, 9.881343242109998926 ) ) ;
#17287=CARTESIAN_POINT ( 'NONE',  ( -32.58054283434451293, -74.15589285242916162, -22.16749819904017826 ) ) ;
#17288=CARTESIAN_POINT ( 'NONE',  ( -19.63525383109999822, -57.47122600979999874, 13.01113855729999891 ) ) ;
#17291=ORIENTED_EDGE ( 'NONE', *, *, #5008, .T. ) ;
#17298=CARTESIAN_POINT ( 'NONE',  ( -32.78146620020000057, -74.32000120609998817, -22.21606701669999850 ) ) ;
#17299=CARTESIAN_POINT ( 'NONE',  ( -22.39529575027539110, -79.87460703810864970, -32.76478017285002409 ) ) ;
#17300=ORIENTED_EDGE ( 'NONE', *, *, #1716, .F. ) ;
#17304=CYLINDRICAL_SURFACE ( 'NONE', #16750, 0.5000000000000012212 ) ;
#17306=ORIENTED_EDGE ( 'NONE', *, *, #11110, .T. ) ;
#17307=DIRECTION ( 'NONE',  ( 0.000000000000000000, -1.000000000000000000, 0.000000000000000000 ) ) ;
#17309=CARTESIAN_POINT ( 'NONE',  ( 20.38362048469999976, -53.84434310259999279, 11.15071595380000069 ) ) ;
#17312=ORIENTED_EDGE ( 'NONE', *, *, #4606, .F. ) ;
#17315=AXIS2_PLACEMENT_3D ( 'NONE', #15353, #24269, #4309 ) ;
#17319=CARTESIAN_POINT ( 'NONE',  ( 25.56573787435306144, -68.11428155215978109, 10.87001957151865383 ) ) ;
#17324=EDGE_CURVE ( 'NONE', #16038, #13829, #15570, .T. ) ;
#17325=DIRECTION ( 'NONE',  ( 0.4794255386042040601, 0.000000000000000000, 0.8775825618903720926 ) ) ;
#17327=CARTESIAN_POINT ( 'NONE',  ( 11.65689279962786884, -72.11966578858674382, -27.17683449633075554 ) ) ;
#17329=ORIENTED_EDGE ( 'NONE', *, *, #17432, .F. ) ;
#17334=EDGE_CURVE ( 'NONE', #5555, #15327, #2523, .T. ) ;
#17337=TOROIDAL_SURFACE ( 'NONE', #4318, 6.750000000000000000, 0.5000000000000000000 ) ;
#17339=TOROIDAL_SURFACE ( 'NONE', #146, 21.03431122519999974, 1.000000000000000000 ) ;
#17340=FACE_OUTER_BOUND ( 'NONE', #22846, .T. ) ;
#17341=ORIENTED_EDGE ( 'NONE', *, *, #1993, .T. ) ;
#17344=CARTESIAN_POINT ( 'NONE',  ( 21.52213036419999881, -37.12342612100000139, -7.869482006920000217 ) ) ;
#17348=B_SPLINE_SURFACE_WITH_KNOTS ( 'NONE', 5, 5, ( 
 ( #19230, #5687, #3644, #1073, #12508, #20868 ),
 ( #27715, #8155, #25932, #5955, #11956, #27981 ),
 ( #25516, #1334, #928, #3514, #16620, #18956 ),
 ( #14437, #12097, #23328, #1476, #14839, #27839 ),
 ( #21010, #23193, #7884, #7621, #9913, #16763 ),
 ( #25658, #12370, #7757, #14569, #23474, #21278 ) ),
 .UNSPECIFIED., .F., .F., .F.,
 ( 6, 6 ),
 ( 6, 6 ),
 ( 3.704386147560000175, 9.195309357930000260 ),
 ( 0.000000000000000000, 0.5000000000000000000 ),
 .UNSPECIFIED. ) ;
#17353=CARTESIAN_POINT ( 'NONE',  ( 9.427231679889999327, -53.23790003359999901, -23.11289036089999982 ) ) ;
#17354=LINE ( 'NONE', #23911, #10171 ) ;
#17355=DIRECTION ( 'NONE',  ( 0.000000000000000000, -1.000000000000000000, 0.000000000000000000 ) ) ;
#17356=EDGE_LOOP ( 'NONE', ( #16487, #11426, #6493, #27120 ) ) ;
#17358=CARTESIAN_POINT ( 'NONE',  ( 24.30550941250000108, -42.22519323649999734, 1.361066622060000064 ) ) ;
#17359=CARTESIAN_POINT ( 'NONE',  ( 23.10489107149999910, -66.56254540410000686, 11.55379042880000107 ) ) ;
#17363=CARTESIAN_POINT ( 'NONE',  ( -2.080583445478223936, -64.78278821048890279, -25.39005510556196654 ) ) ;
#17366=VERTEX_POINT ( 'NONE', #12648 ) ;
#17367=EDGE_CURVE ( 'NONE', #3493, #11457, #12100, .T. ) ;
#17368=DIRECTION ( 'NONE',  ( 0.000000000000000000, -1.000000000000000000, 0.000000000000000000 ) ) ;
#17370=CARTESIAN_POINT ( 'NONE',  ( 22.95932595720000080, -57.43039249360000298, -9.307783803350000440 ) ) ;
#17371=CARTESIAN_POINT ( 'NONE',  ( -12.07714908089999994, -67.83051071330000070, -24.91356169369999662 ) ) ;
#17372=EDGE_CURVE ( 'NONE', #7997, #10981, #21281, .T. ) ;
#17374=CARTESIAN_POINT ( 'NONE',  ( 24.78974499519999952, -64.24504771300000527, -10.08507930170000044 ) ) ;
#17375=ORIENTED_EDGE ( 'NONE', *, *, #5206, .T. ) ;
#17380=EDGE_LOOP ( 'NONE', ( #5624, #16303, #19720, #4473 ) ) ;
#17383=CARTESIAN_POINT ( 'NONE',  ( 7.250053749315197749, -74.39269056243638545, 40.35493623771126437 ) ) ;
#17384=ORIENTED_EDGE ( 'NONE', *, *, #1297, .F. ) ;
#17389=ORIENTED_EDGE ( 'NONE', *, *, #6138, .T. ) ;
#17392=VERTEX_POINT ( 'NONE', #14573 ) ;
#17393=CARTESIAN_POINT ( 'NONE',  ( 8.071123906760000466, -36.85053012899999914, -21.46851019590000220 ) ) ;
#17397=B_SPLINE_CURVE_WITH_KNOTS ( 'NONE', 3,
 ( #5456, #14339, #23232, #22806 ),
 .UNSPECIFIED., .F., .F.,
 ( 4, 4 ),
 ( -7.329014384030000606, -6.713731535029999975 ),
 .UNSPECIFIED. ) ;
#17398=CARTESIAN_POINT ( 'NONE',  ( 22.56104036090000164, -19.46971296670000129, 0.9632387859859999901 ) ) ;
#17399=CARTESIAN_POINT ( 'NONE',  ( -7.318371247189999984, -73.93831524339999817, 38.68350846249999364 ) ) ;
#17403=DIRECTION ( 'NONE',  ( 0.000000000000000000, -1.000000000000000000, 0.000000000000000000 ) ) ;
#17404=B_SPLINE_CURVE_WITH_KNOTS ( 'NONE', 5,
 ( #16292, #14672, #27382, #12337, #1036, #7580 ),
 .UNSPECIFIED., .F., .F.,
 ( 6, 6 ),
 ( 0.000000000000000000, 1.000000000000000000 ),
 .UNSPECIFIED. ) ;
#17407=CARTESIAN_POINT ( 'NONE',  ( 9.334872109610000362E-16, -74.00000000000000000, -2.419703924680000090E-15 ) ) ;
#17408=CARTESIAN_POINT ( 'NONE',  ( 36.28420073633509446, -75.00000019211667279, -14.96759456046001091 ) ) ;
#17411=VECTOR ( 'NONE', #25092, 1000.000000000000000 ) ;
#17416=CARTESIAN_POINT ( 'NONE',  ( 7.924293243680000209, -18.50000000000000000, -19.29218481000000196 ) ) ;
#17417=CARTESIAN_POINT ( 'NONE',  ( 21.62249394079999831, -36.00000000000000000, -10.68317415409999960 ) ) ;
#17418=CARTESIAN_POINT ( 'NONE',  ( -2.578021201719999933, -61.45046333410000017, -25.33276682509999844 ) ) ;
#17419=CIRCLE ( 'NONE', #21161, 39.25000000000000000 ) ;
#17420=B_SPLINE_CURVE_WITH_KNOTS ( 'NONE', 5,
 ( #4395, #13263, #6281, #17216, #17363, #12963, #4244, #8888, #17801 ),
 .UNSPECIFIED., .F., .F.,
 ( 6, 3, 6 ),
 ( 0.000000000000000000, 0.5000000000000000000, 1.000000000000000000 ),
 .UNSPECIFIED. ) ;
#17423=DIRECTION ( 'NONE',  ( 1.000000000000000000, 0.000000000000000000, 0.000000000000000000 ) ) ;
#17425=CARTESIAN_POINT ( 'NONE',  ( 21.19938064309999959, -34.67919421940000291, -7.731040044549999379 ) ) ;
#17429=DIRECTION ( 'NONE',  ( 0.000000000000000000, 1.000000000000000000, 0.000000000000000000 ) ) ;
#17431=CARTESIAN_POINT ( 'NONE',  ( 21.40964882759999810, -19.42987840509999842, 9.433029012200000452 ) ) ;
#17432=EDGE_CURVE ( 'NONE', #10427, #8854, #9000, .T. ) ;
#17433=CARTESIAN_POINT ( 'NONE',  ( -22.19729432756942700, -74.24324329339850692, -32.70355094814552643 ) ) ;
#17436=CARTESIAN_POINT ( 'NONE',  ( -32.71258333431942589, -74.25151540671238592, -22.19947060199589828 ) ) ;
#17439=AXIS2_PLACEMENT_3D ( 'NONE', #25699, #16949, #3823 ) ;
#17442=CARTESIAN_POINT ( 'NONE',  ( -22.83401285485959065, -72.59721320750036000, 17.30277226862465412 ) ) ;
#17444=ORIENTED_EDGE ( 'NONE', *, *, #3812, .F. ) ;
#17448=CARTESIAN_POINT ( 'NONE',  ( -32.54298110219999529, -74.18397341870000616, -22.08462029819999728 ) ) ;
#17454=ORIENTED_EDGE ( 'NONE', *, *, #21515, .F. ) ;
#17458=LINE ( 'NONE', #19772, #18594 ) ;
#17459=ORIENTED_EDGE ( 'NONE', *, *, #18934, .F. ) ;
#17460=CARTESIAN_POINT ( 'NONE',  ( 21.33676308416200129, -18.50000000000000000, -0.4490900276398021584 ) ) ;
#17461=CARTESIAN_POINT ( 'NONE',  ( -21.85457013290000106, -79.50000016359999222, -32.66023313979999187 ) ) ;
#17462=CARTESIAN_POINT ( 'NONE',  ( -2.583988331150000040, -57.40875702419999982, -25.23271569440000306 ) ) ;
#17463=CARTESIAN_POINT ( 'NONE',  ( 8.793944060959999476, -36.72282064609999708, -21.68248837259999817 ) ) ;
#17465=CARTESIAN_POINT ( 'NONE',  ( -3.641273963749999787, -18.50000000000000000, -23.80755169360000068 ) ) ;
#17468=ADVANCED_FACE ( 'NONE', ( #5556 ), #25326, .F. ) ;
#17470=CARTESIAN_POINT ( 'NONE',  ( 23.97433219293744955, -62.13475794617575332, -0.5610772764335347773 ) ) ;
#17473=DIRECTION ( 'NONE',  ( 0.000000000000000000, -1.000000000000000000, 0.000000000000000000 ) ) ;
#17474=CARTESIAN_POINT ( 'NONE',  ( 11.38494915445543754, -72.26806502549214883, -27.01670803782107910 ) ) ;
#17475=CARTESIAN_POINT ( 'NONE',  ( -18.60684769790000104, -18.50000000000000000, 14.95957231910000118 ) ) ;
#17481=CARTESIAN_POINT ( 'NONE',  ( 8.862965437350000641, -35.80913068480000305, -20.41714882420000166 ) ) ;
#17484=CARTESIAN_POINT ( 'NONE',  ( -31.64302845809999809, -74.50000000000000000, -31.64302845809999809 ) ) ;
#17490=CARTESIAN_POINT ( 'NONE',  ( 21.47403927899999587, -36.87897171440000221, -8.083288125820001113 ) ) ;
#17491=DIRECTION ( 'NONE',  ( 0.000000000000000000, -1.000000000000000000, 0.000000000000000000 ) ) ;
#17492=VERTEX_POINT ( 'NONE', #6699 ) ;
#17493=CARTESIAN_POINT ( 'NONE',  ( 8.479935047972508855, -37.33301741675911245, -21.77931238865912533 ) ) ;
#17495=ORIENTED_EDGE ( 'NONE', *, *, #3792, .F. ) ;
#17497=CARTESIAN_POINT ( 'NONE',  ( 41.00000000000000000, -84.00000000000000000, -10.20110288159999890 ) ) ;
#17499=CARTESIAN_POINT ( 'NONE',  ( -10.85800713629999947, -18.85488210659999808, -19.08173651049999719 ) ) ;
#17504=CARTESIAN_POINT ( 'NONE',  ( 22.83116343590000241, -42.27294335679999904, -0.2419517822940000229 ) ) ;
#17505=CARTESIAN_POINT ( 'NONE',  ( 22.17951941979999830, -65.07442867339999282, 11.85657634389999870 ) ) ;
#17508=CARTESIAN_POINT ( 'NONE',  ( 7.105427357599999217E-15, -69.00000000000000000, -40.00000000000000000 ) ) ;
#17510=CARTESIAN_POINT ( 'NONE',  ( 10.50000000000000000, -89.00000000000000000, -1.981748098959999875E-14 ) ) ;
#17511=ORIENTED_EDGE ( 'NONE', *, *, #23981, .T. ) ;
#17512=DIRECTION ( 'NONE',  ( 0.4794255386042036160, 0.000000000000000000, 0.8775825618903723147 ) ) ;
#17514=CARTESIAN_POINT ( 'NONE',  ( 23.52264653552683527, -74.11875716583942619, -31.20127190410864770 ) ) ;
#17515=CARTESIAN_POINT ( 'NONE',  ( -12.47539548249999974, -69.51716295290000858, -24.28999545310000130 ) ) ;
#17517=CARTESIAN_POINT ( 'NONE',  ( 22.76327770750000212, -62.13507791070000508, -7.555575355879999400 ) ) ;
#17519=CARTESIAN_POINT ( 'NONE',  ( 9.334872109610000362E-16, -74.00000000000000000, -2.419703924680000090E-15 ) ) ;
#17521=ORIENTED_EDGE ( 'NONE', *, *, #27694, .F. ) ;
#17526=ORIENTED_EDGE ( 'NONE', *, *, #27781, .T. ) ;
#17528=EDGE_CURVE ( 'NONE', #5350, #27002, #23204, .T. ) ;
#17535=DIRECTION ( 'NONE',  ( 0.5301416321220552286, 0.000000000000000000, 0.8479091047340884257 ) ) ;
#17536=EDGE_CURVE ( 'NONE', #10144, #26598, #27658, .T. ) ;
#17537=DIRECTION ( 'NONE',  ( 1.000000000000000000, 0.000000000000000000, 0.000000000000000000 ) ) ;
#17538=EDGE_CURVE ( 'NONE', #8283, #28554, #5445, .T. ) ;
#17541=CARTESIAN_POINT ( 'NONE',  ( -7.196176986149999344, -73.81415963839999961, 38.70548920639999579 ) ) ;
#17549=CARTESIAN_POINT ( 'NONE',  ( -12.13283323140000114, -67.24447298400001216, -23.70109879609999837 ) ) ;
#17550=CARTESIAN_POINT ( 'NONE',  ( 18.95948039760000015, -19.91448514760000066, -9.022805879459999900 ) ) ;
#17551=ORIENTED_EDGE ( 'NONE', *, *, #28575, .T. ) ;
#17552=CARTESIAN_POINT ( 'NONE',  ( 8.341252703189999451, -18.50000000000000000, -18.88171238309999822 ) ) ;
#17553=CARTESIAN_POINT ( 'NONE',  ( -9.356041104380000917, -84.00000000000000000, -37.60355029590000697 ) ) ;
#17554=AXIS2_PLACEMENT_3D ( 'NONE', #26422, #20294, #2388 ) ;
#17556=CARTESIAN_POINT ( 'NONE',  ( -12.91148099519999981, -61.97049086579999511, 20.77791015659999729 ) ) ;
#17558=ADVANCED_FACE ( 'NONE', ( #4209 ), #13198, .T. ) ;
#17560=CARTESIAN_POINT ( 'NONE',  ( -19.90265987359999755, -57.44036991819999827, 14.20824064939999865 ) ) ;
#17563=VERTEX_POINT ( 'NONE', #11020 ) ;
#17565=AXIS2_PLACEMENT_3D ( 'NONE', #4724, #17985, #9083 ) ;
#17566=CARTESIAN_POINT ( 'NONE',  ( 7.196176986149999344, -73.81415963839999961, -38.70548920639999579 ) ) ;
#17569=CARTESIAN_POINT ( 'NONE',  ( 7.694334339803791778, -37.39019464809554449, -21.51655577991487078 ) ) ;
#17571=CARTESIAN_POINT ( 'NONE',  ( -14.13580644329999991, -80.00000064429998758, 36.98348703120000636 ) ) ;
#17572=CARTESIAN_POINT ( 'NONE',  ( 20.39668362470000318, -32.72716367860000020, 10.02066118239999959 ) ) ;
#17573=DIRECTION ( 'NONE',  ( 1.000000000000000000, 0.000000000000000000, 0.000000000000000000 ) ) ;
#17574=AXIS2_PLACEMENT_3D ( 'NONE', #1697, #21647, #6638 ) ;
#17576=LINE ( 'NONE', #1998, #15525 ) ;
#17578=ORIENTED_EDGE ( 'NONE', *, *, #19283, .F. ) ;
#17580=DIRECTION ( 'NONE',  ( -0.6390296260299768161, 0.06995790998169656993, -0.7659941435069727023 ) ) ;
#17583=CARTESIAN_POINT ( 'NONE',  ( -7.223639776384101374, -73.64317723970496843, 39.38195712097429180 ) ) ;
#17584=CARTESIAN_POINT ( 'NONE',  ( -40.70731707320000226, -74.50000000000000000, -7.215414233289999757 ) ) ;
#17585=ORIENTED_EDGE ( 'NONE', *, *, #7384, .F. ) ;
#17586=CARTESIAN_POINT ( 'NONE',  ( 19.97576656849999921, -36.00000000000000000, -19.97576656849999921 ) ) ;
#17587=CARTESIAN_POINT ( 'NONE',  ( -32.46931817979999835, -74.16345073059999038, -21.99116898890000016 ) ) ;
#17588=CARTESIAN_POINT ( 'NONE',  ( -22.35195235113883783, -79.82938816292890749, -32.78357590675958733 ) ) ;
#17589=B_SPLINE_CURVE_WITH_KNOTS ( 'NONE', 3,
 ( #26699, #22320, #13568, #10922, #2519, #8746, #17514, #22035, #11375, #28706, #24361, #20278, #9049, #18093, #4402, #6430, #15293, #13269, #345, #6881, #10776, #19976, #7034, #199, #6740, #15900, #26994, #4844, #17953, #15604, #13723, #24503 ),
 .UNSPECIFIED., .F., .F.,
 ( 4, 2, 2, 2, 1, 1, 1, 1, 1, 2, 2, 2, 2, 1, 1, 1, 1, 1, 2, 2, 4 ),
 ( 0.000000000000000000, 0.2500000000000248690, 0.3750000000000378031, 0.4375000000000447420, 0.4687500000000484612, 0.4843750000000501821, 0.4921875000000506817, 0.4960937500000511258, 0.4980468750000515143, 0.4990234375000516254, 0.5000000000000518474, 0.6250000000000320854, 0.6875000000000219824, 0.7187500000000174305, 0.7343750000000153211, 0.7421875000000136557, 0.7460937500000127676, 0.7480468750000124345, 0.7490234375000122125, 0.7500000000000119904, 1.000000000000000000 ),
 .UNSPECIFIED. ) ;
#17590=ORIENTED_EDGE ( 'NONE', *, *, #7631, .F. ) ;
#17592=DIRECTION ( 'NONE',  ( 0.000000000000000000, -1.000000000000000000, 0.000000000000000000 ) ) ;
#17593=CARTESIAN_POINT ( 'NONE',  ( 19.61885648609999677, -35.93737992959999872, -9.235927176200000588 ) ) ;
#17595=ORIENTED_EDGE ( 'NONE', *, *, #16236, .F. ) ;
#17597=AXIS2_PLACEMENT_3D ( 'NONE', #3476, #6212, #25624 ) ;
#17598=DIRECTION ( 'NONE',  ( -0.9952295494196654602, 0.000000000000000000, 0.09756097560976760563 ) ) ;
#17602=CARTESIAN_POINT ( 'NONE',  ( 46.36824973070000055, -73.69905166609999014, -3.512760466140000037 ) ) ;
#17610=EDGE_LOOP ( 'NONE', ( #25698, #21104, #14557, #8954 ) ) ;
#17611=CARTESIAN_POINT ( 'NONE',  ( 36.38880822659999836, -73.99825405529999500, -13.96626921939999910 ) ) ;
#17617=CARTESIAN_POINT ( 'NONE',  ( -17.71392320319999669, -18.50000000000000000, 12.76655036999999915 ) ) ;
#17619=CIRCLE ( 'NONE', #19475, 1.000000000000000888 ) ;
#17624=CARTESIAN_POINT ( 'NONE',  ( 47.25000000000000000, -79.00000000000000000, -13.75000000000000000 ) ) ;
#17628=DIRECTION ( 'NONE',  ( 0.02956883857460810769, 0.000000000000000000, 0.9995627462972741517 ) ) ;
#17630=CARTESIAN_POINT ( 'NONE',  ( -11.22183587500000002, -57.45864773929999814, -21.12541641649999846 ) ) ;
#17633=ADVANCED_FACE ( 'NONE', ( #8704 ), #18347, .T. ) ;
#17636=EDGE_LOOP ( 'NONE', ( #28085, #1906, #10490, #13445 ) ) ;
#17637=CARTESIAN_POINT ( 'NONE',  ( -13.46276276179999876, -19.49999999970000175, 20.39865906480000035 ) ) ;
#17639=ORIENTED_EDGE ( 'NONE', *, *, #15571, .F. ) ;
#17644=VERTEX_POINT ( 'NONE', #26507 ) ;
#17646=CARTESIAN_POINT ( 'NONE',  ( 9.476764215410000247, -84.00000000000000000, -38.08875739639999836 ) ) ;
#17652=CARTESIAN_POINT ( 'NONE',  ( 22.53098139629999963, -27.06313850649999964, 0.4808225629529999656 ) ) ;
#17653=CARTESIAN_POINT ( 'NONE',  ( -14.81587592385739605, -80.00394138637977903, 36.34631758749846853 ) ) ;
#17656=CYLINDRICAL_SURFACE ( 'NONE', #8075, 7.249999999999999112 ) ;
#17659=CARTESIAN_POINT ( 'NONE',  ( 26.61465604159999998, -68.28989644159999273, 0.1578853838729999959 ) ) ;
#17660=ADVANCED_FACE ( 'NONE', ( #24320 ), #2918, .T. ) ;
#17661=AXIS2_PLACEMENT_3D ( 'NONE', #14871, #3410, #1781 ) ;
#17663=CARTESIAN_POINT ( 'NONE',  ( 9.564508935660001043, -57.40875689140000304, -23.52622281860000086 ) ) ;
#17665=CARTESIAN_POINT ( 'NONE',  ( -11.22008224870000070, -57.43018267659999765, -22.06025767750000099 ) ) ;
#17667=CIRCLE ( 'NONE', #15298, 39.25000000000000000 ) ;
#17669=CARTESIAN_POINT ( 'NONE',  ( 22.13628285440143983, -57.47600047054346817, -7.675802460420446671 ) ) ;
#17672=EDGE_CURVE ( 'NONE', #14960, #27229, #4847, .T. ) ;
#17674=DIRECTION ( 'NONE',  ( 1.000000000000000000, 0.000000000000000000, 0.000000000000000000 ) ) ;
#17678=PLANE ( 'NONE',  #14757 ) ;
#17681=CARTESIAN_POINT ( 'NONE',  ( 8.154778043900000384, -36.28970872960000094, -21.27812994379999978 ) ) ;
#17683=CIRCLE ( 'NONE', #8364, 32.39999999999999858 ) ;
#17686=CARTESIAN_POINT ( 'NONE',  ( 46.25000000000000000, -75.00000000000000000, -13.75000000000000000 ) ) ;
#17687=DIRECTION ( 'NONE',  ( 0.7678754814159409747, 0.000000000000000000, -0.6405991297529499695 ) ) ;
#17689=CARTESIAN_POINT ( 'NONE',  ( -13.46276276189999876, -19.18584073440000282, 20.39865906470000212 ) ) ;
#17690=DIRECTION ( 'NONE',  ( 0.2414462220490755373, 0.000000000000000000, 0.9704142011833033488 ) ) ;
#17692=EDGE_CURVE ( 'NONE', #19989, #23575, #23897, .T. ) ;
#17700=CARTESIAN_POINT ( 'NONE',  ( 8.810535018830000453, -19.17198326990000012, -19.82299369949999956 ) ) ;
#17701=CARTESIAN_POINT ( 'NONE',  ( 22.51363372970000043, -36.53914150059999599, -9.828880634039999009 ) ) ;
#17705=ORIENTED_EDGE ( 'NONE', *, *, #1297, .T. ) ;
#17707=CARTESIAN_POINT ( 'NONE',  ( -12.17169857430000057, -60.55460316730000159, 20.45714472730000111 ) ) ;
#17708=CARTESIAN_POINT ( 'NONE',  ( 7.215414233289999757, -74.50000000000000000, 40.70731707320000226 ) ) ;
#17710=CARTESIAN_POINT ( 'NONE',  ( -20.27744904749999932, -56.20810645120000260, 14.66966877139999959 ) ) ;
#17711=B_SPLINE_CURVE_WITH_KNOTS ( 'NONE', 5,
 ( #3629, #9644, #14821, #5295, #23725, #12488 ),
 .UNSPECIFIED., .F., .F.,
 ( 6, 6 ),
 ( 0.000000000000000000, 1.000000000000000000 ),
 .UNSPECIFIED. ) ;
#17712=CARTESIAN_POINT ( 'NONE',  ( 38.57396449699999863, -80.50000000000000000, -9.597487326430000465 ) ) ;
#17713=CARTESIAN_POINT ( 'NONE',  ( 20.63161943080000071, -19.46510050319999863, -7.734358783100000245 ) ) ;
#17718=EDGE_LOOP ( 'NONE', ( #22482, #17705 ) ) ;
#17722=CARTESIAN_POINT ( 'NONE',  ( 19.55467021020000118, -26.09744228899999996, 10.64706777249999980 ) ) ;
#17723=AXIS2_PLACEMENT_3D ( 'NONE', #3512, #25655, #25513 ) ;
#17726=CIRCLE ( 'NONE', #20048, 34.89999999999999858 ) ;
#17727=TOROIDAL_SURFACE ( 'NONE', #1023, 30.50381168839999901, 2.000000000000000000 ) ;
#17729=CARTESIAN_POINT ( 'NONE',  ( 10.65559738969999870, -67.35763218280000331, -25.86638506229999734 ) ) ;
#17733=CARTESIAN_POINT ( 'NONE',  ( 8.996935515640000602, -29.61190174099999695, -19.27470341220000094 ) ) ;
#17734=CARTESIAN_POINT ( 'NONE',  ( -7.249922261819999214, -74.00000000000000000, 40.03357376379999977 ) ) ;
#17737=ADVANCED_FACE ( 'NONE', ( #7140 ), #12277, .T. ) ;
#17738=DIRECTION ( 'NONE',  ( -0.000000000000000000, 1.000000000000000000, 0.000000000000000000 ) ) ;
#17739=CARTESIAN_POINT ( 'NONE',  ( -32.34497379209999934, -74.07302383969998516, -22.05334043340000250 ) ) ;
#17742=ADVANCED_FACE ( 'NONE', ( #9150 ), #3205, .F. ) ;
#17744=CIRCLE ( 'NONE', #5192, 7.250000000000000000 ) ;
#17747=EDGE_LOOP ( 'NONE', ( #8291, #19622 ) ) ;
#17750=CARTESIAN_POINT ( 'NONE',  ( 8.408333318189998979E-15, -74.00000000000000000, 40.00000000000000000 ) ) ;
#17755=CARTESIAN_POINT ( 'NONE',  ( 21.08559791559969554, -57.47122622298945060, 10.49905601409981237 ) ) ;
#17759=ORIENTED_EDGE ( 'NONE', *, *, #25573, .T. ) ;
#17762=CARTESIAN_POINT ( 'NONE',  ( -22.04294097380000039, -74.04477437299999565, -32.27064897399999666 ) ) ;
#17763=CARTESIAN_POINT ( 'NONE',  ( -2.355531086969999688, -56.22908209860000284, -24.30570137699999833 ) ) ;
#17765=DIRECTION ( 'NONE',  ( 0.000000000000000000, 1.000000000000000000, 0.000000000000000000 ) ) ;
#17766=VECTOR ( 'NONE', #23194, 1000.000000000000000 ) ;
#17768=CARTESIAN_POINT ( 'NONE',  ( 7.627566167509999495, -74.00000000000000000, -38.62788938250000115 ) ) ;
#17770=VERTEX_POINT ( 'NONE', #15055 ) ;
#17772=CARTESIAN_POINT ( 'NONE',  ( 7.727581852389999284, -65.07443093669999712, -23.93312597839999967 ) ) ;
#17773=CARTESIAN_POINT ( 'NONE',  ( -12.09704001540000107, -77.00000000000000000, 47.10905722069999513 ) ) ;
#17777=EDGE_CURVE ( 'NONE', #17228, #26695, #2993, .T. ) ;
#17779=FACE_OUTER_BOUND ( 'NONE', #23233, .T. ) ;
#17780=ORIENTED_EDGE ( 'NONE', *, *, #10852, .T. ) ;
#17782=EDGE_LOOP ( 'NONE', ( #2559, #9569, #18025, #15630 ) ) ;
#17783=DIRECTION ( 'NONE',  ( 0.000000000000000000, -1.000000000000000000, 0.000000000000000000 ) ) ;
#17789=CARTESIAN_POINT ( 'NONE',  ( 22.29340633682235762, -27.06771711593788154, -0.5094401308349546520 ) ) ;
#17792=CARTESIAN_POINT ( 'NONE',  ( -10.67495457480000098, -18.61783141309999934, -18.91245961079999915 ) ) ;
#17793=CARTESIAN_POINT ( 'NONE',  ( 47.21754643642892546, -79.25383175836481087, -0.8707321872798817752 ) ) ;
#17796=CARTESIAN_POINT ( 'NONE',  ( 23.08853106659999810, -49.87553805839999654, -0.5737624632769999788 ) ) ;
#17799=EDGE_LOOP ( 'NONE', ( #43, #1005, #3497, #4058, #16363 ) ) ;
#17801=CARTESIAN_POINT ( 'NONE',  ( -2.790536503729999840, -64.24504439390000243, -26.36014981959999659 ) ) ;
#17804=ORIENTED_EDGE ( 'NONE', *, *, #907, .T. ) ;
#17806=CARTESIAN_POINT ( 'NONE',  ( 28.43332587009999912, -71.30829807179999591, 2.547915100310000014 ) ) ;
#17809=CARTESIAN_POINT ( 'NONE',  ( -12.09181944520000052, -68.76958053619999589, -24.81138139369999962 ) ) ;
#17810=CARTESIAN_POINT ( 'NONE',  ( -11.22183525189999820, -57.45864775100000088, -21.12541653479999937 ) ) ;
#17824=CARTESIAN_POINT ( 'NONE',  ( -16.49390888960000368, -79.50000000000000000, 44.28897684009999836 ) ) ;
#17826=CARTESIAN_POINT ( 'NONE',  ( 8.983162410790001218, -36.08615800729999989, -20.65197200649999942 ) ) ;
#17827=AXIS2_PLACEMENT_3D ( 'NONE', #5710, #5150, #9652 ) ;
#17831=DIRECTION ( 'NONE',  ( 1.000000000000000000, 0.000000000000000000, 0.000000000000000000 ) ) ;
#17833=DIRECTION ( 'NONE',  ( 1.000000000000000000, 0.000000000000000000, 0.000000000000000000 ) ) ;
#17835=CARTESIAN_POINT ( 'NONE',  ( 28.81424833448794942, -71.66550124175094538, 2.966281764014999656 ) ) ;
#17839=B_SPLINE_SURFACE_WITH_KNOTS ( 'NONE', 5, 5, ( 
 ( #2666, #11820, #792, #2810, #14303, #24806, #11667, #9189, #7033 ),
 ( #4843, #3109, #9492, #16342, #18397, #25250, #20578, #25098, #9776 ),
 ( #11517, #20875, #11961, #14166, #27432, #16189, #5279, #3245, #25393 ),
 ( #21017, #9631, #4979, #22769, #934, #5419, #27140, #14013, #18689 ),
 ( #22919, #13866, #27585, #23198, #13722, #20734, #12101, #7180, #7626 ),
 ( #18092, #18537, #15899, #22622, #10320, #1619, #23891, #19374, #1078 ) ),
 .UNSPECIFIED., .F., .F., .F.,
 ( 6, 6 ),
 ( 6, 3, 6 ),
 ( 0.000000000000000000, 46.92994236210000025 ),
 ( 0.000000000000000000, 1.000000000000000000, 2.000000000000000000 ),
 .UNSPECIFIED. ) ;
#17841=DIRECTION ( 'NONE',  ( -0.3687499999999814260, 0.000000000000000000, 0.9295286103719527793 ) ) ;
#17843=CARTESIAN_POINT ( 'NONE',  ( -13.45981261770000081, -71.49302942239999936, -24.63802173330000045 ) ) ;
#17847=CARTESIAN_POINT ( 'NONE',  ( 36.59060417929999431, -75.00000019720000921, -14.75000047440000017 ) ) ;
#17849=CIRCLE ( 'NONE', #14134, 0.5000000000000004441 ) ;
#17851=CARTESIAN_POINT ( 'NONE',  ( -12.77829499169999927, -60.48561587360000402, 20.49208202570000026 ) ) ;
#17852=CARTESIAN_POINT ( 'NONE',  ( 7.239203719536035031, -74.26034152750678174, 40.39659210523164745 ) ) ;
#17857=CARTESIAN_POINT ( 'NONE',  ( -11.49099193064466817, -57.47122622516366874, -20.56185111776623486 ) ) ;
#17858=ORIENTED_EDGE ( 'NONE', *, *, #3812, .T. ) ;
#17861=CARTESIAN_POINT ( 'NONE',  ( 8.036479196959999201E-15, -84.50000000000000000, -43.75000000000000000 ) ) ;
#17862=CARTESIAN_POINT ( 'NONE',  ( 7.250123850439999629, -73.75838856979999036, -39.12175830369999829 ) ) ;
#17863=ORIENTED_EDGE ( 'NONE', *, *, #10792, .T. ) ;
#17867=CARTESIAN_POINT ( 'NONE',  ( -9.642319748410001168, -18.50000000000000000, -21.65408590870000083 ) ) ;
#17869=CARTESIAN_POINT ( 'NONE',  ( 7.105427357599999217E-15, -69.00000000000000000, 40.00000000000000000 ) ) ;
#17871=CARTESIAN_POINT ( 'NONE',  ( 19.41707937360000003, -18.50000000000000000, 9.264983660499998663 ) ) ;
#17874=EDGE_LOOP ( 'NONE', ( #19288, #3709, #9953 ) ) ;
#17875=DIRECTION ( 'NONE',  ( 0.1066420485059984824, 0.000000000000000000, 0.9942974773630094409 ) ) ;
#17876=CARTESIAN_POINT ( 'NONE',  ( 9.024081099289999131, -19.49999992740000110, -18.94592230980000380 ) ) ;
#17877=CARTESIAN_POINT ( 'NONE',  ( -16.78865735879999832, -74.00000000000000000, 25.46808810279999946 ) ) ;
#17879=CARTESIAN_POINT ( 'NONE',  ( 23.93312658989999875, -65.07443093669999712, -7.727579958389999781 ) ) ;
#17880=ORIENTED_EDGE ( 'NONE', *, *, #14157, .T. ) ;
#17882=CIRCLE ( 'NONE', #228, 0.4999999999999967804 ) ;
#17885=CARTESIAN_POINT ( 'NONE',  ( -7.325370793560000315, -18.50000000000000000, -24.94672208400000102 ) ) ;
#17886=CARTESIAN_POINT ( 'NONE',  ( 19.54920062769999944, -35.79804965070000122, -9.079275989799999280 ) ) ;
#17887=CONICAL_SURFACE ( 'NONE', #2556, 25.14975229270001833, 0.4276056667390000787 ) ;
#17888=CARTESIAN_POINT ( 'NONE',  ( -0.5884599110899999541, -61.88564085890000399, -23.95484640009999922 ) ) ;
#17889=EDGE_LOOP ( 'NONE', ( #12818, #22584, #26667 ) ) ;
#17891=TOROIDAL_SURFACE ( 'NONE', #21171, 0.5000000000000000000, 0.5000000000000000000 ) ;
#17892=ORIENTED_EDGE ( 'NONE', *, *, #2284, .F. ) ;
#17897=CARTESIAN_POINT ( 'NONE',  ( 21.88953683589687671, -18.85523522018264941, -0.4607246244462301910 ) ) ;
#17898=CARTESIAN_POINT ( 'NONE',  ( -22.00249007819999747, -79.50000010050000299, -32.67527197889999258 ) ) ;
#17899=EDGE_CURVE ( 'NONE', #6032, #3916, #12065, .T. ) ;
#17905=VERTEX_POINT ( 'NONE', #17116 ) ;
#17910=CARTESIAN_POINT ( 'NONE',  ( -40.03821526680000176, -73.97917265380000629, 7.260248548399999891 ) ) ;
#17911=CARTESIAN_POINT ( 'NONE',  ( -21.98999391060000264, -74.14434415679998835, -32.46673792200000008 ) ) ;
#17914=DIRECTION ( 'NONE',  ( 0.000000000000000000, 0.000000000000000000, -1.000000000000000000 ) ) ;
#17915=CARTESIAN_POINT ( 'NONE',  ( -18.46388027080000072, -18.85965710059999978, 13.47021038649999980 ) ) ;
#17918=AXIS2_PLACEMENT_3D ( 'NONE', #471, #7599, #7454 ) ;
#17919=CARTESIAN_POINT ( 'NONE',  ( 20.32381860445705968, -73.59933368480965044, -31.74152625608882161 ) ) ;
#17921=FACE_OUTER_BOUND ( 'NONE', #8661, .T. ) ;
#17928=CARTESIAN_POINT ( 'NONE',  ( 24.39713723570755022, -19.23820060856055392, 1.459765156892738558 ) ) ;
#17929=ORIENTED_EDGE ( 'NONE', *, *, #3188, .F. ) ;
#17930=CARTESIAN_POINT ( 'NONE',  ( -13.61274982059999950, -49.81668346450000229, 20.80692016579999759 ) ) ;
#17932=EDGE_LOOP ( 'NONE', ( #8669, #3156, #15387 ) ) ;
#17934=EDGE_CURVE ( 'NONE', #27321, #6167, #4175, .T. ) ;
#17937=CARTESIAN_POINT ( 'NONE',  ( -26.33972759919999973, -74.50000000000000000, -36.23922253580000330 ) ) ;
#17939=CARTESIAN_POINT ( 'NONE',  ( 26.57206548991637973, -68.20221397703001287, 0.6012562671682266657 ) ) ;
#17940=CARTESIAN_POINT ( 'NONE',  ( 26.22877582859999990, -72.82938648530000592, 11.61106434019999867 ) ) ;
#17941=ORIENTED_EDGE ( 'NONE', *, *, #1722, .T. ) ;
#17942=EDGE_CURVE ( 'NONE', #22026, #28497, #3012, .T. ) ;
#17943=DIRECTION ( 'NONE',  ( 0.000000000000000000, -1.000000000000000000, 0.000000000000000000 ) ) ;
#17949=CARTESIAN_POINT ( 'NONE',  ( 19.97576656849999921, -19.50000000000000000, -19.97576656849999921 ) ) ;
#17950=EDGE_LOOP ( 'NONE', ( #6580, #8936, #27983, #22278 ) ) ;
#17951=CARTESIAN_POINT ( 'NONE',  ( 27.79580722110000224, -70.93604331640000282, 1.283943149509999992 ) ) ;
#17953=CARTESIAN_POINT ( 'NONE',  ( 26.08183366116990243, -74.32916785640455259, -29.29060224673261459 ) ) ;
#17954=CARTESIAN_POINT ( 'NONE',  ( -12.22902516030000086, -69.69726588759999686, -24.77074270770000197 ) ) ;
#17955=CARTESIAN_POINT ( 'NONE',  ( 23.78781103989999934, -65.02207070560001512, -8.286109287880000451 ) ) ;
#17956=FACE_OUTER_BOUND ( 'NONE', #3173, .T. ) ;
#17958=DIRECTION ( 'NONE',  ( 0.7071067811865475727, 0.000000000000000000, 0.7071067811865475727 ) ) ;
#17960=CARTESIAN_POINT ( 'NONE',  ( -3.610293368829999849, -18.50000000000000000, -24.43613445369999937 ) ) ;
#17962=DIRECTION ( 'NONE',  ( 1.000000000000000000, 0.000000000000000000, 0.000000000000000000 ) ) ;
#17967=CARTESIAN_POINT ( 'NONE',  ( 22.76152370333024422, -19.47294761907691907, 1.041135354044837147 ) ) ;
#17969=CARTESIAN_POINT ( 'NONE',  ( 27.02346536675331734, -72.26149772935862359, -11.39735799491197987 ) ) ;
#17971=CARTESIAN_POINT ( 'NONE',  ( 9.289605485279999186, -35.98680449440000473, -20.22331461079999926 ) ) ;
#17972=ADVANCED_FACE ( 'NONE', ( #22361 ), #21596, .T. ) ;
#17973=DIRECTION ( 'NONE',  ( 1.000000000000000000, 0.000000000000000000, 0.000000000000000000 ) ) ;
#17974=EDGE_CURVE ( 'NONE', #23734, #27321, #392, .T. ) ;
#17976=CARTESIAN_POINT ( 'NONE',  ( 24.41973528469999977, -18.87168159810000034, 1.581049218290000002 ) ) ;
#17981=CARTESIAN_POINT ( 'NONE',  ( 28.22776569104305722, -69.76795196468695792, 2.414911384691903251 ) ) ;
#17983=CARTESIAN_POINT ( 'NONE',  ( 7.019998623859999398, -53.29680639659999741, -22.12830645909999916 ) ) ;
#17984=CARTESIAN_POINT ( 'NONE',  ( 20.82957722899999808, -36.00000000010000178, -9.510883249549999974 ) ) ;
#17985=DIRECTION ( 'NONE',  ( -0.9704142011833034598, 0.000000000000000000, -0.2414462220490750932 ) ) ;
#17986=LINE ( 'NONE', #17843, #1248 ) ;
#17987=LINE ( 'NONE', #13606, #9033 ) ;
#17988=CARTESIAN_POINT ( 'NONE',  ( 1.013794083399999955E-14, -69.50000000000000000, 33.25000000000000000 ) ) ;
#17989=ORIENTED_EDGE ( 'NONE', *, *, #26947, .T. ) ;
#17992=ORIENTED_EDGE ( 'NONE', *, *, #14658, .F. ) ;
#17994=CARTESIAN_POINT ( 'NONE',  ( -11.31498420849999853, -60.59635495490000778, 20.73642217629999962 ) ) ;
#17995=CARTESIAN_POINT ( 'NONE',  ( 7.244146985818051832, -74.18164516875302184, 40.29126735535029269 ) ) ;
#17997=CARTESIAN_POINT ( 'NONE',  ( 21.85900874260000037, -37.33604033319999616, -8.605626153620001162 ) ) ;
#17998=CARTESIAN_POINT ( 'NONE',  ( -12.06048066911961492, -66.52142429456056050, -24.43994840845913075 ) ) ;
#17999=EDGE_CURVE ( 'NONE', #23425, #6357, #20168, .T. ) ;
#18001=ORIENTED_EDGE ( 'NONE', *, *, #16717, .T. ) ;
#18002=DIRECTION ( 'NONE',  ( 1.738658080640003812E-17, 0.000000000000000000, -1.000000000000000000 ) ) ;
#18003=EDGE_CURVE ( 'NONE', #23692, #3267, #27114, .T. ) ;
#18006=CARTESIAN_POINT ( 'NONE',  ( -13.17060483900000101, -68.28989248250000799, -23.12790341000000183 ) ) ;
#18009=CARTESIAN_POINT ( 'NONE',  ( 19.74600256529999953, -32.73130089770000239, 10.78004968070000125 ) ) ;
#18010=CARTESIAN_POINT ( 'NONE',  ( -0.5856137342820000313, -19.46510053389999939, -22.02591827759999887 ) ) ;
#18012=CARTESIAN_POINT ( 'NONE',  ( 22.16736984139999933, -65.04750180880000698, 11.85329599529999989 ) ) ;
#18013=CARTESIAN_POINT ( 'NONE',  ( -32.76786048424294506, -79.86746516107372429, -22.38819307479873544 ) ) ;
#18015=B_SPLINE_SURFACE_WITH_KNOTS ( 'NONE', 5, 5, ( 
 ( #2710, #24850, #27184, #9095, #9239, #16090 ),
 ( #5027, #13915, #689, #11717, #9541, #18443 ),
 ( #27329, #2570, #11418, #7371, #27040, #7531 ),
 ( #25147, #3010, #16387, #20320, #17997, #18141 ),
 ( #15945, #4888, #6916, #237, #15783, #26877 ),
 ( #9082, #17984, #26504, #9146, #2036, #8700 ) ),
 .UNSPECIFIED., .F., .F., .F.,
 ( 6, 6 ),
 ( 6, 6 ),
 ( 3.491867373409999864, 4.007730545210000273 ),
 ( 0.000000000000000000, 2.000000000000000000 ),
 .UNSPECIFIED. ) ;
#18016=EDGE_LOOP ( 'NONE', ( #26902, #28306, #23485, #10870 ) ) ;
#18021=CARTESIAN_POINT ( 'NONE',  ( -40.03809227510000568, -73.97913911409999344, -7.260235792849999648 ) ) ;
#18022=EDGE_LOOP ( 'NONE', ( #5169, #8479, #15806, #18901 ) ) ;
#18025=ORIENTED_EDGE ( 'NONE', *, *, #4441, .F. ) ;
#18026=DIRECTION ( 'NONE',  ( 0.000000000000000000, 1.000000000000000000, 0.000000000000000000 ) ) ;
#18030=ORIENTED_EDGE ( 'NONE', *, *, #16021, .F. ) ;
#18032=CARTESIAN_POINT ( 'NONE',  ( -14.93121066289999987, -82.25000000000000000, 36.29905574720000061 ) ) ;
#18036=DIRECTION ( 'NONE',  ( 0.9982470477219616001, 0.000000000000000000, 0.05918472534689760839 ) ) ;
#18037=ORIENTED_EDGE ( 'NONE', *, *, #7604, .T. ) ;
#18039=CARTESIAN_POINT ( 'NONE',  ( 38.62788938250000115, -74.00000000000000000, 7.627566167509999495 ) ) ;
#18044=CARTESIAN_POINT ( 'NONE',  ( 7.460698725479999927E-15, -73.50000000000000000, 40.00000000000000000 ) ) ;
#18045=ORIENTED_EDGE ( 'NONE', *, *, #13073, .T. ) ;
#18047=CARTESIAN_POINT ( 'NONE',  ( -2.583988331150000040, -57.40875702419999982, -25.23271569440000306 ) ) ;
#18048=DIRECTION ( 'NONE',  ( 0.000000000000000000, 1.000000000000000000, 0.000000000000000000 ) ) ;
#18049=CARTESIAN_POINT ( 'NONE',  ( -22.02869148110000452, -74.01492597349999869, -32.14913059759999214 ) ) ;
#18050=CARTESIAN_POINT ( 'NONE',  ( 8.988996100299999625, -34.66800400750000222, -19.43643858049999906 ) ) ;
#18054=ORIENTED_EDGE ( 'NONE', *, *, #20660, .F. ) ;
#18055=DIRECTION ( 'NONE',  ( 0.000000000000000000, 1.000000000000000000, 0.000000000000000000 ) ) ;
#18057=CARTESIAN_POINT ( 'NONE',  ( -11.16118678780000018, -74.00000000000000000, 46.75000000000000000 ) ) ;
#18061=CARTESIAN_POINT ( 'NONE',  ( 47.25083273380000293, -79.30142995810000173, -0.9228940748419999229 ) ) ;
#18062=CARTESIAN_POINT ( 'NONE',  ( 13.45981261770000081, -71.49302942239999936, 24.63802173330000045 ) ) ;
#18064=PRODUCT_CONTEXT ( 'NONE', #11440, 'mechanical' ) ;
#18065=AXIS2_PLACEMENT_3D ( 'NONE', #4201, #4053, #12920 ) ;
#18066=CARTESIAN_POINT ( 'NONE',  ( 23.42789392040000251, -57.47571038070000782, 0.04069498556230000119 ) ) ;
#18067=ADVANCED_FACE ( 'NONE', ( #15933 ), #16223, .F. ) ;
#18070=CARTESIAN_POINT ( 'NONE',  ( 46.91398284789494966, -74.02346682147648949, -2.186286367158106980 ) ) ;
#18072=CARTESIAN_POINT ( 'NONE',  ( -14.15885437638525168, -18.49999999992862953, 20.15290185130359291 ) ) ;
#18074=ORIENTED_EDGE ( 'NONE', *, *, #22784, .T. ) ;
#18075=CARTESIAN_POINT ( 'NONE',  ( 9.476129726560001743, -36.00000000000000000, -20.06309461059999677 ) ) ;
#18077=CARTESIAN_POINT ( 'NONE',  ( 22.02882315030000271, -19.46510050329999686, -0.4636558402470000173 ) ) ;
#18080=CARTESIAN_POINT ( 'NONE',  ( 27.13958276158709282, -67.66819096094158681, 1.745391524347732704 ) ) ;
#18081=ORIENTED_EDGE ( 'NONE', *, *, #24232, .T. ) ;
#18084=CARTESIAN_POINT ( 'NONE',  ( -2.578307999469999778, -19.50000000000000000, -25.11373953509999879 ) ) ;
#18085=CARTESIAN_POINT ( 'NONE',  ( -32.32657687519999712, -74.05570514439999386, -21.80503578329999925 ) ) ;
#18087=CARTESIAN_POINT ( 'NONE',  ( 3.907985046679999924E-15, -73.50000000000000000, -40.00000000000000000 ) ) ;
#18089=CARTESIAN_POINT ( 'NONE',  ( -21.88268327719999817, -66.31484486759998731, 16.13005244970000263 ) ) ;
#18091=CARTESIAN_POINT ( 'NONE',  ( 37.29611236860000645, -80.00000000000000000, -13.75000000000000000 ) ) ;
#18092=CARTESIAN_POINT ( 'NONE',  ( -18.78215030510000005, -19.46363745430000236, 11.52009539260000004 ) ) ;
#18093=CARTESIAN_POINT ( 'NONE',  ( 24.27323469296766234, -74.17273658677886772, -30.68895570800956918 ) ) ;
#18099=CARTESIAN_POINT ( 'NONE',  ( 8.235816542629999560E-15, -69.50000000000000000, -40.00000000000000000 ) ) ;
#18100=VECTOR ( 'NONE', #16995, 1000.000000000000000 ) ;
#18102=EDGE_CURVE ( 'NONE', #15244, #26586, #17397, .T. ) ;
#18104=AXIS2_PLACEMENT_3D ( 'NONE', #23320, #21409, #5818 ) ;
#18105=AXIS2_PLACEMENT_3D ( 'NONE', #23704, #12468, #14939 ) ;
#18106=VERTEX_POINT ( 'NONE', #25138 ) ;
#18108=CARTESIAN_POINT ( 'NONE',  ( 10.29737924729999854, -36.00000000000000000, -20.64806254930000051 ) ) ;
#18109=DIRECTION ( 'NONE',  ( 0.000000000000000000, 1.000000000000000000, 0.000000000000000000 ) ) ;
#18113=EDGE_LOOP ( 'NONE', ( #3418, #8012, #19802, #1422 ) ) ;
#18114=CARTESIAN_POINT ( 'NONE',  ( 7.440556932049999794, -74.12472287219999600, 39.45553247920000217 ) ) ;
#18117=CARTESIAN_POINT ( 'NONE',  ( -3.730706907091303481, -79.99999997488282588, 46.61318877841384989 ) ) ;
#18118=CARTESIAN_POINT ( 'NONE',  ( 8.390131615779999663, -37.63096262599999875, -21.73500566539999923 ) ) ;
#18121=DIRECTION ( 'NONE',  ( 0.000000000000000000, -1.000000000000000000, 0.000000000000000000 ) ) ;
#18122=DIRECTION ( 'NONE',  ( 1.000000000000000000, 0.000000000000000000, 0.000000000000000000 ) ) ;
#18123=DIRECTION ( 'NONE',  ( -0.000000000000000000, 1.000000000000000000, 0.000000000000000000 ) ) ;
#18125=CARTESIAN_POINT ( 'NONE',  ( 27.76234330132245276, -68.29340503348747404, 2.076308288554540304 ) ) ;
#18127=AXIS2_PLACEMENT_3D ( 'NONE', #426, #7561, #27071 ) ;
#18130=DIRECTION ( 'NONE',  ( 0.000000000000000000, 1.000000000000000000, 0.000000000000000000 ) ) ;
#18131=CARTESIAN_POINT ( 'NONE',  ( 20.06309763089999620, -36.00000000000000000, -9.476129751679998492 ) ) ;
#18132=CARTESIAN_POINT ( 'NONE',  ( -10.60770804610000084, -19.15810967940000253, 19.29995473580000009 ) ) ;
#18133=ORIENTED_EDGE ( 'NONE', *, *, #4842, .T. ) ;
#18135=CARTESIAN_POINT ( 'NONE',  ( 36.29507663750000290, -74.81267993790000048, -14.94134320780000103 ) ) ;
#18136=EDGE_CURVE ( 'NONE', #1612, #18945, #9668, .T. ) ;
#18138=CARTESIAN_POINT ( 'NONE',  ( -41.00000000000000000, -74.00000000000000000, -10.20110288159999890 ) ) ;
#18139=CARTESIAN_POINT ( 'NONE',  ( 0.000000000000000000, -57.47855601759999900, 0.000000000000000000 ) ) ;
#18141=CARTESIAN_POINT ( 'NONE',  ( 21.87044453209999872, -37.95525411010000028, -8.597789012979999868 ) ) ;
#18142=AXIS2_PLACEMENT_3D ( 'NONE', #8442, #14991, #26238 ) ;
#18143=AXIS2_PLACEMENT_3D ( 'NONE', #8927, #26872, #22507 ) ;
#18144=DIRECTION ( 'NONE',  ( 0.000000000000000000, 0.000000000000000000, -1.000000000000000000 ) ) ;
#18145=ORIENTED_EDGE ( 'NONE', *, *, #27784, .F. ) ;
#18146=CARTESIAN_POINT ( 'NONE',  ( -7.215414233289999757, -74.50000000000000000, -40.70731707320000226 ) ) ;
#18147=DIRECTION ( 'NONE',  ( 0.000000000000000000, 1.000000000000000000, 0.000000000000000000 ) ) ;
#18149=EDGE_LOOP ( 'NONE', ( #8988, #5899, #15765, #10113 ) ) ;
#18150=CARTESIAN_POINT ( 'NONE',  ( -13.04239910971960015, -66.15241698556883421, -22.07654756397324292 ) ) ;
#18151=B_SPLINE_CURVE_WITH_KNOTS ( 'NONE', 3,
 ( #10562, #7859, #25777, #21259, #25493, #3900, #16741, #16887, #28366, #16600, #12482, #25635, #12763, #21674, #14546, #17157, #8258, #23452, #1724, #3353, #19351, #5932, #26046, #10155, #12217, #19074, #3489, #10295, #21395, #14953, #1452, #1185, #5666, #12349, #23860, #6073 ),
 .UNSPECIFIED., .F., .F.,
 ( 4, 2, 2, 1, 1, 1, 1, 2, 2, 2, 1, 1, 1, 1, 2, 2, 2, 1, 1, 1, 1, 2, 2, 4 ),
 ( 0.000000000000000000, 0.1250000000000244804, 0.1875000000000347777, 0.2187500000000399125, 0.2343750000000394962, 0.2421875000000392741, 0.2460937500000396905, 0.2480468750000404121, 0.2500000000000411338, 0.3750000000000714429, 0.4375000000000848766, 0.4687500000000905942, 0.4843750000000933142, 0.4921875000000928702, 0.4960937500000925926, 0.5000000000000922595, 0.6250000000000517364, 0.6875000000000291989, 0.7187500000000193179, 0.7343750000000142109, 0.7421875000000096589, 0.7460937500000072164, 0.7500000000000047740, 1.000000000000000000 ),
 .UNSPECIFIED. ) ;
#18155=B_SPLINE_CURVE_WITH_KNOTS ( 'NONE', 5,
 ( #2455, #10706, #28512, #132, #6362, #4626, #17593, #8678, #12899, #17886, #15227, #9127 ),
 .UNSPECIFIED., .F., .F.,
 ( 6, 3, 3, 6 ),
 ( 0.000000000000000000, 0.1767099789820964495, 0.4698587576253994702, 1.000000000000000000 ),
 .UNSPECIFIED. ) ;
#18157=CARTESIAN_POINT ( 'NONE',  ( -7.221517031004696108, -73.63371395845983614, -39.35783505872542776 ) ) ;
#18158=CARTESIAN_POINT ( 'NONE',  ( 19.61197036049999909, -18.61786835250000038, 9.515235106480000482 ) ) ;
#18159=CARTESIAN_POINT ( 'NONE',  ( -21.43328945980000100, -64.24504445130001784, 15.59674557630000180 ) ) ;
#18161=ORIENTED_EDGE ( 'NONE', *, *, #23439, .T. ) ;
#18162=CARTESIAN_POINT ( 'NONE',  ( -12.63785399150000011, -72.17920235959999786, -25.42231943180000187 ) ) ;
#18163=EDGE_CURVE ( 'NONE', #26221, #9130, #9450, .T. ) ;
#18165=CARTESIAN_POINT ( 'NONE',  ( 22.35420107259999867, -19.50000000000000000, 9.881343484100000296 ) ) ;
#18166=AXIS2_PLACEMENT_3D ( 'NONE', #2184, #11, #8858 ) ;
#18170=EDGE_CURVE ( 'NONE', #12644, #1175, #26657, .T. ) ;
#18172=ORIENTED_EDGE ( 'NONE', *, *, #14844, .T. ) ;
#18173=DIRECTION ( 'NONE',  ( 0.000000000000000000, 1.000000000000000000, 0.000000000000000000 ) ) ;
#18177=EDGE_LOOP ( 'NONE', ( #24464, #25934, #24244, #22164 ) ) ;
#18179=ORIENTED_EDGE ( 'NONE', *, *, #21386, .F. ) ;
#18180=CARTESIAN_POINT ( 'NONE',  ( -22.84072196045827496, -70.62850378349290281, 15.63790239815233996 ) ) ;
#18181=FACE_OUTER_BOUND ( 'NONE', #16810, .T. ) ;
#18182=CARTESIAN_POINT ( 'NONE',  ( 47.08865343609999599, -74.38949312799999802, -1.581891583850000060 ) ) ;
#18183=EDGE_LOOP ( 'NONE', ( #9354, #27346, #5772, #23296 ) ) ;
#18184=AXIS2_PLACEMENT_3D ( 'NONE', #2725, #27200, #15961 ) ;
#18186=CARTESIAN_POINT ( 'NONE',  ( -11.77059236524900676, -63.22433976061354599, 21.39084228963605483 ) ) ;
#18187=AXIS2_PLACEMENT_3D ( 'NONE', #4067, #21705, #1756 ) ;
#18189=ADVANCED_FACE ( 'NONE', ( #20769 ), #8068, .F. ) ;
#18190=CARTESIAN_POINT ( 'NONE',  ( 30.45033996220000105, -72.00000000000000000, 1.805359716810000181 ) ) ;
#18194=CARTESIAN_POINT ( 'NONE',  ( 36.80494456599999609, -74.39262779950000493, -14.59792775669999898 ) ) ;
#18195=CARTESIAN_POINT ( 'NONE',  ( -2.790536503729999840, -64.24504439390000243, -26.36014981959999659 ) ) ;
#18196=CARTESIAN_POINT ( 'NONE',  ( -40.70731707320000226, -74.50000000000000000, 7.215414233289999757 ) ) ;
#18197=CARTESIAN_POINT ( 'NONE',  ( -21.98017993790000091, -74.00000000020000357, -32.02104148659999794 ) ) ;
#18201=CARTESIAN_POINT ( 'NONE',  ( -18.19560383140000326, -18.61776472269999871, 11.73914725620000077 ) ) ;
#18202=ORIENTED_EDGE ( 'NONE', *, *, #23094, .T. ) ;
#18204=ADVANCED_FACE ( 'NONE', ( #7518 ), #21322, .T. ) ;
#18208=CARTESIAN_POINT ( 'NONE',  ( 45.84677419350000349, -73.50000000000000000, -4.286925650119999709 ) ) ;
#18209=ORIENTED_EDGE ( 'NONE', *, *, #4159, .F. ) ;
#18210=CARTESIAN_POINT ( 'NONE',  ( 47.25120369400000442, -79.35618804639999269, -0.8986897406489999796 ) ) ;
#18211=AXIS2_PLACEMENT_3D ( 'NONE', #18992, #18861, #16522 ) ;
#18212=LINE ( 'NONE', #464, #11707 ) ;
#18213=CIRCLE ( 'NONE', #26125, 3.750000000000000000 ) ;
#18214=AXIS2_PLACEMENT_3D ( 'NONE', #20156, #226, #18122 ) ;
#18215=CARTESIAN_POINT ( 'NONE',  ( -11.76511348380000044, -63.41220263479998920, -21.95613077419999826 ) ) ;
#18216=FACE_OUTER_BOUND ( 'NONE', #27332, .T. ) ;
#18219=CARTESIAN_POINT ( 'NONE',  ( -12.00297273912186391, -70.31047685921210189, -25.86267369459898191 ) ) ;
#18221=CARTESIAN_POINT ( 'NONE',  ( -11.04737574249999987, -49.87551312379999757, 20.28213158860000220 ) ) ;
#18222=CARTESIAN_POINT ( 'NONE',  ( 7.105427357599999217E-15, -69.00000000000000000, -33.25000000000000000 ) ) ;
#18223=ORIENTED_EDGE ( 'NONE', *, *, #331, .T. ) ;
#18224=CARTESIAN_POINT ( 'NONE',  ( -9.356041104380000917, -74.00000000000000000, 37.60355029590000697 ) ) ;
#18225=EDGE_CURVE ( 'NONE', #27146, #18344, #5731, .T. ) ;
#18236=ORIENTED_EDGE ( 'NONE', *, *, #899, .F. ) ;
#18237=B_SPLINE_CURVE_WITH_KNOTS ( 'NONE', 3,
 ( #17637, #15423, #24334, #11493, #18072, #2645 ),
 .UNSPECIFIED., .F., .F.,
 ( 4, 2, 4 ),
 ( 0.000000000000000000, 0.5000000000000000000, 1.000000000000000000 ),
 .UNSPECIFIED. ) ;
#18241=FACE_OUTER_BOUND ( 'NONE', #22516, .T. ) ;
#18247=CARTESIAN_POINT ( 'NONE',  ( -14.72614960323499922, -74.20703269541404268, 36.28169309294055012 ) ) ;
#18249=CARTESIAN_POINT ( 'NONE',  ( 26.68454220230000118, -66.39602363720000255, 1.565571359830000064 ) ) ;
#18253=CARTESIAN_POINT ( 'NONE',  ( -39.22862632829222918, -73.58711170889174014, -7.208933142661926752 ) ) ;
#18257=CARTESIAN_POINT ( 'NONE',  ( 7.248115120159999591, -74.24284936579999794, 40.37845838710000379 ) ) ;
#18258=CARTESIAN_POINT ( 'NONE',  ( 47.09727354990000237, -74.46036430799999550, -1.896414880740000086 ) ) ;
#18260=B_SPLINE_SURFACE_WITH_KNOTS ( 'NONE', 5, 5, ( 
 ( #21212, #28602, #18524, #4886, #14022, #5428, #7901, #22932, #949 ),
 ( #27444, #14313, #18696, #18972, #27595, #5141, #2971, #9641, #16779 ),
 ( #25675, #16636, #3390, #7489, #14586, #5292, #23487, #3118, #9502 ),
 ( #25530, #18548, #27295, #1088, #7635, #9788, #16198, #21164, #20887 ),
 ( #16502, #3527, #14453, #25111, #10060, #14178, #23073, #23208, #3258 ),
 ( #12111, #21029, #20590, #9926, #23345, #19384, #24036, #10600, #24189 ),
 ( #26237, #3938, #19246, #5839, #17198, #28552, #14722, #21574, #1630 ),
 ( #28404, #12943, #28135, #26374, #12802, #28262, #17490, #17344, #21856 ),
 ( #12522, #10749, #14990, #19519, #23759, #8295, #15127, #12662, #1907 ),
 ( #10468, #23902, #6263, #3659, #4075, #10331, #10195, #23617, #19661 ),
 ( #21434, #8587, #8441, #15269, #25816, #14856, #26087, #25947, #12384 ),
 ( #21712, #21296, #5970, #1347, #6115, #19111, #1761, #17055, #1493 ) ),
 .UNSPECIFIED., .F., .F., .F.,
 ( 6, 3, 3, 6 ),
 ( 6, 3, 6 ),
 ( 3.065779847589999996, 3.494148935390000155, 4.204781552860000104, 5.489916222159999748 ),
 ( 0.000000000000000000, 1.000000000000000000, 2.000000000000000000 ),
 .UNSPECIFIED. ) ;
#18261=CARTESIAN_POINT ( 'NONE',  ( 22.17252228646381340, -19.46530601809573824, 0.2404182486420052278 ) ) ;
#18264=CARTESIAN_POINT ( 'NONE',  ( -20.69822367649999961, -60.21448500349999478, 14.94573686989999928 ) ) ;
#18265=CARTESIAN_POINT ( 'NONE',  ( 8.509936819460000024, -37.33446438219999663, -21.72762629869999884 ) ) ;
#18266=CARTESIAN_POINT ( 'NONE',  ( 8.613618054504685873, -19.47920864798205187, -19.98378909640561929 ) ) ;
#18268=ADVANCED_FACE ( 'NONE', ( #3969 ), #1518, .T. ) ;
#18270=AXIS2_PLACEMENT_3D ( 'NONE', #17497, #7943, #12298 ) ;
#18273=CARTESIAN_POINT ( 'NONE',  ( -2.557268395391378846, -19.48549492419126494, -23.46282872328029612 ) ) ;
#18280=LINE ( 'NONE', #27169, #10436 ) ;
#18281=CARTESIAN_POINT ( 'NONE',  ( -16.67828388959999941, -79.50000000000000000, 44.75374114529999758 ) ) ;
#18282=CARTESIAN_POINT ( 'NONE',  ( -21.43329341219999762, -64.24504445130001784, 15.59675287610000005 ) ) ;
#18284=CARTESIAN_POINT ( 'NONE',  ( 18.94592261899999741, -19.50000000000000000, -9.024080787800000891 ) ) ;
#18286=CARTESIAN_POINT ( 'NONE',  ( 36.60104255959999620, -74.78622670140001105, -14.73083308719999884 ) ) ;
#18288=CARTESIAN_POINT ( 'NONE',  ( -22.27690828497248887, -79.71584375156908209, -32.81592425880721464 ) ) ;
#18290=CARTESIAN_POINT ( 'NONE',  ( -15.08135542309999977, -67.66819112809999126, 22.63088101159999610 ) ) ;
#18291=CARTESIAN_POINT ( 'NONE',  ( 21.26630101029999764, -34.86445789710000298, -7.573067088439999317 ) ) ;
#18292=FACE_OUTER_BOUND ( 'NONE', #18977, .T. ) ;
#18295=CARTESIAN_POINT ( 'NONE',  ( 26.22877582859999990, -72.82938648530000592, 11.61106434019999867 ) ) ;
#18300=VERTEX_POINT ( 'NONE', #10362 ) ;
#18301=CARTESIAN_POINT ( 'NONE',  ( 29.56751773550223916, -74.29781185500684160, -25.75375116768845629 ) ) ;
#18303=ORIENTED_EDGE ( 'NONE', *, *, #21108, .T. ) ;
#18305=ADVANCED_FACE ( 'NONE', ( #3417 ), #11240, .T. ) ;
#18306=CARTESIAN_POINT ( 'NONE',  ( 20.49588873659998356, -52.63280639819947737, 10.85734681379999067 ) ) ;
#18309=AXIS2_PLACEMENT_3D ( 'NONE', #22978, #13632, #25161 ) ;
#18310=CARTESIAN_POINT ( 'NONE',  ( 36.32450514027038935, -74.54297173968070922, -14.86961495641581266 ) ) ;
#18314=CARTESIAN_POINT ( 'NONE',  ( -21.88268327719999817, -66.31484486759998731, 16.13005244970000263 ) ) ;
#18316=ORIENTED_EDGE ( 'NONE', *, *, #10785, .F. ) ;
#18317=CARTESIAN_POINT ( 'NONE',  ( -13.03622110660000111, -71.76391764010000429, -25.00534121280000122 ) ) ;
#18321=CARTESIAN_POINT ( 'NONE',  ( 21.58303657365043904, -19.48524588020601556, 9.513186693407064354 ) ) ;
#18322=CARTESIAN_POINT ( 'NONE',  ( -39.49501612540000650, -74.05258142259999943, -7.367357169149999940 ) ) ;
#18323=ORIENTED_EDGE ( 'NONE', *, *, #8631, .F. ) ;
#18325=ORIENTED_EDGE ( 'NONE', *, *, #18810, .T. ) ;
#18326=DIRECTION ( 'NONE',  ( 1.000000000000000000, 0.000000000000000000, 0.000000000000000000 ) ) ;
#18327=CIRCLE ( 'NONE', #11803, 1.000000000000000888 ) ;
#18328=CARTESIAN_POINT ( 'NONE',  ( 9.915197167549999691, -36.54217832150000334, -22.83075791629999785 ) ) ;
#18329=CARTESIAN_POINT ( 'NONE',  ( 21.92880676370000259, -37.95796630400000282, -8.677144394200000832 ) ) ;
#18334=CARTESIAN_POINT ( 'NONE',  ( 47.16974587269999830, -74.50000000000000000, -1.075755842369999993 ) ) ;
#18337=CARTESIAN_POINT ( 'NONE',  ( 7.247654292434177137, -73.86170940525964568, -39.81550290722874763 ) ) ;
#18339=ADVANCED_FACE ( 'NONE', ( #28582 ), #22937, .F. ) ;
#18341=DIRECTION ( 'NONE',  ( 0.9659258262889440783, 0.000000000000000000, -0.2588190451029840911 ) ) ;
#18342=CARTESIAN_POINT ( 'NONE',  ( -2.266663600180000238, -67.98014023149998764, -26.53490553780000027 ) ) ;
#18343=CARTESIAN_POINT ( 'NONE',  ( -14.57294834049999821, -70.03174454519999870, 23.21865845770000192 ) ) ;
#18344=VERTEX_POINT ( 'NONE', #22772 ) ;
#18346=CARTESIAN_POINT ( 'NONE',  ( 0.000000000000000000, -82.25000000000000000, -40.00000000000000000 ) ) ;
#18347=TOROIDAL_SURFACE ( 'NONE', #5767, 21.03431122519999974, 1.000000000000000000 ) ;
#18349=FACE_OUTER_BOUND ( 'NONE', #16500, .T. ) ;
#18350=CARTESIAN_POINT ( 'NONE',  ( -21.99985828019999801, -74.00000000000000000, -31.89935321680000158 ) ) ;
#18351=ORIENTED_EDGE ( 'NONE', *, *, #26829, .F. ) ;
#18353=CARTESIAN_POINT ( 'NONE',  ( 7.105427357599999217E-15, -69.00000000000000000, -46.75000000000000000 ) ) ;
#18355=ORIENTED_EDGE ( 'NONE', *, *, #9744, .F. ) ;
#18358=CARTESIAN_POINT ( 'NONE',  ( 8.986868621639999333, -35.35042264319999816, -19.48148203319999894 ) ) ;
#18360=CARTESIAN_POINT ( 'NONE',  ( 0.000000000000000000, -82.25000000000000000, -40.00000000000000000 ) ) ;
#18362=CARTESIAN_POINT ( 'NONE',  ( 46.55694345450000071, -80.05246764049999797, -3.671297399519999782 ) ) ;
#18363=CIRCLE ( 'NONE', #11814, 7.249999999999999112 ) ;
#18365=CARTESIAN_POINT ( 'NONE',  ( -11.47349711059999855, -61.75794029829999943, -22.43277763900000110 ) ) ;
#18368=CARTESIAN_POINT ( 'NONE',  ( 25.58501779599999892, -69.55030827429999363, -9.797057152780000777 ) ) ;
#18370=ORIENTED_EDGE ( 'NONE', *, *, #25325, .F. ) ;
#18372=ORIENTED_EDGE ( 'NONE', *, *, #9895, .T. ) ;
#18374=CARTESIAN_POINT ( 'NONE',  ( 20.94731949980000252, -52.62618816519999854, 10.41165191600000028 ) ) ;
#18377=PLANE ( 'NONE',  #12654 ) ;
#18380=CARTESIAN_POINT ( 'NONE',  ( -10.90069029708386061, -19.46519145482681523, -19.29382020368896278 ) ) ;
#18381=DIRECTION ( 'NONE',  ( 1.000000000000000000, 0.000000000000000000, 0.000000000000000000 ) ) ;
#18383=CARTESIAN_POINT ( 'NONE',  ( -10.47316257489999991, -19.17416318749999959, -21.16246808460000040 ) ) ;
#18384=CARTESIAN_POINT ( 'NONE',  ( 47.22403540388852150, -79.22821869427725971, -0.7816738164049302773 ) ) ;
#18386=FACE_OUTER_BOUND ( 'NONE', #5332, .T. ) ;
#18388=CARTESIAN_POINT ( 'NONE',  ( 10.20110288159999890, -84.00000000000000000, -41.00000000000000000 ) ) ;
#18392=CARTESIAN_POINT ( 'NONE',  ( 7.649154837969999399, -64.64960695860000328, -23.76019412080000137 ) ) ;
#18395=B_SPLINE_CURVE_WITH_KNOTS ( 'NONE', 3,
 ( #12399, #25834, #5856, #8459 ),
 .UNSPECIFIED., .F., .F.,
 ( 4, 4 ),
 ( 0.000000000000000000, 1.000000000000000000 ),
 .UNSPECIFIED. ) ;
#18396=AXIS2_PLACEMENT_3D ( 'NONE', #10357, #14742, #10220 ) ;
#18397=CARTESIAN_POINT ( 'NONE',  ( -19.32502251940000448, -45.98073373379999396, 13.48194705230000068 ) ) ;
#18404=CARTESIAN_POINT ( 'NONE',  ( 10.41045773099999927, -35.99999999980000354, -21.22141853569999981 ) ) ;
#18405=CARTESIAN_POINT ( 'NONE',  ( -19.47573906445313696, -18.50000000000000000, 15.05374977158872163 ) ) ;
#18410=CARTESIAN_POINT ( 'NONE',  ( 8.020103622739998883, -18.50000000000000000, -18.94130590319999996 ) ) ;
#18411=DIRECTION ( 'NONE',  ( 0.000000000000000000, 1.000000000000000000, 0.000000000000000000 ) ) ;
#18414=CARTESIAN_POINT ( 'NONE',  ( 9.212446728010000641, -35.92148816550000134, -19.60212694180000170 ) ) ;
#18415=CARTESIAN_POINT ( 'NONE',  ( 7.734359568749999525, -19.46510050329999686, -20.63161913629999944 ) ) ;
#18417=CARTESIAN_POINT ( 'NONE',  ( -40.01432744643470585, -73.98707088488757222, 7.250083186823315984 ) ) ;
#18418=CARTESIAN_POINT ( 'NONE',  ( 24.52276133189999996, -18.50000000000000000, 2.134003991790000221 ) ) ;
#18420=EDGE_LOOP ( 'NONE', ( #9429, #16998, #18431, #6113 ) ) ;
#18421=CARTESIAN_POINT ( 'NONE',  ( 1.776356839399999804E-15, -82.50000000000000000, 2.375877272699999867E-15 ) ) ;
#18423=CARTESIAN_POINT ( 'NONE',  ( -2.578307999469999778, -52.56313962710000709, -25.11373953509999879 ) ) ;
#18426=CIRCLE ( 'NONE', #9570, 0.5000000000000004441 ) ;
#18428=CARTESIAN_POINT ( 'NONE',  ( 22.02398067749999910, -53.29009989779999756, -7.952618468089998949 ) ) ;
#18429=CARTESIAN_POINT ( 'NONE',  ( -41.00000000000000000, -84.00000000000000000, 10.20110288159999890 ) ) ;
#18431=ORIENTED_EDGE ( 'NONE', *, *, #22382, .F. ) ;
#18432=EDGE_CURVE ( 'NONE', #26232, #16270, #2447, .T. ) ;
#18436=AXIS2_PLACEMENT_3D ( 'NONE', #3307, #25595, #22985 ) ;
#18439=CARTESIAN_POINT ( 'NONE',  ( 19.94240929510000271, -34.98557214560000261, -8.964904971799999345 ) ) ;
#18440=CARTESIAN_POINT ( 'NONE',  ( 7.248366623731350877, -73.88016183364510425, 39.84605369636854988 ) ) ;
#18441=EDGE_CURVE ( 'NONE', #12661, #22026, #25293, .T. ) ;
#18442=DIRECTION ( 'NONE',  ( 0.000000000000000000, -1.000000000000000000, 0.000000000000000000 ) ) ;
#18443=CARTESIAN_POINT ( 'NONE',  ( 21.81705090039999817, -37.95267571900000547, -8.514971793249999976 ) ) ;
#18449=CARTESIAN_POINT ( 'NONE',  ( -32.56304129029999217, -80.37807044109999310, -21.91706417159999987 ) ) ;
#18450=CARTESIAN_POINT ( 'NONE',  ( 0.000000000000000000, -65.07443093669999712, 0.000000000000000000 ) ) ;
#18456=DIRECTION ( 'NONE',  ( 0.3687499999999825917, 0.000000000000000000, -0.9295286103719523352 ) ) ;
#18457=CARTESIAN_POINT ( 'NONE',  ( -7.249313954213982392, -73.91187068844764951, -39.89765284858961536 ) ) ;
#18458=CARTESIAN_POINT ( 'NONE',  ( -14.59919359709999931, -74.45413981500000489, 36.80099833719999936 ) ) ;
#18462=CARTESIAN_POINT ( 'NONE',  ( -12.20941802519999975, -70.78179667580000967, -25.27574197309999704 ) ) ;
#18463=CARTESIAN_POINT ( 'NONE',  ( 8.805378577759999104, -28.56548875780000074, -20.15266227960000123 ) ) ;
#18464=DIRECTION ( 'NONE',  ( 1.000000000000000000, 0.000000000000000000, 0.000000000000000000 ) ) ;
#18465=CARTESIAN_POINT ( 'NONE',  ( 19.69821314702292625, -19.46453794985196595, 10.02888976161207957 ) ) ;
#18467=ORIENTED_EDGE ( 'NONE', *, *, #1032, .T. ) ;
#18469=EDGE_CURVE ( 'NONE', #10333, #3863, #6235, .T. ) ;
#18473=CARTESIAN_POINT ( 'NONE',  ( -36.23922253580000330, -80.00000000000000000, -27.04683438039999999 ) ) ;
#18476=ORIENTED_EDGE ( 'NONE', *, *, #20906, .T. ) ;
#18480=CARTESIAN_POINT ( 'NONE',  ( 47.09802472229999637, -74.43779277660000560, -1.603613559539999844 ) ) ;
#18482=CARTESIAN_POINT ( 'NONE',  ( 7.248706349655917869, -74.07739338312913446, -40.14660266898284391 ) ) ;
#18483=CARTESIAN_POINT ( 'NONE',  ( -11.72351936051625465, -62.99289890070036790, 21.32833123790344487 ) ) ;
#18484=CARTESIAN_POINT ( 'NONE',  ( -7.325370793560000315, -74.00000000000000000, -24.94672208400000102 ) ) ;
#18485=CARTESIAN_POINT ( 'NONE',  ( -3.546124265460000036, -70.16663891509999473, -27.89480033579999940 ) ) ;
#18486=CARTESIAN_POINT ( 'NONE',  ( -15.33695941859999934, -70.78240035880001813, 23.26337115899999830 ) ) ;
#18487=EDGE_LOOP ( 'NONE', ( #18576, #10602, #10013, #11640 ) ) ;
#18488=CARTESIAN_POINT ( 'NONE',  ( 36.40080311519999867, -74.58594348169998511, -14.77956081080000139 ) ) ;
#18491=VERTEX_POINT ( 'NONE', #21425 ) ;
#18493=PLANE ( 'NONE',  #26711 ) ;
#18496=CARTESIAN_POINT ( 'NONE',  ( -10.20110288159999890, -84.00000000000000000, 41.00000000000000000 ) ) ;
#18497=CARTESIAN_POINT ( 'NONE',  ( 22.32971180670000066, -62.77692288629999240, 10.61393702059999988 ) ) ;
#18498=DIRECTION ( 'NONE',  ( 0.000000000000000000, 1.000000000000000000, 0.000000000000000000 ) ) ;
#18500=FACE_OUTER_BOUND ( 'NONE', #10031, .T. ) ;
#18502=CARTESIAN_POINT ( 'NONE',  ( 46.85827871259999711, -80.18254846009999426, -2.615703315070000201 ) ) ;
#18503=EDGE_CURVE ( 'NONE', #19001, #10144, #10052, .T. ) ;
#18506=CARTESIAN_POINT ( 'NONE',  ( -11.33865485209999946, -58.84796781909999908, -22.38742378179999903 ) ) ;
#18507=CARTESIAN_POINT ( 'NONE',  ( 24.31832408829999892, -64.48635707210000589, -9.855635234570000236 ) ) ;
#18509=EDGE_CURVE ( 'NONE', #7537, #3863, #1758, .T. ) ;
#18512=CARTESIAN_POINT ( 'NONE',  ( 46.95741704872503419, -74.08013721110678773, -2.044574777238248764 ) ) ;
#18514=CARTESIAN_POINT ( 'NONE',  ( 22.48679802749999723, -53.79621871020000157, 10.10357420090000069 ) ) ;
#18518=DIRECTION ( 'NONE',  ( -0.7071067811865474617, 0.000000000000000000, 0.7071067811865474617 ) ) ;
#18522=FACE_OUTER_BOUND ( 'NONE', #10961, .T. ) ;
#18523=CARTESIAN_POINT ( 'NONE',  ( -10.41327899729999906, -18.50000000000000000, -22.30433628020000114 ) ) ;
#18524=CARTESIAN_POINT ( 'NONE',  ( 20.59810750560000159, -36.05978015090000355, -9.165578419380000952 ) ) ;
#18525=CARTESIAN_POINT ( 'NONE',  ( 46.72518785275575937, -79.87994607672447955, -3.403393787862253550 ) ) ;
#18528=DIRECTION ( 'NONE',  ( 0.000000000000000000, 1.000000000000000000, 0.000000000000000000 ) ) ;
#18531=B_SPLINE_CURVE_WITH_KNOTS ( 'NONE', 3,
 ( #3880, #14667, #19461, #21658, #1706, #23561, #6206, #15074 ),
 .UNSPECIFIED., .F., .F.,
 ( 4, 2, 2, 4 ),
 ( 0.000000000000000000, 0.2500000000000012212, 0.5000000000000024425, 1.000000000000000000 ),
 .UNSPECIFIED. ) ;
#18535=EDGE_LOOP ( 'NONE', ( #3770, #6306, #21625, #18635 ) ) ;
#18537=CARTESIAN_POINT ( 'NONE',  ( -18.60084818170000176, -19.46563609400000061, 11.81582046800000008 ) ) ;
#18538=CARTESIAN_POINT ( 'NONE',  ( 7.289196689104602278, -35.72560966896035239, -21.42683523805979462 ) ) ;
#18539=CARTESIAN_POINT ( 'NONE',  ( 27.75394116159999669, -74.50000000000000000, -27.75394116159999669 ) ) ;
#18543=TOROIDAL_SURFACE ( 'NONE', #3634, 6.750000000000000000, 0.5000000000000000000 ) ;
#18544=EDGE_CURVE ( 'NONE', #6780, #4268, #6666, .T. ) ;
#18545=ORIENTED_EDGE ( 'NONE', *, *, #8922, .T. ) ;
#18546=CARTESIAN_POINT ( 'NONE',  ( -39.29494613580084916, -73.61009970501154953, -7.215638845197088536 ) ) ;
#18548=CARTESIAN_POINT ( 'NONE',  ( 20.15734887640000039, -35.97442374919999963, -9.269656953000000144 ) ) ;
#18550=ORIENTED_EDGE ( 'NONE', *, *, #23576, .F. ) ;
#18551=DIRECTION ( 'NONE',  ( 0.000000000000000000, 1.000000000000000000, 0.000000000000000000 ) ) ;
#18552=CARTESIAN_POINT ( 'NONE',  ( -11.21645807309999832, -18.61794787939999907, -18.51636674970000129 ) ) ;
#18555=CARTESIAN_POINT ( 'NONE',  ( 46.43423234700000535, -80.49808279690000745, -3.486565683130000259 ) ) ;
#18558=CARTESIAN_POINT ( 'NONE',  ( 8.940781202869999333, -36.53304298860000188, -22.07739135909999817 ) ) ;
#18559=DIRECTION ( 'NONE',  ( 0.000000000000000000, 1.000000000000000000, 0.000000000000000000 ) ) ;
#18562=B_SPLINE_CURVE_WITH_KNOTS ( 'NONE', 3,
 ( #1748, #28392, #8575, #160, #9013, #26811 ),
 .UNSPECIFIED., .F., .F.,
 ( 4, 2, 4 ),
 ( 0.000000000000000000, 0.5000000000000000000, 1.000000000000000000 ),
 .UNSPECIFIED. ) ;
#18564=CARTESIAN_POINT ( 'NONE',  ( 23.97060671510000063, -18.50000000000000000, 2.556446744250000069 ) ) ;
#18567=CARTESIAN_POINT ( 'NONE',  ( -1.741759767157955219, -19.46809228179713713, -22.35565690618285828 ) ) ;
#18570=CARTESIAN_POINT ( 'NONE',  ( -1.993723132860000025, -52.61368720120000120, -23.68602550419999986 ) ) ;
#18572=DIRECTION ( 'NONE',  ( 0.9993816408608721114, 0.000000000000000000, -0.03516156865429537204 ) ) ;
#18573=CARTESIAN_POINT ( 'NONE',  ( 20.85226889350772339, -36.17942473021693672, -9.018047964458704158 ) ) ;
#18574=CARTESIAN_POINT ( 'NONE',  ( 21.61346702620000215, -40.75181153009999946, -7.194012074159999770 ) ) ;
#18575=CARTESIAN_POINT ( 'NONE',  ( -40.70731707320000226, -74.50000000000000000, -7.215414233289999757 ) ) ;
#18576=ORIENTED_EDGE ( 'NONE', *, *, #18731, .T. ) ;
#18578=ADVANCED_FACE ( 'NONE', ( #22146 ), #15414, .T. ) ;
#18580=AXIS2_PLACEMENT_3D ( 'NONE', #18819, #21271, #11949 ) ;
#18581=CARTESIAN_POINT ( 'NONE',  ( -32.77174708420000115, -74.50000000069999828, -21.60034937769999885 ) ) ;
#18583=AXIS2_PLACEMENT_3D ( 'NONE', #26977, #9172, #8875 ) ;
#18584=CARTESIAN_POINT ( 'NONE',  ( -13.91383203010000003, -65.33610288280000589, 21.79517489670000074 ) ) ;
#18585=CARTESIAN_POINT ( 'NONE',  ( 20.45837631639999898, -35.09297533480000908, -8.783856190409998987 ) ) ;
#18587=B_SPLINE_CURVE_WITH_KNOTS ( 'NONE', 5,
 ( #14948, #25771, #27812, #10290, #21256, #12346 ),
 .UNSPECIFIED., .F., .F.,
 ( 6, 6 ),
 ( 0.000000000000000000, 1.000000000000000000 ),
 .UNSPECIFIED. ) ;
#18588=DIRECTION ( 'NONE',  ( -0.1770468907230370870, 0.000000000000000000, -0.9842024174352068666 ) ) ;
#18590=B_SPLINE_CURVE_WITH_KNOTS ( 'NONE', 3,
 ( #17879, #13644, #19756, #26779, #22400, #123, #11442, #9267, #26472, #24874, #6959, #2147, #15672, #278, #8820, #10846, #13196, #26620, #13337, #2445, #11301, #20348, #15971, #19901, #4909, #21958, #8672, #2007 ),
 .UNSPECIFIED., .F., .F.,
 ( 4, 2, 1, 1, 1, 1, 2, 2, 2, 2, 1, 1, 1, 1, 2, 2, 2, 4 ),
 ( 0.000000000000000000, 0.1250000000000460465, 0.1875000000000690559, 0.2187500000000805744, 0.2343750000000861811, 0.2421875000000865696, 0.2460937500000842382, 0.2500000000000818789, 0.3750000000000255351, 0.4374999999999959477, 0.4687499999999797939, 0.4843749999999705791, 0.4921874999999659717, 0.4960937499999635292, 0.4980468749999634737, 0.4999999999999634182, 0.7499999999999816813, 1.000000000000000000 ),
 .UNSPECIFIED. ) ;
#18593=ORIENTED_EDGE ( 'NONE', *, *, #22206, .F. ) ;
#18594=VECTOR ( 'NONE', #22260, 1000.000000000000000 ) ;
#18595=FILL_AREA_STYLE_COLOUR ( '', #24545 ) ;
#18601=AXIS2_PLACEMENT_3D ( 'NONE', #9141, #2031, #10871 ) ;
#18604=ADVANCED_FACE ( 'NONE', ( #26365 ), #8578, .T. ) ;
#18605=CARTESIAN_POINT ( 'NONE',  ( -7.227599506459999823, -73.59185047150000969, 39.32706724020000877 ) ) ;
#18606=CARTESIAN_POINT ( 'NONE',  ( -10.04487041370000000, -18.50000000000000000, -22.35700885240000346 ) ) ;
#18608=CARTESIAN_POINT ( 'NONE',  ( -21.83717417439999764, -67.94514003989999651, 15.21749783979999826 ) ) ;
#18610=ORIENTED_EDGE ( 'NONE', *, *, #24844, .F. ) ;
#18612=CARTESIAN_POINT ( 'NONE',  ( 8.124863382020000913, -28.53805538430000155, -20.82664772909999940 ) ) ;
#18613=CARTESIAN_POINT ( 'NONE',  ( -1.981473163719889241, -57.45864759319265147, -23.83876219059375501 ) ) ;
#18625=CARTESIAN_POINT ( 'NONE',  ( 20.64806783649999744, -36.00000000000000000, -10.29738622729999875 ) ) ;
#18626=CARTESIAN_POINT ( 'NONE',  ( 46.84462288190000123, -73.99960224719998791, -2.454903744640000163 ) ) ;
#18627=ORIENTED_EDGE ( 'NONE', *, *, #24110, .T. ) ;
#18629=CARTESIAN_POINT ( 'NONE',  ( -11.43090272393724227, -61.14595846210385588, 20.91059242002400254 ) ) ;
#18630=CARTESIAN_POINT ( 'NONE',  ( -14.69254889179999957, -80.02777972779999516, 36.39670833679999618 ) ) ;
#18632=CARTESIAN_POINT ( 'NONE',  ( -2.733878092589999920, -65.50583529140000394, -26.26633881939999782 ) ) ;
#18633=AXIS2_PLACEMENT_3D ( 'NONE', #17484, #24625, #4814 ) ;
#18634=CARTESIAN_POINT ( 'NONE',  ( -15.42363691649999957, -67.46051858619999564, 22.84488648889999851 ) ) ;
#18635=ORIENTED_EDGE ( 'NONE', *, *, #25179, .F. ) ;
#18638=CARTESIAN_POINT ( 'NONE',  ( 36.69073705870000168, -74.41569028729999502, -14.60033862030000051 ) ) ;
#18640=CARTESIAN_POINT ( 'NONE',  ( 24.75430904529999765, -58.88258727490000410, 1.309835822719999987 ) ) ;
#18641=CARTESIAN_POINT ( 'NONE',  ( 19.46230083649999898, -35.13262238679999427, -8.987746796310000619 ) ) ;
#18645=CARTESIAN_POINT ( 'NONE',  ( -2.587000173290000316, -19.48534420260000033, -23.45837883329999940 ) ) ;
#18646=CARTESIAN_POINT ( 'NONE',  ( 36.75513477746535074, -74.61502060571835671, -14.67454940403652586 ) ) ;
#18647=ORIENTED_EDGE ( 'NONE', *, *, #13034, .T. ) ;
#18648=ADVANCED_FACE ( 'NONE', ( #2636 ), #851, .T. ) ;
#18649=CARTESIAN_POINT ( 'NONE',  ( -12.77207206940000006, -18.50000000000000000, 18.29965927990000196 ) ) ;
#18650=DIRECTION ( 'NONE',  ( -0.9952295494196654602, 0.000000000000000000, 0.09756097560976667582 ) ) ;
#18651=CARTESIAN_POINT ( 'NONE',  ( 8.770435442900000211, -35.38531402059999920, -20.52569425229999922 ) ) ;
#18654=ORIENTED_EDGE ( 'NONE', *, *, #16855, .T. ) ;
#18656=CARTESIAN_POINT ( 'NONE',  ( -7.325370793560000315, -72.00000000000000000, -24.94672208400000102 ) ) ;
#18661=ORIENTED_EDGE ( 'NONE', *, *, #16657, .T. ) ;
#18665=VERTEX_POINT ( 'NONE', #22593 ) ;
#18666=CARTESIAN_POINT ( 'NONE',  ( -17.94180966909999597, -45.73899999920000425, 18.81731824139999887 ) ) ;
#18669=CARTESIAN_POINT ( 'NONE',  ( -19.92984078955770499, -19.50000000000000000, 15.63765909864717152 ) ) ;
#18671=CARTESIAN_POINT ( 'NONE',  ( -10.52744371402527790, -19.48510007433630520, -21.09691113857233802 ) ) ;
#18674=DIRECTION ( 'NONE',  ( 0.000000000000000000, -1.000000000000000000, 0.000000000000000000 ) ) ;
#18675=ORIENTED_EDGE ( 'NONE', *, *, #3085, .T. ) ;
#18676=ADVANCED_FACE ( 'NONE', ( #27250 ), #25267, .T. ) ;
#18677=CARTESIAN_POINT ( 'NONE',  ( -32.77174707999999725, -79.50000000000000000, -21.60034937969999902 ) ) ;
#18683=CARTESIAN_POINT ( 'NONE',  ( 9.356041104380000917, -84.00000000000000000, 37.60355029590000697 ) ) ;
#18685=AXIS2_PLACEMENT_3D ( 'NONE', #16775, #5698, #14581 ) ;
#18687=CARTESIAN_POINT ( 'NONE',  ( 4.882943008269999509E-15, -69.50000000000000000, -40.00000000000000000 ) ) ;
#18689=CARTESIAN_POINT ( 'NONE',  ( -20.03437290520000147, -32.66150190460000147, 14.54837859389999899 ) ) ;
#18691=CARTESIAN_POINT ( 'NONE',  ( 27.75394116159999669, -74.50000000000000000, -27.75394116159999669 ) ) ;
#18693=CARTESIAN_POINT ( 'NONE',  ( 23.71521856880000101, -60.21977178070000036, -9.629174062080000596 ) ) ;
#18695=DIRECTION ( 'NONE',  ( 1.000000000000000000, 0.000000000000000000, 0.000000000000000000 ) ) ;
#18696=CARTESIAN_POINT ( 'NONE',  ( 20.54661061919999554, -36.04663673480000341, -9.151657597179999826 ) ) ;
#18698=VERTEX_POINT ( 'NONE', #24272 ) ;
#18700=PLANE ( 'NONE',  #10165 ) ;
#18701=CARTESIAN_POINT ( 'NONE',  ( -11.34376786329999831, -18.85523522049999912, -18.72653253400000040 ) ) ;
#18702=CIRCLE ( 'NONE', #21927, 7.249999999999999112 ) ;
#18705=CARTESIAN_POINT ( 'NONE',  ( 1.509903313490000218E-14, -80.00000000000000000, 40.00000000000000000 ) ) ;
#18707=CARTESIAN_POINT ( 'NONE',  ( 10.20110288159999890, -74.00000000000000000, 41.00000000000000000 ) ) ;
#18709=EDGE_CURVE ( 'NONE', #26262, #21465, #3472, .T. ) ;
#18710=CARTESIAN_POINT ( 'NONE',  ( -40.53346806335466113, -74.36482065553560972, 7.230685509125985178 ) ) ;
#18711=DIRECTION ( 'NONE',  ( 0.09756097560976997873, 0.000000000000000000, 0.9952295494196653491 ) ) ;
#18712=FACE_OUTER_BOUND ( 'NONE', #16919, .T. ) ;
#18713=VERTEX_POINT ( 'NONE', #12017 ) ;
#18714=CARTESIAN_POINT ( 'NONE',  ( 19.75624615420000296, -18.86343728519999985, -8.697936434349999857 ) ) ;
#18716=CARTESIAN_POINT ( 'NONE',  ( -0.8522615965990000264, -39.36582103130000121, -22.71500442319999991 ) ) ;
#18718=ADVANCED_FACE ( 'NONE', ( #23118 ), #3164, .F. ) ;
#18719=CARTESIAN_POINT ( 'NONE',  ( -17.94180966909999597, -72.00000000000000000, 18.81731824139999887 ) ) ;
#18722=CARTESIAN_POINT ( 'NONE',  ( 22.46104921339999905, -40.70401306749999293, -9.175396146790001595 ) ) ;
#18723=CARTESIAN_POINT ( 'NONE',  ( -38.79561088340664554, -74.00013394023025626, -7.600490370241675286 ) ) ;
#18726=EDGE_LOOP ( 'NONE', ( #2358, #19156, #26654, #10291, #15314 ) ) ;
#18728=CARTESIAN_POINT ( 'NONE',  ( -22.00249031559999935, -74.50000000000000000, -32.67527180329999936 ) ) ;
#18731=EDGE_CURVE ( 'NONE', #21679, #26473, #5272, .T. ) ;
#18732=CARTESIAN_POINT ( 'NONE',  ( 21.24009719620000070, -34.72971490739999467, -7.623606132409999958 ) ) ;
#18733=CARTESIAN_POINT ( 'NONE',  ( 36.67694313739999501, -80.46520755129999714, -13.97975614370000130 ) ) ;
#18739=DIRECTION ( 'NONE',  ( -0.04116274481150321296, -0.9430444279530652008, 0.3301103381390215752 ) ) ;
#18740=DIRECTION ( 'NONE',  ( -1.000000000000000000, 0.000000000000000000, 1.203338504110000538E-16 ) ) ;
#18743=CARTESIAN_POINT ( 'NONE',  ( -16.86265888959999870, -77.00000000000000000, 45.21850545039999503 ) ) ;
#18744=EDGE_CURVE ( 'NONE', #3120, #21366, #16425, .T. ) ;
#18747=CARTESIAN_POINT ( 'NONE',  ( -7.588109730960000299, -73.99999952349999432, 38.87068334559999983 ) ) ;
#18753=B_SPLINE_SURFACE_WITH_KNOTS ( 'NONE', 5, 5, ( 
 ( #4537, #28704, #26697, #24060, #8892, #15012 ),
 ( #21883, #13415, #22318, #2365, #8610, #197 ),
 ( #24501, #24359, #15447, #20127, #8464, #11219 ),
 ( #6737, #1934, #19686, #15602, #17951, #9046 ),
 ( #2080, #17806, #3963, #10920, #26543, #13120 ),
 ( #6139, #10629, #23925, #19974, #19827, #12824 ) ),
 .UNSPECIFIED., .F., .F., .F.,
 ( 6, 6 ),
 ( 6, 6 ),
 ( 13.75713939520000118, 20.91598888789999933 ),
 ( 0.000000000000000000, 2.000000000000000000 ),
 .UNSPECIFIED. ) ;
#18754=DIRECTION ( 'NONE',  ( 1.000000000000000000, 0.000000000000000000, 0.000000000000000000 ) ) ;
#18756=FACE_OUTER_BOUND ( 'NONE', #22347, .T. ) ;
#18759=LINE ( 'NONE', #27920, #3688 ) ;
#18764=CARTESIAN_POINT ( 'NONE',  ( -1.979299272550000266, -58.31202229489999667, -23.87650549820000023 ) ) ;
#18768=ORIENTED_EDGE ( 'NONE', *, *, #18003, .T. ) ;
#18773=DIRECTION ( 'NONE',  ( 1.000000000000000000, 0.000000000000000000, 0.000000000000000000 ) ) ;
#18777=ORIENTED_EDGE ( 'NONE', *, *, #8829, .F. ) ;
#18778=CARTESIAN_POINT ( 'NONE',  ( -14.53416873709999990, -79.85300529469999731, 36.65982618790000203 ) ) ;
#18780=B_SPLINE_CURVE_WITH_KNOTS ( 'NONE', 3,
 ( #18165, #15521, #22689, #277, #8818, #9119, #26918, #24431, #11138, #27063, #4469, #18321, #11588, #22242, #4908, #7107, #122, #15970, #6958, #8973, #15820, #26778, #24732, #4614, #13489, #4767, #13788, #12313, #9700, #23407, #714, #18465, #7555, #27918 ),
 .UNSPECIFIED., .F., .F.,
 ( 4, 2, 2, 2, 1, 1, 2, 2, 2, 2, 1, 1, 2, 2, 2, 2, 2, 2, 4 ),
 ( 0.000000000000000000, 0.1249999999998953615, 0.1874999999998430145, 0.2187499999998188394, 0.2343749999998089584, 0.2421874999998039901, 0.2460937499998017697, 0.2499999999997995492, 0.3749999999998058220, 0.4374999999998089306, 0.4687499999998105404, 0.4843749999998114841, 0.4921874999998120392, 0.4999999999998125944, 0.6249999999998588907, 0.6874999999998817612, 0.7187499999998936406, 0.7499999999999054090, 1.000000000000000000 ),
 .UNSPECIFIED. ) ;
#18781=CARTESIAN_POINT ( 'NONE',  ( -4.234949299229999298, -72.18744871750000414, -28.56489076020000439 ) ) ;
#18784=ORIENTED_EDGE ( 'NONE', *, *, #5287, .T. ) ;
#18785=CARTESIAN_POINT ( 'NONE',  ( 36.28164463560000286, -74.50000004449999835, -14.97346875809999922 ) ) ;
#18787=CARTESIAN_POINT ( 'NONE',  ( 25.16410386810000333, -61.75794029819999764, 1.280048851440000135 ) ) ;
#18788=CARTESIAN_POINT ( 'NONE',  ( -20.33184189050000157, -61.83390236249999816, 14.43150019080000135 ) ) ;
#18789=ORIENTED_EDGE ( 'NONE', *, *, #7502, .T. ) ;
#18791=CARTESIAN_POINT ( 'NONE',  ( -2.647422304290000472, -19.49009541680000268, -23.73806674440000108 ) ) ;
#18794=AXIS2_PLACEMENT_3D ( 'NONE', #26803, #18048, #26945 ) ;
#18796=CARTESIAN_POINT ( 'NONE',  ( -31.99666054769999946, -74.00000000000000000, -22.02415758960000147 ) ) ;
#18798=DIRECTION ( 'NONE',  ( 0.000000000000000000, -1.000000000000000000, 0.000000000000000000 ) ) ;
#18805=ORIENTED_EDGE ( 'NONE', *, *, #3041, .T. ) ;
#18806=CARTESIAN_POINT ( 'NONE',  ( 46.18304991175620700, -73.53220734123081570, -3.800088742014810173 ) ) ;
#18808=CARTESIAN_POINT ( 'NONE',  ( -13.33147262089999963, -42.22514961549999413, 20.36865418349999857 ) ) ;
#18810=EDGE_CURVE ( 'NONE', #11457, #10298, #18327, .T. ) ;
#18811=VERTEX_POINT ( 'NONE', #16550 ) ;
#18813=EDGE_CURVE ( 'NONE', #13063, #16727, #23943, .T. ) ;
#18814=VECTOR ( 'NONE', #1617, 1000.000000000000000 ) ;
#18816=CARTESIAN_POINT ( 'NONE',  ( 40.37851622870000057, -74.24288085019999528, 7.248115061030000028 ) ) ;
#18817=DIRECTION ( 'NONE',  ( 1.000000000000000000, 0.000000000000000000, 0.000000000000000000 ) ) ;
#18818=CARTESIAN_POINT ( 'NONE',  ( -11.70907145606914135, -62.05375851120123087, -23.11666430726260657 ) ) ;
#18819=CARTESIAN_POINT ( 'NONE',  ( -40.00000000000000000, -84.00000000000000000, 0.000000000000000000 ) ) ;
#18822=CARTESIAN_POINT ( 'NONE',  ( 8.113043078722281365, -34.60505764027403330, -21.05852217749055555 ) ) ;
#18823=DIRECTION ( 'NONE',  ( 0.000000000000000000, 1.000000000000000000, 0.000000000000000000 ) ) ;
#18825=ORIENTED_EDGE ( 'NONE', *, *, #7185, .F. ) ;
#18832=CARTESIAN_POINT ( 'NONE',  ( 7.426814492070000107, -35.28814190290000141, -21.34788074219999743 ) ) ;
#18833=CARTESIAN_POINT ( 'NONE',  ( 27.75394116159999669, -74.50000000000000000, -27.75394116159999669 ) ) ;
#18838=CARTESIAN_POINT ( 'NONE',  ( 5.326862811529999898E-15, -73.00000000000000000, -47.25000000000000000 ) ) ;
#18839=CARTESIAN_POINT ( 'NONE',  ( -13.17060483900000101, -68.28989248250000799, -23.12790341000000183 ) ) ;
#18840=EDGE_CURVE ( 'NONE', #12917, #22615, #2871, .T. ) ;
#18842=CARTESIAN_POINT ( 'NONE',  ( 47.13608539959999888, -74.52720457959999578, -1.647993573179999949 ) ) ;
#18843=LINE ( 'NONE', #23350, #9418 ) ;
#18847=AXIS2_PLACEMENT_3D ( 'NONE', #17885, #26627, #28792 ) ;
#18848=CARTESIAN_POINT ( 'NONE',  ( -18.77458274581442765, -19.20927481204605769, 11.51544471821851445 ) ) ;
#18849=CARTESIAN_POINT ( 'NONE',  ( 7.156454249440000304, -36.57019169040000151, -21.47211211410000331 ) ) ;
#18850=CARTESIAN_POINT ( 'NONE',  ( 40.00000000000000000, -79.00000000000000000, 4.898587196589999938E-15 ) ) ;
#18851=ORIENTED_EDGE ( 'NONE', *, *, #25423, .F. ) ;
#18852=CARTESIAN_POINT ( 'NONE',  ( -39.74699101870318430, -73.82038814073398214, 7.246150394361534630 ) ) ;
#18854=CARTESIAN_POINT ( 'NONE',  ( 26.30230850349999727, -72.70510570390000282, 11.30503913470000121 ) ) ;
#18855=CARTESIAN_POINT ( 'NONE',  ( 22.97877291159999658, -37.99999999279999230, -9.393614097370001303 ) ) ;
#18857=TOROIDAL_SURFACE ( 'NONE', #3934, 6.750000000000000000, 2.000000000000000000 ) ;
#18858=CARTESIAN_POINT ( 'NONE',  ( 20.50116792230000229, -18.85523517670000260, -7.685455265189999885 ) ) ;
#18859=FACE_OUTER_BOUND ( 'NONE', #21419, .T. ) ;
#18860=CARTESIAN_POINT ( 'NONE',  ( -2.572575538410000195, -45.92926717529999792, -24.95080834190000019 ) ) ;
#18861=DIRECTION ( 'NONE',  ( 0.000000000000000000, 1.000000000000000000, 0.000000000000000000 ) ) ;
#18868=CARTESIAN_POINT ( 'NONE',  ( -32.75442352089999787, -74.37394555080000202, -21.60834384349999837 ) ) ;
#18873=EDGE_CURVE ( 'NONE', #26586, #18106, #27430, .T. ) ;
#18875=CARTESIAN_POINT ( 'NONE',  ( 19.92119995959999912, -34.82099949419999518, -8.965452275210001432 ) ) ;
#18876=CARTESIAN_POINT ( 'NONE',  ( 7.249276399906878332, -74.06318173168557450, 40.12703402721685109 ) ) ;
#18884=CARTESIAN_POINT ( 'NONE',  ( 25.86648696739999664, -67.35799165719998882, -10.65566759900000093 ) ) ;
#18887=CARTESIAN_POINT ( 'NONE',  ( -11.29440317008408101, -19.46531115638632059, 19.08176919539176097 ) ) ;
#18888=CARTESIAN_POINT ( 'NONE',  ( -29.16815472389999897, -80.00000000000000000, -29.16815472389999897 ) ) ;
#18892=CARTESIAN_POINT ( 'NONE',  ( 21.99462582090000140, -74.00072165509999422, -32.20449087679999423 ) ) ;
#18893=CARTESIAN_POINT ( 'NONE',  ( -22.94161197439999711, -72.70510790119999456, 17.12593288190000251 ) ) ;
#18897=CARTESIAN_POINT ( 'NONE',  ( 40.00000000000000000, -69.50000000000000000, 2.433892081919999696E-15 ) ) ;
#18898=DIRECTION ( 'NONE',  ( 0.000000000000000000, 1.000000000000000000, 0.000000000000000000 ) ) ;
#18900=CARTESIAN_POINT ( 'NONE',  ( 9.476129726560001743, -36.00000000000000000, -20.06309461059999677 ) ) ;
#18901=ORIENTED_EDGE ( 'NONE', *, *, #20433, .F. ) ;
#18906=EDGE_CURVE ( 'NONE', #11916, #3127, #10385, .T. ) ;
#18911=VERTEX_POINT ( 'NONE', #28047 ) ;
#18914=CARTESIAN_POINT ( 'NONE',  ( 8.904194151329999585, -35.90042246200000164, -20.44172831670000079 ) ) ;
#18917=CARTESIAN_POINT ( 'NONE',  ( -15.08135663260000037, -67.66819252530000028, 22.63088120529999969 ) ) ;
#18921=CARTESIAN_POINT ( 'NONE',  ( 25.30470987589999865, -63.24100619570000248, 1.147374915679999940 ) ) ;
#18922=CARTESIAN_POINT ( 'NONE',  ( 19.45083578249999690, -34.98500792359999423, -8.988292418119998572 ) ) ;
#18923=B_SPLINE_SURFACE_WITH_KNOTS ( 'NONE', 5, 5, ( 
 ( #8941, #26593, #26890, #26449, #387, #2264, #20317, #15496, #15344 ),
 ( #2566, #24260, #7080, #22663, #8792, #2707, #24405, #11561, #20025 ),
 ( #17994, #6929, #4299, #17707, #17851, #20177, #22523, #6481, #9234 ),
 ( #4442, #26749, #15939, #11415, #17556, #15792, #24846, #20470, #19872 ),
 ( #11107, #24702, #11268, #22081, #13171, #2127, #24548, #248, #13613 ),
 ( #13314, #8652, #10962, #6782, #4736, #93, #6634, #28752, #22218 ) ),
 .UNSPECIFIED., .F., .F., .F.,
 ( 6, 6 ),
 ( 6, 3, 6 ),
 ( 20.62672786149999737, 31.13134626069999911 ),
 ( 0.000000000000000000, 1.000000000000000000, 2.000000000000000000 ),
 .UNSPECIFIED. ) ;
#18925=VERTEX_POINT ( 'NONE', #10104 ) ;
#18926=CARTESIAN_POINT ( 'NONE',  ( 9.334872109610000362E-16, -74.00000000000000000, -2.419703924680000090E-15 ) ) ;
#18927=CARTESIAN_POINT ( 'NONE',  ( -7.249922261819999214, -74.00000000000000000, 40.03357376379999977 ) ) ;
#18929=ORIENTED_EDGE ( 'NONE', *, *, #4882, .F. ) ;
#18931=CARTESIAN_POINT ( 'NONE',  ( 7.426814476920000629, -35.28814186609999837, -21.34788074160000093 ) ) ;
#18932=CARTESIAN_POINT ( 'NONE',  ( 37.00594063530000000, -79.99129919269999789, -13.97169134750000019 ) ) ;
#18934=EDGE_CURVE ( 'NONE', #24982, #23662, #5291, .T. ) ;
#18935=CARTESIAN_POINT ( 'NONE',  ( 37.01148927991571469, -79.86867281223175041, -14.24953229101417840 ) ) ;
#18937=ORIENTED_EDGE ( 'NONE', *, *, #26640, .T. ) ;
#18940=ORIENTED_EDGE ( 'NONE', *, *, #19423, .T. ) ;
#18943=ORIENTED_EDGE ( 'NONE', *, *, #13069, .F. ) ;
#18945=VERTEX_POINT ( 'NONE', #19433 ) ;
#18946=CARTESIAN_POINT ( 'NONE',  ( 38.62788781560000473, -74.00000025069999765, 7.627567457969999687 ) ) ;
#18949=CARTESIAN_POINT ( 'NONE',  ( 46.74944134502681692, -79.86660166543690309, -3.328368085118203368 ) ) ;
#18950=EDGE_LOOP ( 'NONE', ( #9915, #22366, #13686, #5030, #19380, #8846, #19843 ) ) ;
#18951=CARTESIAN_POINT ( 'NONE',  ( -32.38674382290000153, -80.50000054920000991, -22.17565024390000161 ) ) ;
#18956=CARTESIAN_POINT ( 'NONE',  ( -2.303924720019999928, -79.89639594039999793, 47.10762694129999772 ) ) ;
#18958=ORIENTED_EDGE ( 'NONE', *, *, #9703, .T. ) ;
#18959=DIRECTION ( 'NONE',  ( 0.000000000000000000, -1.000000000000000000, 0.000000000000000000 ) ) ;
#18960=DIRECTION ( 'NONE',  ( 0.000000000000000000, -1.000000000000000000, 0.000000000000000000 ) ) ;
#18962=CARTESIAN_POINT ( 'NONE',  ( 29.87432578229999791, -73.33171065870000405, -25.19102557209999915 ) ) ;
#18964=CARTESIAN_POINT ( 'NONE',  ( -15.78701020529999965, -72.82938648530000592, 23.94860758700000147 ) ) ;
#18966=TOROIDAL_SURFACE ( 'NONE', #17554, 38.75000000000000000, 0.5000000000000000000 ) ;
#18968=CIRCLE ( 'NONE', #19411, 7.250000000000000000 ) ;
#18970=CARTESIAN_POINT ( 'NONE',  ( -40.26982517637422632, -74.16605908757436794, -7.244980372376159217 ) ) ;
#18971=AXIS2_PLACEMENT_3D ( 'NONE', #21189, #17222, #14743 ) ;
#18972=CARTESIAN_POINT ( 'NONE',  ( 20.80917882690000198, -36.16278974830000692, -9.004964305669998836 ) ) ;
#18976=CARTESIAN_POINT ( 'NONE',  ( 46.85827871259999711, -80.18254846009999426, -2.615703315070000201 ) ) ;
#18977=EDGE_LOOP ( 'NONE', ( #7614, #18937, #1302, #10411, #11445 ) ) ;
#18980=CARTESIAN_POINT ( 'NONE',  ( 0.000000000000000000, -57.47855601759999900, 0.000000000000000000 ) ) ;
#18983=CARTESIAN_POINT ( 'NONE',  ( -11.91266501540000000, -74.50000000000000000, 46.64429291560000479 ) ) ;
#18985=CARTESIAN_POINT ( 'NONE',  ( 26.22877567449999958, -72.82938648530000592, 11.61106382910000079 ) ) ;
#18987=VERTEX_POINT ( 'NONE', #8774 ) ;
#18990=CARTESIAN_POINT ( 'NONE',  ( -14.59012856380000045, -74.40829841730000282, 36.78913623730000637 ) ) ;
#18992=CARTESIAN_POINT ( 'NONE',  ( 5.258016244619999627E-13, -84.00000000000000000, -5.364597654989999396E-13 ) ) ;
#18994=CARTESIAN_POINT ( 'NONE',  ( -1.179554765616546597, -74.20448909913940838, 47.15348454221184227 ) ) ;
#19001=VERTEX_POINT ( 'NONE', #8925 ) ;
#19002=EDGE_CURVE ( 'NONE', #4316, #18713, #28086, .T. ) ;
#19004=CARTESIAN_POINT ( 'NONE',  ( -32.73892504640000567, -79.50000000000048317, -22.13232332860000184 ) ) ;
#19007=CARTESIAN_POINT ( 'NONE',  ( 7.936589523510000355, -35.30313553290000073, -21.23424061160000065 ) ) ;
#19008=CARTESIAN_POINT ( 'NONE',  ( 36.60240428190000017, -80.39630767040000592, -14.17343997929999944 ) ) ;
#19012=DIRECTION ( 'NONE',  ( 1.000000000000000000, 0.000000000000000000, 0.000000000000000000 ) ) ;
#19013=CARTESIAN_POINT ( 'NONE',  ( 19.43643821180000231, -34.66800313659999944, -8.988996541680000618 ) ) ;
#19016=FACE_OUTER_BOUND ( 'NONE', #24860, .T. ) ;
#19017=DIRECTION ( 'NONE',  ( 0.000000000000000000, -1.000000000000000000, 0.000000000000000000 ) ) ;
#19018=ORIENTED_EDGE ( 'NONE', *, *, #5188, .T. ) ;
#19019=CARTESIAN_POINT ( 'NONE',  ( 26.88013615959999925, -70.45756328170000415, -11.38838332670000142 ) ) ;
#19023=CARTESIAN_POINT ( 'NONE',  ( -40.00000000000000000, -73.50000000000000000, 3.397282455350000038E-15 ) ) ;
#19025=CARTESIAN_POINT ( 'NONE',  ( 21.86871528920000074, -73.56645110550000766, -31.55443393359999504 ) ) ;
#19028=CARTESIAN_POINT ( 'NONE',  ( -22.65660754319999626, -72.37489965160000338, 17.66159453560000259 ) ) ;
#19029=CIRCLE ( 'NONE', #24589, 0.5000000000000004441 ) ;
#19030=CARTESIAN_POINT ( 'NONE',  ( -11.85905031950000144, -65.11419048950000388, -23.43762659500000112 ) ) ;
#19031=CARTESIAN_POINT ( 'NONE',  ( -2.583988331150000040, -57.40875702419999982, -25.23271569440000306 ) ) ;
#19032=CARTESIAN_POINT ( 'NONE',  ( 0.000000000000000000, -65.07443093669999712, 0.000000000000000000 ) ) ;
#19033=ORIENTED_EDGE ( 'NONE', *, *, #26724, .T. ) ;
#19034=EDGE_CURVE ( 'NONE', #26062, #8713, #11762, .T. ) ;
#19035=CARTESIAN_POINT ( 'NONE',  ( 4.534235129290000123E-15, -84.50000000000000000, -36.25000000000000000 ) ) ;
#19036=ORIENTED_EDGE ( 'NONE', *, *, #13690, .F. ) ;
#19040=CARTESIAN_POINT ( 'NONE',  ( -19.65068252670000248, -52.63280639840000674, 12.32128691209999971 ) ) ;
#19041=CIRCLE ( 'NONE', #13451, 4.750000000000000888 ) ;
#19042=CIRCLE ( 'NONE', #23689, 0.5000000000000004441 ) ;
#19045=ORIENTED_EDGE ( 'NONE', *, *, #7396, .F. ) ;
#19046=DIRECTION ( 'NONE',  ( 0.4794255386042036715, 0.000000000000000000, 0.8775825618903724257 ) ) ;
#19050=CARTESIAN_POINT ( 'NONE',  ( 7.766330995219999700, -36.89698705200000006, -21.49508235269999901 ) ) ;
#19051=ORIENTED_EDGE ( 'NONE', *, *, #22382, .T. ) ;
#19058=CARTESIAN_POINT ( 'NONE',  ( -20.66721530050000055, -63.24178865179999320, 14.64673528719999851 ) ) ;
#19062=EDGE_CURVE ( 'NONE', #25324, #8136, #5877, .T. ) ;
#19063=CARTESIAN_POINT ( 'NONE',  ( -2.319540309899999819, -19.47458110719999880, -22.80676616219999886 ) ) ;
#19065=EDGE_LOOP ( 'NONE', ( #6223, #24112, #3646, #16154 ) ) ;
#19070=CARTESIAN_POINT ( 'NONE',  ( 36.36273659750000320, -79.72376025959999879, -14.77704751070000100 ) ) ;
#19072=CARTESIAN_POINT ( 'NONE',  ( 36.90024110328112528, -79.72731463880091951, -14.43636043974571415 ) ) ;
#19074=CARTESIAN_POINT ( 'NONE',  ( -2.342296125043147992, -80.31169701321654486, 46.86165116740200887 ) ) ;
#19076=CARTESIAN_POINT ( 'NONE',  ( -19.81272040990000249, -52.63293862049999916, 12.05498172269999912 ) ) ;
#19077=CARTESIAN_POINT ( 'NONE',  ( 45.84677419350000349, -73.50000000000000000, -4.286925650119999709 ) ) ;
#19079=CARTESIAN_POINT ( 'NONE',  ( 22.86992907279999798, -57.41946977150000464, 10.24154027049999982 ) ) ;
#19081=ORIENTED_EDGE ( 'NONE', *, *, #27753, .T. ) ;
#19085=CARTESIAN_POINT ( 'NONE',  ( 39.85902549349999902, -74.23956954010000686, 7.332363420190000092 ) ) ;
#19086=CARTESIAN_POINT ( 'NONE',  ( 8.605625357259999220, -37.33604032199999523, -21.85900819109999915 ) ) ;
#19087=CARTESIAN_POINT ( 'NONE',  ( 19.74602846389999655, -32.73217875680000333, 10.78006621239999951 ) ) ;
#19088=CARTESIAN_POINT ( 'NONE',  ( 7.564829567879999012E-15, -73.00000000000000000, 47.25000000000000000 ) ) ;
#19089=EDGE_LOOP ( 'NONE', ( #14241, #2866, #27583, #13545 ) ) ;
#19090=CARTESIAN_POINT ( 'NONE',  ( -32.20769381950000110, -80.50000045429999318, -22.43272063739999922 ) ) ;
#19091=EDGE_CURVE ( 'NONE', #9130, #13313, #14125, .T. ) ;
#19094=CARTESIAN_POINT ( 'NONE',  ( -1.454765721469999828, -53.83744478090000030, -23.38761430650000150 ) ) ;
#19096=CARTESIAN_POINT ( 'NONE',  ( 30.97095665689999677, -72.00000182920000213, -20.30102787789999752 ) ) ;
#19098=CARTESIAN_POINT ( 'NONE',  ( -7.278395029380000381, -74.00000000000000000, 36.96243111169999906 ) ) ;
#19099=CARTESIAN_POINT ( 'NONE',  ( 7.105427357599999217E-15, -69.00000000000000000, 40.00000000000000000 ) ) ;
#19101=CARTESIAN_POINT ( 'NONE',  ( 31.22904256650000221, -73.17619182029999081, -21.84902289639999751 ) ) ;
#19102=CARTESIAN_POINT ( 'NONE',  ( -13.96509519684253497, -74.00000000000328271, 36.21398730655364062 ) ) ;
#19104=DIRECTION ( 'NONE',  ( 0.000000000000000000, -1.000000000000000000, 0.000000000000000000 ) ) ;
#19109=EDGE_CURVE ( 'NONE', #3210, #8623, #2035, .T. ) ;
#19110=CARTESIAN_POINT ( 'NONE',  ( 21.41825492180000268, -36.11004389149999838, -7.844212321469999694 ) ) ;
#19111=CARTESIAN_POINT ( 'NONE',  ( 21.26282345629999782, -36.17810633689999378, -8.125022609230001081 ) ) ;
#19112=CARTESIAN_POINT ( 'NONE',  ( 5.988482279510000053E-15, -69.00000000000000000, 40.00000000000000000 ) ) ;
#19117=DIRECTION ( 'NONE',  ( 1.000000000000000000, 0.000000000000000000, 0.000000000000000000 ) ) ;
#19119=AXIS2_PLACEMENT_3D ( 'NONE', #20136, #17958, #12251 ) ;
#19121=AXIS2_PLACEMENT_3D ( 'NONE', #5441, #3401, #18711 ) ;
#19124=VERTEX_POINT ( 'NONE', #11987 ) ;
#19125=CARTESIAN_POINT ( 'NONE',  ( 19.62439614639999874, -18.62065274400000092, -8.477761181410000901 ) ) ;
#19126=B_SPLINE_CURVE_WITH_KNOTS ( 'NONE', 3,
 ( #13373, #13523, #2478, #15855, #24908, #4939, #22434, #11333, #6991, #24765, #4800, #13677, #11621, #13969, #7430, #22582, #2626, #22873, #11474, #9445, #2915, #24462, #4498, #22276, #23440, #20975, #1040, #7584, #27540, #5517, #1173, #27683, #18927 ),
 .UNSPECIFIED., .F., .F.,
 ( 4, 2, 2, 1, 1, 1, 2, 2, 2, 2, 1, 2, 2, 2, 2, 1, 2, 2, 4 ),
 ( 0.000000000000000000, 0.1250000000002373379, 0.1875000000003559930, 0.2187500000004060918, 0.2343750000004311274, 0.2421875000004436451, 0.2460937500004491962, 0.2500000000004547474, 0.3750000000005158096, 0.4375000000005400125, 0.4687500000005451750, 0.4843750000005399015, 0.5000000000005345724, 0.6250000000004063416, 0.6875000000003421707, 0.7187500000003028688, 0.7343750000002831069, 0.7500000000002633449, 1.000000000000000000 ),
 .UNSPECIFIED. ) ;
#19128=CARTESIAN_POINT ( 'NONE',  ( -11.35954001540000036, -74.00000000000000000, 45.25000000000000000 ) ) ;
#19131=VERTEX_POINT ( 'NONE', #20900 ) ;
#19132=CARTESIAN_POINT ( 'NONE',  ( -1.301749480425372862, -74.17765396621948071, 47.13223634305940379 ) ) ;
#19133=FACE_OUTER_BOUND ( 'NONE', #16170, .T. ) ;
#19134=CARTESIAN_POINT ( 'NONE',  ( 9.454036308939999245, -61.76794852879999809, -23.45130291470000117 ) ) ;
#19136=CARTESIAN_POINT ( 'NONE',  ( 21.66730995129999826, -58.31202229489999667, 10.22412929740000109 ) ) ;
#19137=ORIENTED_EDGE ( 'NONE', *, *, #10616, .F. ) ;
#19140=AXIS2_PLACEMENT_3D ( 'NONE', #28467, #19722, #17690 ) ;
#19145=DIRECTION ( 'NONE',  ( 1.000000000000000000, 0.000000000000000000, 0.000000000000000000 ) ) ;
#19148=FACE_OUTER_BOUND ( 'NONE', #7073, .T. ) ;
#19150=ADVANCED_FACE ( 'NONE', ( #13893 ), #9473, .T. ) ;
#19151=CARTESIAN_POINT ( 'NONE',  ( 19.33939820260000175, -31.63434013299999847, -8.993759961960000382 ) ) ;
#19153=ORIENTED_EDGE ( 'NONE', *, *, #17899, .T. ) ;
#19154=DIRECTION ( 'NONE',  ( -0.09756097560976760563, 0.000000000000000000, -0.9952295494196654602 ) ) ;
#19156=ORIENTED_EDGE ( 'NONE', *, *, #15825, .T. ) ;
#19157=ADVANCED_FACE ( 'NONE', ( #2549, #9214 ), #22948, .F. ) ;
#19158=EDGE_CURVE ( 'NONE', #25354, #16270, #15568, .T. ) ;
#19160=DIRECTION ( 'NONE',  ( 1.000000000000000000, 0.000000000000000000, 0.000000000000000000 ) ) ;
#19163=CARTESIAN_POINT ( 'NONE',  ( 20.31705537619999902, -73.45782167609999647, -31.51289803219999541 ) ) ;
#19164=AXIS2_PLACEMENT_3D ( 'NONE', #20390, #14131, #1277 ) ;
#19166=CARTESIAN_POINT ( 'NONE',  ( -11.90443934750000032, -64.24504445130001784, -23.68393507400000075 ) ) ;
#19167=CARTESIAN_POINT ( 'NONE',  ( 6.948750308559999311, -36.56992524569999858, -21.53806860960000336 ) ) ;
#19169=VERTEX_POINT ( 'NONE', #12129 ) ;
#19170=CARTESIAN_POINT ( 'NONE',  ( -11.18243144779999909, -57.47855601759999900, 20.51090144570000007 ) ) ;
#19171=ORIENTED_EDGE ( 'NONE', *, *, #19339, .T. ) ;
#19173=CIRCLE ( 'NONE', #10774, 28.68388914670000034 ) ;
#19174=CARTESIAN_POINT ( 'NONE',  ( -2.719187978309999920, -64.35840732030000311, -26.13123539399999729 ) ) ;
#19181=CARTESIAN_POINT ( 'NONE',  ( 21.55427193970000133, -36.12241491659999326, -6.846103682259999879 ) ) ;
#19182=EDGE_LOOP ( 'NONE', ( #7564, #2051, #5457 ) ) ;
#19183=CARTESIAN_POINT ( 'NONE',  ( 7.665546204827036192, -37.34293801103260080, -21.51184040533545527 ) ) ;
#19184=ADVANCED_FACE ( 'NONE', ( #3675 ), #21084, .T. ) ;
#19188=CARTESIAN_POINT ( 'NONE',  ( -32.72541325773076437, -74.26385168283852067, -22.20255679915483782 ) ) ;
#19189=CARTESIAN_POINT ( 'NONE',  ( -9.476764215410000247, -80.50000000000000000, 38.08875739639999836 ) ) ;
#19195=CARTESIAN_POINT ( 'NONE',  ( -2.619606476369999992, -19.50000008899999671, -24.29997799710000095 ) ) ;
#19197=ORIENTED_EDGE ( 'NONE', *, *, #10792, .F. ) ;
#19199=CARTESIAN_POINT ( 'NONE',  ( -31.89935321680000158, -74.00000000000000000, -21.99985828019999801 ) ) ;
#19200=CARTESIAN_POINT ( 'NONE',  ( -20.56018235820000228, -57.40875686090000585, 14.85415984670000000 ) ) ;
#19202=B_SPLINE_SURFACE_WITH_KNOTS ( 'NONE', 5, 5, ( 
 ( #3609, #3477, #14404, #23570, #20829, #19195 ),
 ( #25352, #16730, #14533, #23157, #5236, #16447 ),
 ( #16589, #25625, #5655, #5381, #3202, #18791 ),
 ( #25482, #23294, #12340, #25764, #10285, #18645 ),
 ( #14676, #14264, #21249, #10142, #3338, #19063 ),
 ( #14121, #889, #1442, #12205, #21117, #28083 ),
 ( #1300, #27947, #16295, #21381, #7984, #5793 ),
 ( #9732, #12470, #25205, #12060, #23019, #3069 ),
 ( #23706, #17146, #1581, #6062, #25897, #10422 ) ),
 .UNSPECIFIED., .F., .F., .F.,
 ( 6, 3, 6 ),
 ( 6, 6 ),
 ( 0.000000000000000000, 2.252774941520000240, 5.576981603780000185 ),
 ( 0.000000000000000000, 1.000000000000000000 ),
 .UNSPECIFIED. ) ;
#19203=CARTESIAN_POINT ( 'NONE',  ( 36.72530057213035803, -79.26975512441563865, -14.72286002414454309 ) ) ;
#19205=B_SPLINE_CURVE_WITH_KNOTS ( 'NONE', 3,
 ( #24893, #22570, #16131, #20516, #20962, #22859, #2901, #11759, #7413, #13804, #2751, #22709, #11458, #11607, #585, #20672, #18337, #9581, #27226, #7266, #732, #7570, #18482, #20813, #876, #16276, #25191, #5222, #16430, #14106, #3054, #9718 ),
 .UNSPECIFIED., .F., .F.,
 ( 4, 2, 1, 1, 1, 2, 2, 2, 1, 1, 1, 2, 2, 2, 1, 1, 1, 1, 2, 2, 4 ),
 ( 0.000000000000000000, 0.1250000000000754119, 0.1875000000001171285, 0.2187500000001439682, 0.2343750000001598166, 0.2421875000001667277, 0.2500000000001736389, 0.3750000000001862954, 0.4375000000001967315, 0.4687500000002018941, 0.4843750000002002842, 0.4921875000002037259, 0.5000000000002071676, 0.6250000000002902123, 0.6875000000003331779, 0.7187500000003561595, 0.7343750000003677059, 0.7421875000003733680, 0.7460937500003761436, 0.7500000000003789191, 1.000000000000000000 ),
 .UNSPECIFIED. ) ;
#19210=CARTESIAN_POINT ( 'NONE',  ( 20.98165098409999985, -53.83744478090000030, 10.43394308190000075 ) ) ;
#19212=CARTESIAN_POINT ( 'NONE',  ( -7.314390784529999578, -73.97626148509999666, -39.54176628510000313 ) ) ;
#19217=CARTESIAN_POINT ( 'NONE',  ( 22.92823879609795057, -37.07368284069996633, -9.571688886919444528 ) ) ;
#19219=ORIENTED_EDGE ( 'NONE', *, *, #27147, .F. ) ;
#19220=FACE_OUTER_BOUND ( 'NONE', #826, .T. ) ;
#19221=CARTESIAN_POINT ( 'NONE',  ( 22.97877291159999658, -37.99999999279999230, -9.393614097370001303 ) ) ;
#19223=ORIENTED_EDGE ( 'NONE', *, *, #20569, .F. ) ;
#19228=EDGE_LOOP ( 'NONE', ( #4633, #7172, #15584, #12995 ) ) ;
#19230=CARTESIAN_POINT ( 'NONE',  ( -3.562216355159999903, -80.49999996399999702, 46.31451622859999873 ) ) ;
#19231=CARTESIAN_POINT ( 'NONE',  ( -18.99880662649999863, -18.62181730670000235, 14.46168826759999959 ) ) ;
#19235=CARTESIAN_POINT ( 'NONE',  ( 38.67409491847346459, -73.94611239985914608, 7.370697001239634005 ) ) ;
#19236=DIRECTION ( 'NONE',  ( 1.000000000000000000, 0.000000000000000000, 0.000000000000000000 ) ) ;
#19237=DIRECTION ( 'NONE',  ( 1.000000000000000000, 0.000000000000000000, 0.000000000000000000 ) ) ;
#19238=CIRCLE ( 'NONE', #21567, 3.000000000000000000 ) ;
#19239=EDGE_CURVE ( 'NONE', #6357, #15974, #18395, .T. ) ;
#19241=EDGE_CURVE ( 'NONE', #7122, #27225, #3872, .T. ) ;
#19242=AXIS2_PLACEMENT_3D ( 'NONE', #1077, #5418, #5831 ) ;
#19243=CARTESIAN_POINT ( 'NONE',  ( 19.54737287369999876, -35.65078480380000059, -9.004240688089998557 ) ) ;
#19244=ORIENTED_EDGE ( 'NONE', *, *, #18813, .T. ) ;
#19246=CARTESIAN_POINT ( 'NONE',  ( 20.25798860239999755, -35.94310217329999801, -9.093914510570000331 ) ) ;
#19248=ORIENTED_EDGE ( 'NONE', *, *, #17367, .F. ) ;
#19255=TOROIDAL_SURFACE ( 'NONE', #28093, 7.750000000000000000, 0.5000000000000000000 ) ;
#19260=CARTESIAN_POINT ( 'NONE',  ( -13.07632843636527475, -19.48670010342060976, 19.73696929114215237 ) ) ;
#19262=ORIENTED_EDGE ( 'NONE', *, *, #14508, .T. ) ;
#19263=CARTESIAN_POINT ( 'NONE',  ( 19.70300571909999832, -18.50000000000000000, -8.011708434370000020 ) ) ;
#19264=CARTESIAN_POINT ( 'NONE',  ( -14.58326278150000022, -74.39167553240000075, 36.61803022830000032 ) ) ;
#19266=LINE ( 'NONE', #28701, #27549 ) ;
#19267=ORIENTED_EDGE ( 'NONE', *, *, #17934, .F. ) ;
#19269=CARTESIAN_POINT ( 'NONE',  ( 2.842170943039999687E-14, -72.82938648530000592, 1.776356839399999804E-15 ) ) ;
#19271=ADVANCED_FACE ( 'NONE', ( #8313 ), #16640, .T. ) ;
#19276=CARTESIAN_POINT ( 'NONE',  ( 20.65722554970000147, -57.91738531389999878, 10.94680766110000114 ) ) ;
#19277=DIRECTION ( 'NONE',  ( 0.000000000000000000, 1.000000000000000000, 0.000000000000000000 ) ) ;
#19278=ORIENTED_EDGE ( 'NONE', *, *, #6922, .T. ) ;
#19281=TOROIDAL_SURFACE ( 'NONE', #10412, 13.00000000000000000, 2.000000000000000000 ) ;
#19282=ADVANCED_FACE ( 'NONE', ( #17214 ), #7634, .T. ) ;
#19283=EDGE_CURVE ( 'NONE', #898, #21056, #9925, .T. ) ;
#19286=CIRCLE ( 'NONE', #6732, 2.500000000000000444 ) ;
#19288=ORIENTED_EDGE ( 'NONE', *, *, #21964, .T. ) ;
#19293=ORIENTED_EDGE ( 'NONE', *, *, #1993, .F. ) ;
#19302=CARTESIAN_POINT ( 'NONE',  ( 26.57254216609999986, -73.97490553219999754, -28.93874024099999787 ) ) ;
#19303=SPHERICAL_SURFACE ( 'NONE', #11331, 2.000000035459999825 ) ;
#19304=EDGE_CURVE ( 'NONE', #9596, #28564, #13650, .T. ) ;
#19305=EDGE_CURVE ( 'NONE', #28456, #178, #25768, .T. ) ;
#19306=CARTESIAN_POINT ( 'NONE',  ( -21.60034937969999902, -82.25000000000000000, -32.77174707999999725 ) ) ;
#19307=CARTESIAN_POINT ( 'NONE',  ( -19.03439102309033260, -19.48534489991826746, 13.93933370342093170 ) ) ;
#19309=CARTESIAN_POINT ( 'NONE',  ( 0.000000000000000000, -42.50000000000000000, 0.000000000000000000 ) ) ;
#19312=FACE_OUTER_BOUND ( 'NONE', #8522, .T. ) ;
#19314=B_SPLINE_CURVE_WITH_KNOTS ( 'NONE', 5,
 ( #19564, #19841, #15312, #1530, #13139, #10375 ),
 .UNSPECIFIED., .F., .F.,
 ( 6, 6 ),
 ( 0.000000000000000000, 1.000000000000000000 ),
 .UNSPECIFIED. ) ;
#19316=CARTESIAN_POINT ( 'NONE',  ( 22.97877291129999833, -37.68584072819999875, -9.393614098449999616 ) ) ;
#19318=ORIENTED_EDGE ( 'NONE', *, *, #16193, .F. ) ;
#19319=CARTESIAN_POINT ( 'NONE',  ( -2.618120360420000292, -61.37513324760000444, -25.61258802169999882 ) ) ;
#19326=AXIS2_PLACEMENT_3D ( 'NONE', #25930, #28387, #17325 ) ;
#19329=CARTESIAN_POINT ( 'NONE',  ( 4.426600958609999879E-15, -79.00000000000000000, 43.75000000000000000 ) ) ;
#19333=CARTESIAN_POINT ( 'NONE',  ( 21.70051260119999625, -18.62107711730000048, 9.116757753519999952 ) ) ;
#19334=CARTESIAN_POINT ( 'NONE',  ( 23.35417726449999876, -57.47855601710000428, -0.5711878197419999470 ) ) ;
#19335=DIRECTION ( 'NONE',  ( 1.000000000000000000, 0.000000000000000000, 0.000000000000000000 ) ) ;
#19339=EDGE_CURVE ( 'NONE', #2162, #10257, #23444, .T. ) ;
#19343=ADVANCED_FACE ( 'NONE', ( #18349 ), #20840, .F. ) ;
#19345=CARTESIAN_POINT ( 'NONE',  ( 37.06867693649999751, -79.93087181439999256, -14.15266191389999939 ) ) ;
#19347=EDGE_CURVE ( 'NONE', #25813, #16909, #24302, .T. ) ;
#19351=CARTESIAN_POINT ( 'NONE',  ( -1.780211689454020751, -80.14649671107554241, 47.02804128279894513 ) ) ;
#19355=CARTESIAN_POINT ( 'NONE',  ( 20.45876929980000369, -56.26715181569999658, 11.18963356429999934 ) ) ;
#19356=FACE_OUTER_BOUND ( 'NONE', #12860, .T. ) ;
#19357=CARTESIAN_POINT ( 'NONE',  ( -7.305170733980000719, -74.19145785139998850, -39.89387480210000092 ) ) ;
#19358=EDGE_LOOP ( 'NONE', ( #15597, #23562, #26306, #13525 ) ) ;
#19359=CARTESIAN_POINT ( 'NONE',  ( 9.807088892109998568, -36.00000000000000000, -20.27618918270000137 ) ) ;
#19361=CARTESIAN_POINT ( 'NONE',  ( 22.70406349567018722, -37.99004392654882878, -9.315656979556900197 ) ) ;
#19363=CARTESIAN_POINT ( 'NONE',  ( -2.481488253459999793, -18.50000000000000000, -21.63557997309999692 ) ) ;
#19365=CARTESIAN_POINT ( 'NONE',  ( 19.55068592539999983, -35.72724453810000256, -9.038647860560001135 ) ) ;
#19372=EDGE_LOOP ( 'NONE', ( #5795, #12218, #15011, #22694 ) ) ;
#19374=CARTESIAN_POINT ( 'NONE',  ( -19.41104744409999938, -19.40610837510000053, 14.28697461880000041 ) ) ;
#19375=CARTESIAN_POINT ( 'NONE',  ( 38.71640881029999548, -73.50000064450000536, 7.135467304789999687 ) ) ;
#19376=CARTESIAN_POINT ( 'NONE',  ( 7.356933064080000584, -36.56811125840000187, -21.47791245320000186 ) ) ;
#19377=CARTESIAN_POINT ( 'NONE',  ( -14.07395139057579669, -74.01137367045767235, 36.22381386828725169 ) ) ;
#19379=DIRECTION ( 'NONE',  ( -1.000000000000000000, 0.000000000000000000, 0.000000000000000000 ) ) ;
#19380=ORIENTED_EDGE ( 'NONE', *, *, #2685, .T. ) ;
#19381=DIRECTION ( 'NONE',  ( 0.000000000000000000, 1.000000000000000000, 0.000000000000000000 ) ) ;
#19382=CARTESIAN_POINT ( 'NONE',  ( 20.12810827960000282, -35.68342701319999577, -8.993407668519999731 ) ) ;
#19383=VERTEX_POINT ( 'NONE', #17003 ) ;
#19384=CARTESIAN_POINT ( 'NONE',  ( 21.44636399800000248, -36.83820790320000782, -8.385252985220001065 ) ) ;
#19385=DIRECTION ( 'NONE',  ( 0.000000000000000000, 1.000000000000000000, 0.000000000000000000 ) ) ;
#19390=CARTESIAN_POINT ( 'NONE',  ( 7.952618468089998949, -53.29009989829999938, -22.02398067749999910 ) ) ;
#19392=ORIENTED_EDGE ( 'NONE', *, *, #5632, .F. ) ;
#19394=CARTESIAN_POINT ( 'NONE',  ( 23.09634100869999784, -49.87554870529999818, -0.2593201272430000204 ) ) ;
#19395=CARTESIAN_POINT ( 'NONE',  ( 23.44226622849999941, -65.21231684830000574, 10.79519211999999939 ) ) ;
#19400=CARTESIAN_POINT ( 'NONE',  ( -14.59431547039999977, -74.43317772470001614, 36.62860707189999943 ) ) ;
#19402=DIRECTION ( 'NONE',  ( 0.000000000000000000, 1.000000000000000000, 0.000000000000000000 ) ) ;
#19403=ORIENTED_EDGE ( 'NONE', *, *, #865, .T. ) ;
#19404=VECTOR ( 'NONE', #8996, 1000.000000000000000 ) ;
#19405=EDGE_CURVE ( 'NONE', #13313, #8306, #17576, .T. ) ;
#19406=CARTESIAN_POINT ( 'NONE',  ( -1.240000067321601396, -74.19110756884491309, 47.14321378798046425 ) ) ;
#19409=CARTESIAN_POINT ( 'NONE',  ( -12.07234849260000153, -68.56747070539999811, -25.18735587219999772 ) ) ;
#19410=CARTESIAN_POINT ( 'NONE',  ( 20.53475899579999719, -58.35721741809999941, 11.22800282539999905 ) ) ;
#19411=AXIS2_PLACEMENT_3D ( 'NONE', #7889, #16912, #10183 ) ;
#19412=DIRECTION ( 'NONE',  ( 0.000000000000000000, -1.000000000000000000, 0.000000000000000000 ) ) ;
#19413=ORIENTED_EDGE ( 'NONE', *, *, #17123, .F. ) ;
#19416=VECTOR ( 'NONE', #11856, 1000.000000000000000 ) ;
#19417=CARTESIAN_POINT ( 'NONE',  ( 8.956866503930001500, -35.50841500800000716, -20.05333527200000177 ) ) ;
#19418=CARTESIAN_POINT ( 'NONE',  ( 22.06868239059999937, -18.50000000000000000, 1.779150257960000037 ) ) ;
#19422=STYLED_ITEM ( 'NONE', ( #15171 ), #15722 ) ;
#19423=EDGE_CURVE ( 'NONE', #2030, #10820, #21139, .T. ) ;
#19425=CARTESIAN_POINT ( 'NONE',  ( -10.50000000000000000, -19.00000000000000000, 1.748601263780000010E-15 ) ) ;
#19427=DIRECTION ( 'NONE',  ( 0.000000000000000000, 1.000000000000000000, 0.000000000000000000 ) ) ;
#19429=ORIENTED_EDGE ( 'NONE', *, *, #9552, .T. ) ;
#19431=CARTESIAN_POINT ( 'NONE',  ( 22.02882266680000001, -19.46510059719999930, -0.4636565024600000084 ) ) ;
#19433=CARTESIAN_POINT ( 'NONE',  ( -32.77174708219999388, -74.50000000000000000, -21.60034937629999874 ) ) ;
#19434=AXIS2_PLACEMENT_3D ( 'NONE', #18099, #24811, #15607 ) ;
#19435=EDGE_CURVE ( 'NONE', #20924, #3048, #24624, .T. ) ;
#19436=CARTESIAN_POINT ( 'NONE',  ( -23.16987202530000189, -72.82938842069999907, 16.90923852390000093 ) ) ;
#19437=B_SPLINE_SURFACE_WITH_KNOTS ( 'NONE', 5, 5, ( 
 ( #19166, #28053, #21494, #14647, #14774, #1685 ),
 ( #23543, #19030, #27916, #23675, #10524, #19439 ),
 ( #3719, #12579, #19863, #4433, #4576, #22358 ),
 ( #28744, #6625, #24396, #13304, #22209, #238 ),
 ( #7068, #15333, #17549, #11407, #10953, #6774 ),
 ( #15486, #15784, #19725, #1973, #8644, #27025 ) ),
 .UNSPECIFIED., .F., .F., .F.,
 ( 6, 6 ),
 ( 6, 6 ),
 ( 26.13957982610000030, 31.08299525409999831 ),
 ( 0.000000000000000000, 2.000000000000000000 ),
 .UNSPECIFIED. ) ;
#19439=CARTESIAN_POINT ( 'NONE',  ( -12.98506133270000085, -65.72122283929999753, -21.88189319379999986 ) ) ;
#19444=AXIS2_PLACEMENT_3D ( 'NONE', #21692, #10581, #1740 ) ;
#19446=CARTESIAN_POINT ( 'NONE',  ( 22.65555239909999941, -37.06806482060000008, -9.497542709419999341 ) ) ;
#19448=CARTESIAN_POINT ( 'NONE',  ( -1.977440293640000402, -58.73757401350000151, -23.91133900879999885 ) ) ;
#19451=CARTESIAN_POINT ( 'NONE',  ( -19.81272040990000249, -52.63293862049999916, 12.05498172269999912 ) ) ;
#19455=CARTESIAN_POINT ( 'NONE',  ( 21.18066447389999851, -34.91901312109999367, -7.923301732400000574 ) ) ;
#19456=CARTESIAN_POINT ( 'NONE',  ( 7.323177335909999641, -73.87252278319999732, -39.07223452299999167 ) ) ;
#19460=EDGE_CURVE ( 'NONE', #21679, #12727, #26236, .T. ) ;
#19461=CARTESIAN_POINT ( 'NONE',  ( 38.96762186381851478, -74.02518375729582090, 7.561767225083936061 ) ) ;
#19462=CARTESIAN_POINT ( 'NONE',  ( 22.96746030019999907, -18.50000000000000000, 9.091461201590000485 ) ) ;
#19463=CARTESIAN_POINT ( 'NONE',  ( -19.65424240789999999, -57.45864753259999702, 13.63538986699999889 ) ) ;
#19472=CARTESIAN_POINT ( 'NONE',  ( -32.69122048629999711, -74.22019266179999875, -22.19435191799999885 ) ) ;
#19473=VERTEX_POINT ( 'NONE', #28637 ) ;
#19474=TOROIDAL_SURFACE ( 'NONE', #2767, 3.500000000000000000, 0.5000000000000000000 ) ;
#19475=AXIS2_PLACEMENT_3D ( 'NONE', #23817, #1549, #27777 ) ;
#19476=CIRCLE ( 'NONE', #1823, 39.25000000000000000 ) ;
#19481=ORIENTED_EDGE ( 'NONE', *, *, #22890, .T. ) ;
#19482=CARTESIAN_POINT ( 'NONE',  ( 21.05079011269999967, -56.25996389440000200, 10.47764512320000030 ) ) ;
#19485=ORIENTED_EDGE ( 'NONE', *, *, #4825, .T. ) ;
#19489=ADVANCED_FACE ( 'NONE', ( #114 ), #23168, .T. ) ;
#19492=FACE_OUTER_BOUND ( 'NONE', #25176, .T. ) ;
#19495=CARTESIAN_POINT ( 'NONE',  ( -1.282825862340494893, -79.73120692033671730, 47.21063963482292536 ) ) ;
#19504=CARTESIAN_POINT ( 'NONE',  ( 10.20338128179359316, -72.72363397105058880, -26.83891338716990660 ) ) ;
#19505=CARTESIAN_POINT ( 'NONE',  ( -2.597184389209999722, -26.11257328410000156, -24.46312728259999858 ) ) ;
#19506=VERTEX_POINT ( 'NONE', #20490 ) ;
#19507=CARTESIAN_POINT ( 'NONE',  ( 8.271554556730841057, -65.04365450819993555, -23.74272564006271580 ) ) ;
#19510=DIRECTION ( 'NONE',  ( 0.000000000000000000, -1.000000000000000000, 0.000000000000000000 ) ) ;
#19517=CARTESIAN_POINT ( 'NONE',  ( 19.52063838700000176, -35.55398684600000081, -8.985157197580001309 ) ) ;
#19519=CARTESIAN_POINT ( 'NONE',  ( 20.45950369499999866, -35.93889390129999839, -8.926507745990001297 ) ) ;
#19521=ORIENTED_EDGE ( 'NONE', *, *, #22668, .T. ) ;
#19528=CARTESIAN_POINT ( 'NONE',  ( 7.215414233289999757, -74.50000000000000000, -40.70731707320000226 ) ) ;
#19529=CARTESIAN_POINT ( 'NONE',  ( 8.529247663789998768, -49.09615641429999755, -22.06548297080000154 ) ) ;
#19534=CARTESIAN_POINT ( 'NONE',  ( 24.42476859379999965, -57.44036992910000095, 1.191907835489999901 ) ) ;
#19535=CARTESIAN_POINT ( 'NONE',  ( 22.86731741559999875, -66.04885972430001573, 11.50583643109999876 ) ) ;
#19537=ORIENTED_EDGE ( 'NONE', *, *, #203, .T. ) ;
#19538=CARTESIAN_POINT ( 'NONE',  ( -39.69269201139999836, -73.74944613229999391, 7.260205543919999727 ) ) ;
#19539=CIRCLE ( 'NONE', #11636, 30.50381168839999901 ) ;
#19546=CARTESIAN_POINT ( 'NONE',  ( 9.720213298399999147, -61.60483519569999800, -23.97432890940000405 ) ) ;
#19547=CARTESIAN_POINT ( 'NONE',  ( -12.17277134789999948, -67.87585403689999453, -23.96831300490000061 ) ) ;
#19549=CARTESIAN_POINT ( 'NONE',  ( -11.19118494029999944, -42.26701801490000321, -20.14459658370000028 ) ) ;
#19550=ORIENTED_EDGE ( 'NONE', *, *, #16424, .T. ) ;
#19553=B_SPLINE_CURVE_WITH_KNOTS ( 'NONE', 3,
 ( #26339, #4038, #10712, #19076 ),
 .UNSPECIFIED., .F., .F.,
 ( 4, 4 ),
 ( -6.855861996759999855, 0.000000000000000000 ),
 .UNSPECIFIED. ) ;
#19555=CARTESIAN_POINT ( 'NONE',  ( 8.749807307070001983, -35.48126036069999856, -20.57860491179999940 ) ) ;
#19556=CARTESIAN_POINT ( 'NONE',  ( 23.70561558430525295, -62.31684853596433271, 10.61541341332936561 ) ) ;
#19561=AXIS2_PLACEMENT_3D ( 'NONE', #18666, #20993, #3357 ) ;
#19562=EDGE_CURVE ( 'NONE', #28257, #16909, #20937, .T. ) ;
#19564=CARTESIAN_POINT ( 'NONE',  ( -7.627568735119999666, -74.00000000000000000, -38.62788659690000515 ) ) ;
#19566=EDGE_LOOP ( 'NONE', ( #6711, #11722, #17444, #14091 ) ) ;
#19569=ORIENTED_EDGE ( 'NONE', *, *, #5597, .F. ) ;
#19570=CARTESIAN_POINT ( 'NONE',  ( 8.954566937750000122, -35.98146629219999681, -20.48934717840000275 ) ) ;
#19571=ADVANCED_FACE ( 'NONE', ( #3166 ), #1585, .T. ) ;
#19573=ADVANCED_FACE ( 'NONE', ( #16107 ), #15666, .T. ) ;
#19575=CARTESIAN_POINT ( 'NONE',  ( 22.28013210319999970, -18.61865660339999806, 1.245317927350000131 ) ) ;
#19577=CARTESIAN_POINT ( 'NONE',  ( 24.33707037739999990, -62.95235822580000473, -9.864745197619999573 ) ) ;
#19579=CARTESIAN_POINT ( 'NONE',  ( 19.57417645929999850, -18.50000000000000000, -7.622693574120000370 ) ) ;
#19582=CARTESIAN_POINT ( 'NONE',  ( -18.48910831820316858, -19.46665351423196455, 12.47298576395390057 ) ) ;
#19588=CARTESIAN_POINT ( 'NONE',  ( 8.901252876769998323, -18.87168143470000103, -18.93437212940000336 ) ) ;
#19589=VECTOR ( 'NONE', #6853, 1000.000000000000000 ) ;
#19590=CARTESIAN_POINT ( 'NONE',  ( 22.83075791639999608, -36.54217832150000334, -9.915197167589999694 ) ) ;
#19592=CARTESIAN_POINT ( 'NONE',  ( -0.6973805902349998753, -64.04267428580000399, -24.66993619630000012 ) ) ;
#19597=ADVANCED_FACE ( 'NONE', ( #15050 ), #19303, .F. ) ;
#19599=ORIENTED_EDGE ( 'NONE', *, *, #7173, .F. ) ;
#19603=AXIS2_PLACEMENT_3D ( 'NONE', #17949, #11514, #19972 ) ;
#19607=B_SPLINE_CURVE_WITH_KNOTS ( 'NONE', 5,
 ( #23968, #28194, #26885, #24403, #15937, #13762 ),
 .UNSPECIFIED., .F., .F.,
 ( 6, 6 ),
 ( 0.000000000000000000, 1.000000000000000000 ),
 .UNSPECIFIED. ) ;
#19608=CARTESIAN_POINT ( 'NONE',  ( 19.90536779560000014, -32.73235193850000257, 10.48824559260000022 ) ) ;
#19609=CARTESIAN_POINT ( 'NONE',  ( -22.13744763498781509, -74.09767108955308856, -32.45678264336510210 ) ) ;
#19610=CARTESIAN_POINT ( 'NONE',  ( 22.25879350760000008, -18.50000000000000000, 8.634216631190000157 ) ) ;
#19614=CARTESIAN_POINT ( 'NONE',  ( 40.65853658540000026, -84.50000000000000000, 6.717799458580000049 ) ) ;
#19616=CARTESIAN_POINT ( 'NONE',  ( -7.155584660037434652, -73.50000006902133975, 38.82824093549695021 ) ) ;
#19621=CARTESIAN_POINT ( 'NONE',  ( -32.35609092660000385, -74.05570514439999386, -22.11293405780000043 ) ) ;
#19622=ORIENTED_EDGE ( 'NONE', *, *, #23587, .F. ) ;
#19623=AXIS2_PLACEMENT_3D ( 'NONE', #18683, #23329, #2954 ) ;
#19627=ORIENTED_EDGE ( 'NONE', *, *, #24623, .T. ) ;
#19629=EDGE_LOOP ( 'NONE', ( #26047, #16879, #1705, #2297, #11350, #17858, #15422 ) ) ;
#19630=CARTESIAN_POINT ( 'NONE',  ( 22.25602728220000159, -57.44036991819999827, 10.13208872880000122 ) ) ;
#19631=CARTESIAN_POINT ( 'NONE',  ( 46.15163212009999683, -73.78135298099999773, -3.953675005160000477 ) ) ;
#19634=CARTESIAN_POINT ( 'NONE',  ( 22.97877291129812605, -37.68584072819992770, -9.393614098449470262 ) ) ;
#19635=CARTESIAN_POINT ( 'NONE',  ( 9.444779992160000859, -36.00000000019999646, -20.77909504619999836 ) ) ;
#19637=CARTESIAN_POINT ( 'NONE',  ( -1.938080129439999855, -18.50000000000000000, -21.30966978559999703 ) ) ;
#19643=CARTESIAN_POINT ( 'NONE',  ( 10.47579678358301436, -72.64479057567018572, -26.80810721546713893 ) ) ;
#19646=DIRECTION ( 'NONE',  ( -0.4822503909160886226, 0.000000000000000000, 0.8760334242831604445 ) ) ;
#19648=CARTESIAN_POINT ( 'NONE',  ( 9.464545271430450768, -57.41957453194978456, -23.23309258220142226 ) ) ;
#19649=DIRECTION ( 'NONE',  ( -6.123031769110000420E-17, 0.000000000000000000, 1.000000000000000000 ) ) ;
#19652=EDGE_CURVE ( 'NONE', #20968, #21377, #23018, .T. ) ;
#19658=ORIENTED_EDGE ( 'NONE', *, *, #15779, .T. ) ;
#19660=ORIENTED_EDGE ( 'NONE', *, *, #7699, .T. ) ;
#19661=CARTESIAN_POINT ( 'NONE',  ( 21.48608955399999942, -36.92296609210000469, -7.459959442930000684 ) ) ;
#19662=CARTESIAN_POINT ( 'NONE',  ( 9.444187806723459033, -35.99901531098080909, -19.97576011151723563 ) ) ;
#19663=EDGE_LOOP ( 'NONE', ( #16006, #15026 ) ) ;
#19672=CARTESIAN_POINT ( 'NONE',  ( 7.362282719720000479, -57.47832541620000057, -22.17287314020000011 ) ) ;
#19676=FACE_OUTER_BOUND ( 'NONE', #25545, .T. ) ;
#19677=CARTESIAN_POINT ( 'NONE',  ( 26.61465604159999998, -68.28989644159999273, 0.1578853838729999959 ) ) ;
#19678=CARTESIAN_POINT ( 'NONE',  ( 25.93066785690000131, -70.16663891479998938, 10.87636646910000060 ) ) ;
#19679=CARTESIAN_POINT ( 'NONE',  ( 38.71640881029999548, -73.50000064450000536, 7.135467304789999687 ) ) ;
#19686=CARTESIAN_POINT ( 'NONE',  ( 27.92725156619999893, -70.60688442979999024, 1.994915591920000342 ) ) ;
#19688=CARTESIAN_POINT ( 'NONE',  ( 8.600016245219999078, -57.45905972560000663, -22.33353789330000083 ) ) ;
#19689=CARTESIAN_POINT ( 'NONE',  ( -12.22512305319999903, -68.97169036700000788, -24.44138895879999751 ) ) ;
#19690=CARTESIAN_POINT ( 'NONE',  ( 22.25602933960000129, -57.44036955189999816, 10.13208958120000069 ) ) ;
#19691=CARTESIAN_POINT ( 'NONE',  ( 22.85528114059999893, -62.13923587570000251, -7.268368518939999134 ) ) ;
#19692=ORIENTED_EDGE ( 'NONE', *, *, #28767, .F. ) ;
#19697=EDGE_CURVE ( 'NONE', #28649, #2030, #5769, .T. ) ;
#19698=EDGE_CURVE ( 'NONE', #14463, #27919, #10402, .T. ) ;
#19700=ORIENTED_EDGE ( 'NONE', *, *, #8922, .F. ) ;
#19702=CARTESIAN_POINT ( 'NONE',  ( 23.48715812726448249, -61.18336516922612844, 10.53353075793953053 ) ) ;
#19705=CIRCLE ( 'NONE', #13170, 7.250000000000000000 ) ;
#19712=CARTESIAN_POINT ( 'NONE',  ( 8.927245643350000037, -35.93968828110000402, -20.45978054029999882 ) ) ;
#19713=CARTESIAN_POINT ( 'NONE',  ( -40.00000000000000000, -77.00000000000000000, 0.000000000000000000 ) ) ;
#19716=CARTESIAN_POINT ( 'NONE',  ( 21.27670944740000181, -18.50000000000000000, 0.7959958381299999663 ) ) ;
#19717=CARTESIAN_POINT ( 'NONE',  ( -7.627567457969999687, -74.00000025069999765, 38.62788781560000473 ) ) ;
#19720=ORIENTED_EDGE ( 'NONE', *, *, #10014, .F. ) ;
#19722=DIRECTION ( 'NONE',  ( 0.000000000000000000, 1.000000000000000000, 0.000000000000000000 ) ) ;
#19724=CARTESIAN_POINT ( 'NONE',  ( 36.70830950850000107, -75.00000000000000000, -14.75000000000000000 ) ) ;
#19725=CARTESIAN_POINT ( 'NONE',  ( -12.17278359089999995, -67.87586094739999965, -23.96830084060000132 ) ) ;
#19726=AXIS2_PLACEMENT_3D ( 'NONE', #2595, #568, #22399 ) ;
#19728=ORIENTED_EDGE ( 'NONE', *, *, #21481, .T. ) ;
#19729=EDGE_CURVE ( 'NONE', #3141, #212, #14173, .T. ) ;
#19730=CARTESIAN_POINT ( 'NONE',  ( 8.311993592450001245, -18.50000000000000000, -19.17432171929999996 ) ) ;
#19732=ORIENTED_EDGE ( 'NONE', *, *, #10755, .F. ) ;
#19733=CARTESIAN_POINT ( 'NONE',  ( -2.496526366579999934, -62.53529079479999808, -25.29179931070000009 ) ) ;
#19735=CARTESIAN_POINT ( 'NONE',  ( 20.33566493080000015, -36.00000000000000000, -9.885503730140001721 ) ) ;
#19736=CARTESIAN_POINT ( 'NONE',  ( -20.48522561129999886, -53.77454410920000072, 14.80553289520000071 ) ) ;
#19738=VERTEX_POINT ( 'NONE', #4286 ) ;
#19740=CARTESIAN_POINT ( 'NONE',  ( 7.318371247189999984, -73.93831524339999817, -38.68350846249999364 ) ) ;
#19742=CIRCLE ( 'NONE', #23490, 11.00000000000000000 ) ;
#19743=CARTESIAN_POINT ( 'NONE',  ( 8.195672531370084002, -37.94341444778289940, -21.63145225707751251 ) ) ;
#19746=CARTESIAN_POINT ( 'NONE',  ( -9.864287931150000688, -18.50000000000000000, -19.01841465109999874 ) ) ;
#19756=CARTESIAN_POINT ( 'NONE',  ( 23.70177636041242764, -64.50388029674192580, -7.622970390447100009 ) ) ;
#19758=ADVANCED_FACE ( 'NONE', ( #11097 ), #21919, .T. ) ;
#19759=FACE_OUTER_BOUND ( 'NONE', #931, .T. ) ;
#19760=CARTESIAN_POINT ( 'NONE',  ( -32.17865685019999233, -74.02983596709999858, -21.95421844790000065 ) ) ;
#19761=CARTESIAN_POINT ( 'NONE',  ( 0.000000000000000000, -56.78056608349999834, 0.000000000000000000 ) ) ;
#19766=SPHERICAL_SURFACE ( 'NONE', #11096, 2.000000000000000000 ) ;
#19767=CARTESIAN_POINT ( 'NONE',  ( -0.8216735279219999910, -65.07443093669999712, -25.13632616349999793 ) ) ;
#19768=VERTEX_POINT ( 'NONE', #6915 ) ;
#19770=ORIENTED_EDGE ( 'NONE', *, *, #9274, .F. ) ;
#19772=CARTESIAN_POINT ( 'NONE',  ( 36.25000000000000000, -79.00000000000000000, 2.314797894279999601E-15 ) ) ;
#19774=LINE ( 'NONE', #28523, #8490 ) ;
#19775=FACE_OUTER_BOUND ( 'NONE', #175, .T. ) ;
#19776=EDGE_CURVE ( 'NONE', #2148, #9200, #7242, .T. ) ;
#19777=CARTESIAN_POINT ( 'NONE',  ( 8.913589957130000130, -36.23936169889999803, -21.16767038869999951 ) ) ;
#19779=CARTESIAN_POINT ( 'NONE',  ( 26.65586303345174812, -70.93575951088651266, 10.69912789994289959 ) ) ;
#19780=VERTEX_POINT ( 'NONE', #10667 ) ;
#19781=CARTESIAN_POINT ( 'NONE',  ( 36.22844186549999534, -74.00000000000000000, -13.75000000000000000 ) ) ;
#19788=PLANE ( 'NONE',  #28466 ) ;
#19789=ORIENTED_EDGE ( 'NONE', *, *, #5008, .F. ) ;
#19793=CARTESIAN_POINT ( 'NONE',  ( 7.362282589680580358, -57.47832521685436546, -22.17287418770180452 ) ) ;
#19802=ORIENTED_EDGE ( 'NONE', *, *, #23998, .F. ) ;
#19803=CARTESIAN_POINT ( 'NONE',  ( -11.95046964750000029, -49.86907377909999894, 20.00125202210000097 ) ) ;
#19804=CARTESIAN_POINT ( 'NONE',  ( 9.227003638719999401, -35.93081093159999995, -19.61343128729999918 ) ) ;
#19805=ORIENTED_EDGE ( 'NONE', *, *, #15749, .T. ) ;
#19807=EDGE_CURVE ( 'NONE', #1569, #24813, #15044, .T. ) ;
#19808=CARTESIAN_POINT ( 'NONE',  ( -3.331535842216653887, -67.92908815540094736, -27.51829522574995579 ) ) ;
#19809=ORIENTED_EDGE ( 'NONE', *, *, #10146, .F. ) ;
#19811=DIRECTION ( 'NONE',  ( 0.000000000000000000, 1.000000000000000000, 0.000000000000000000 ) ) ;
#19812=CARTESIAN_POINT ( 'NONE',  ( 9.464546293550000655, -57.41957467990000197, -23.23309162749999857 ) ) ;
#19817=DIRECTION ( 'NONE',  ( 0.000000000000000000, 1.000000000000000000, 0.000000000000000000 ) ) ;
#19818=CARTESIAN_POINT ( 'NONE',  ( -14.01337423630000067, -80.50000000000000000, 36.66316738249999929 ) ) ;
#19820=ORIENTED_EDGE ( 'NONE', *, *, #1193, .T. ) ;
#19822=EDGE_CURVE ( 'NONE', #16038, #16955, #10848, .T. ) ;
#19823=CARTESIAN_POINT ( 'NONE',  ( -38.71641004229999794, -73.65707963269998970, 7.135467526410000261 ) ) ;
#19825=DIRECTION ( 'NONE',  ( 0.000000000000000000, 1.000000000000000000, 0.000000000000000000 ) ) ;
#19826=EDGE_LOOP ( 'NONE', ( #4960, #25518, #24553, #6960 ) ) ;
#19827=CARTESIAN_POINT ( 'NONE',  ( 28.55874257110000158, -72.70510787919999984, 2.003337190579999927 ) ) ;
#19830=CARTESIAN_POINT ( 'NONE',  ( -12.08584241179999985, -69.49854687080001270, -25.11440336740000134 ) ) ;
#19831=CARTESIAN_POINT ( 'NONE',  ( -11.62511810790000055, -42.27294335669999725, -19.65139164230000191 ) ) ;
#19833=CARTESIAN_POINT ( 'NONE',  ( 22.17287391930145546, -57.47832537024360988, -7.362282751270468495 ) ) ;
#19840=B_SPLINE_SURFACE_WITH_KNOTS ( 'NONE', 2, 5, ( 
 ( #21397, #23722, #27697, #21538, #27961, #7862 ),
 ( #28227, #1594, #9889, #28097, #8261, #3902 ),
 ( #23310, #3492, #16603, #3626, #1053, #21261 ) ),
 .UNSPECIFIED., .F., .F., .F.,
 ( 3, 3 ),
 ( 6, 6 ),
 ( 6.132304667409999688, 7.821587791749999852 ),
 ( 0.000000000000000000, 0.5000000000000000000 ),
 .UNSPECIFIED. ) ;
#19841=CARTESIAN_POINT ( 'NONE',  ( -7.472970580910000216, -74.00000000000000000, -38.65569705749999940 ) ) ;
#19843=ORIENTED_EDGE ( 'NONE', *, *, #28319, .T. ) ;
#19844=CARTESIAN_POINT ( 'NONE',  ( 26.88798373661718344, -72.41637509537598305, -11.07835129732953483 ) ) ;
#19851=FACE_OUTER_BOUND ( 'NONE', #4197, .T. ) ;
#19853=B_SPLINE_CURVE_WITH_KNOTS ( 'NONE', 5,
 ( #27655, #25876, #14650, #1414, #9852, #18900 ),
 .UNSPECIFIED., .F., .F.,
 ( 6, 6 ),
 ( 0.9548616571615553550, 1.000000000000000000 ),
 .UNSPECIFIED. ) ;
#19856=ADVANCED_FACE ( 'NONE', ( #9454 ), #13828, .T. ) ;
#19858=CARTESIAN_POINT ( 'NONE',  ( 28.33616551327313715, -70.11425052315884443, 2.503553257605046323 ) ) ;
#19859=DIRECTION ( 'NONE',  ( 0.2414462220490755373, 0.000000000000000000, -0.9704142011833032377 ) ) ;
#19860=ADVANCED_FACE ( 'NONE', ( #17921 ), #461, .T. ) ;
#19861=CARTESIAN_POINT ( 'NONE',  ( 6.890073352990000011, -40.75155002679999683, -21.70991749099999879 ) ) ;
#19862=CARTESIAN_POINT ( 'NONE',  ( -38.08875739639999836, -82.25000000000000000, 9.476764215410000247 ) ) ;
#19863=CARTESIAN_POINT ( 'NONE',  ( -12.00432114859999899, -65.97406652869999277, -23.19064400290000094 ) ) ;
#19864=CARTESIAN_POINT ( 'NONE',  ( -17.93028678539999987, -18.50000000000000000, 10.99759328500000066 ) ) ;
#19865=CARTESIAN_POINT ( 'NONE',  ( 0.000000000000000000, -80.50000000000000000, 40.00000000000000000 ) ) ;
#19867=ORIENTED_EDGE ( 'NONE', *, *, #24990, .F. ) ;
#19868=CARTESIAN_POINT ( 'NONE',  ( 9.024081099289999131, -19.49999992740000110, -18.94592230980000380 ) ) ;
#19869=CARTESIAN_POINT ( 'NONE',  ( 21.93565869129999868, -36.00000000000000000, -11.17657094590000000 ) ) ;
#19872=CARTESIAN_POINT ( 'NONE',  ( -14.06310087329999803, -61.59908875819999707, 21.57936076700000072 ) ) ;
#19874=CARTESIAN_POINT ( 'NONE',  ( -12.89904789370000060, -65.07443093669999712, -21.58991903219999742 ) ) ;
#19876=CARTESIAN_POINT ( 'NONE',  ( 19.97124347238408859, -19.47946848935876929, -8.623261867002929293 ) ) ;
#19878=ORIENTED_EDGE ( 'NONE', *, *, #24232, .F. ) ;
#19880=AXIS2_PLACEMENT_3D ( 'NONE', #5996, #5727, #3551 ) ;
#19881=CARTESIAN_POINT ( 'NONE',  ( 7.260629316970000247, -73.82505178009999725, -39.64169929279999849 ) ) ;
#19882=EDGE_LOOP ( 'NONE', ( #3061, #6164, #20839, #1504 ) ) ;
#19884=VERTEX_POINT ( 'NONE', #4947 ) ;
#19888=CARTESIAN_POINT ( 'NONE',  ( 22.35211346940000254, -19.39383846089999963, 9.879721194109999161 ) ) ;
#19889=DIRECTION ( 'NONE',  ( 0.000000000000000000, -1.000000000000000000, 0.000000000000000000 ) ) ;
#19892=CIRCLE ( 'NONE', #23631, 1.000000000000000000 ) ;
#19893=CARTESIAN_POINT ( 'NONE',  ( -13.82310862910000004, -74.00000000000000000, 36.20061004779999791 ) ) ;
#19894=CARTESIAN_POINT ( 'NONE',  ( 8.034825427640001294, -66.63181251129999794, -24.57972215990000109 ) ) ;
#19897=CIRCLE ( 'NONE', #24108, 38.75000000000000000 ) ;
#19900=CARTESIAN_POINT ( 'NONE',  ( -7.225954378397760891, -73.65476501621135696, 39.40991843094596447 ) ) ;
#19901=CARTESIAN_POINT ( 'NONE',  ( 22.65305255325292322, -60.89179363350914542, -7.201864690846052852 ) ) ;
#19903=CARTESIAN_POINT ( 'NONE',  ( -40.00000000000000000, -69.00000000000000000, 3.236300116779999679E-15 ) ) ;
#19904=AXIS2_PLACEMENT_3D ( 'NONE', #26406, #6435, #24222 ) ;
#19907=CARTESIAN_POINT ( 'NONE',  ( -22.71848792900000191, -80.00000000000000000, -32.61798286559999838 ) ) ;
#19909=AXIS2_PLACEMENT_3D ( 'NONE', #14263, #5234, #5082 ) ;
#19913=DIRECTION ( 'NONE',  ( -0.09756097560976716154, 0.000000000000000000, -0.9952295494196655712 ) ) ;
#19915=CARTESIAN_POINT ( 'NONE',  ( 21.02965361369999897, -18.50000000000000000, -0.4426258060200000122 ) ) ;
#19916=CARTESIAN_POINT ( 'NONE',  ( -21.93598400869999665, -79.95692792130000726, -32.60789339819999810 ) ) ;
#19920=CARTESIAN_POINT ( 'NONE',  ( -7.215414233289999757, -82.25000000000000000, 40.70731707320000226 ) ) ;
#19921=DIRECTION ( 'NONE',  ( -0.6405991297529511908, 3.017111016349766299E-15, -0.7678754814159401976 ) ) ;
#19924=EDGE_LOOP ( 'NONE', ( #27714, #20746, #22853, #9283 ) ) ;
#19925=ADVANCED_FACE ( 'NONE', ( #13976 ), #5605, .T. ) ;
#19927=DIRECTION ( 'NONE',  ( 0.000000000000000000, -1.000000000000000000, 0.000000000000000000 ) ) ;
#19928=CARTESIAN_POINT ( 'NONE',  ( 47.25000000000000000, -77.00000000000000000, -13.75000000000000000 ) ) ;
#19931=CARTESIAN_POINT ( 'NONE',  ( 10.85455877420105431, -72.50961925363316141, -26.83546891656583711 ) ) ;
#19932=CARTESIAN_POINT ( 'NONE',  ( -17.93694630730000128, -18.50000000000000000, 13.70495702920000092 ) ) ;
#19936=CARTESIAN_POINT ( 'NONE',  ( 20.30102379280298308, -72.26179938780217071, -30.97095677777052813 ) ) ;
#19940=SHAPE_DEFINITION_REPRESENTATION ( #28051, #10734 ) ;
#19941=CARTESIAN_POINT ( 'NONE',  ( 9.476764215410000247, -74.50000000000000000, 38.08875739639999836 ) ) ;
#19944=CIRCLE ( 'NONE', #5081, 22.03370205219999889 ) ;
#19946=FACE_OUTER_BOUND ( 'NONE', #28090, .T. ) ;
#19947=FACE_OUTER_BOUND ( 'NONE', #22704, .T. ) ;
#19951=AXIS2_PLACEMENT_3D ( 'NONE', #21412, #1469, #26215 ) ;
#19952=ADVANCED_FACE ( 'NONE', ( #26660 ), #6702, .T. ) ;
#19955=AXIS2_PLACEMENT_3D ( 'NONE', #1070, #8151, #7617 ) ;
#19958=DIRECTION ( 'NONE',  ( 1.000000000000000000, 0.000000000000000000, 0.000000000000000000 ) ) ;
#19961=CARTESIAN_POINT ( 'NONE',  ( 22.41768028079999908, -65.59529275500000267, 11.91456822289999984 ) ) ;
#19965=CARTESIAN_POINT ( 'NONE',  ( 23.16587695349999976, -49.87340317219999974, 0.05359468315350000150 ) ) ;
#19966=CARTESIAN_POINT ( 'NONE',  ( 24.11425572830000164, -65.50583529140000394, 10.76556153070000121 ) ) ;
#19967=CARTESIAN_POINT ( 'NONE',  ( 40.38463872053225856, -74.25043946767728187, 7.240437622435978327 ) ) ;
#19970=CARTESIAN_POINT ( 'NONE',  ( -20.52703897250000153, -55.79355142130000900, 14.83226277630000034 ) ) ;
#19972=DIRECTION ( 'NONE',  ( 1.000000000000000000, 0.000000000000000000, 0.000000000000000000 ) ) ;
#19973=VERTEX_POINT ( 'NONE', #18208 ) ;
#19974=CARTESIAN_POINT ( 'NONE',  ( 28.54888737639999974, -72.55114965769999458, 2.312894923860000063 ) ) ;
#19976=CARTESIAN_POINT ( 'NONE',  ( 25.79807934023626714, -74.30236118189925776, -29.52720746065469015 ) ) ;
#19977=CARTESIAN_POINT ( 'NONE',  ( -12.76533745180000068, -68.20220936460000871, -23.31270229540000116 ) ) ;
#19978=CARTESIAN_POINT ( 'NONE',  ( 23.78692593859999960, -64.96416322790000208, -8.575408708140001224 ) ) ;
#19980=AXIS2_PLACEMENT_3D ( 'NONE', #17750, #4481, #2747 ) ;
#19981=ADVANCED_FACE ( 'NONE', ( #20097 ), #6999, .T. ) ;
#19982=CYLINDRICAL_SURFACE ( 'NONE', #11993, 0.9999999999999988898 ) ;
#19983=CARTESIAN_POINT ( 'NONE',  ( -2.645751311070000167, -74.00000000000000000, 46.75000000000000000 ) ) ;
#19987=CARTESIAN_POINT ( 'NONE',  ( -34.89999999999999858, -82.50000000000000000, 0.000000000000000000 ) ) ;
#19989=VERTEX_POINT ( 'NONE', #13685 ) ;
#19990=CARTESIAN_POINT ( 'NONE',  ( 7.229383731089999543, -73.50070240710000746, 39.23650411529999360 ) ) ;
#19992=CARTESIAN_POINT ( 'NONE',  ( 20.04401346829999753, -25.53205114500000050, -8.807493111859999502 ) ) ;
#19993=CARTESIAN_POINT ( 'NONE',  ( 22.66861466926381397, -19.47159664147383751, 0.9610264626648014064 ) ) ;
#19995=ORIENTED_EDGE ( 'NONE', *, *, #499, .F. ) ;
#19996=CARTESIAN_POINT ( 'NONE',  ( 26.81105948361605229, -72.58019056410417136, -10.66796337414779217 ) ) ;
#19998=CARTESIAN_POINT ( 'NONE',  ( 9.090175673379999211, -35.93817878899999840, -20.25147856850000139 ) ) ;
#20000=CARTESIAN_POINT ( 'NONE',  ( 21.51532853426891023, -35.83080157483318118, -6.934509737378918182 ) ) ;
#20003=DIRECTION ( 'NONE',  ( -0.7071067811865474617, 0.000000000000000000, -0.7071067811865474617 ) ) ;
#20004=CARTESIAN_POINT ( 'NONE',  ( 21.41854095929999602, -18.50000000000000000, 0.3037881489800000057 ) ) ;
#20008=CARTESIAN_POINT ( 'NONE',  ( -33.18922156509999866, -79.25000000000000000, -21.87551306609999813 ) ) ;
#20009=CARTESIAN_POINT ( 'NONE',  ( 28.91458899939999938, -72.00000000000000000, 3.086557976320000396 ) ) ;
#20010=DIRECTION ( 'NONE',  ( 0.9704142011833034598, 0.000000000000000000, 0.2414462220490750377 ) ) ;
#20011=DIRECTION ( 'NONE',  ( -0.8940996652532122724, 0.000000000000000000, 0.4478680481951061165 ) ) ;
#20012=DIRECTION ( 'NONE',  ( 0.000000000000000000, -1.000000000000000000, 0.000000000000000000 ) ) ;
#20013=CARTESIAN_POINT ( 'NONE',  ( 25.46584391311435880, -59.75127557667808276, 1.379760577311673675 ) ) ;
#20015=CARTESIAN_POINT ( 'NONE',  ( -40.70731707320000226, -77.00000000000000000, 7.215414233289999757 ) ) ;
#20017=VERTEX_POINT ( 'NONE', #2634 ) ;
#20018=CARTESIAN_POINT ( 'NONE',  ( 7.734359208889999948, -19.46510056589999849, -20.63161901249999985 ) ) ;
#20019=EDGE_CURVE ( 'NONE', #10596, #18106, #4060, .T. ) ;
#20020=AXIS2_PLACEMENT_3D ( 'NONE', #12850, #21765, #28183 ) ;
#20022=ADVANCED_FACE ( 'NONE', ( #10019 ), #27935, .T. ) ;
#20023=ORIENTED_EDGE ( 'NONE', *, *, #10927, .F. ) ;
#20025=CARTESIAN_POINT ( 'NONE',  ( -13.87613801740000063, -58.81368956530000247, 21.27373992140000070 ) ) ;
#20026=CARTESIAN_POINT ( 'NONE',  ( 7.224488193780730150, -74.42768721769506612, 40.61475266869189937 ) ) ;
#20028=EDGE_CURVE ( 'NONE', #26317, #9320, #14891, .T. ) ;
#20030=CARTESIAN_POINT ( 'NONE',  ( -11.07305194678827043, -19.50000000000000000, -24.81486620154639411 ) ) ;
#20031=EDGE_CURVE ( 'NONE', #26140, #7537, #16624, .T. ) ;
#20033=CARTESIAN_POINT ( 'NONE',  ( 19.96747957240500071, -19.47954630362596973, -8.626122652564374604 ) ) ;
#20036=CARTESIAN_POINT ( 'NONE',  ( 7.460698725479999927E-15, -73.50000000000000000, 40.00000000000000000 ) ) ;
#20037=CARTESIAN_POINT ( 'NONE',  ( 29.06613905497733086, -74.35453649132965381, -26.34452374057316604 ) ) ;
#20041=CARTESIAN_POINT ( 'NONE',  ( 22.14137210369998243, -52.59522851919948039, 10.05377507689999028 ) ) ;
#20042=B_SPLINE_CURVE_WITH_KNOTS ( 'NONE', 3,
 ( #28645, #28504, #21529, #26189, #1586, #10425 ),
 .UNSPECIFIED., .F., .F.,
 ( 4, 2, 4 ),
 ( 0.000000000000000000, 0.5000000000000000000, 1.000000000000000000 ),
 .UNSPECIFIED. ) ;
#20046=DIRECTION ( 'NONE',  ( 1.000000000000000000, 0.000000000000000000, 0.000000000000000000 ) ) ;
#20048=AXIS2_PLACEMENT_3D ( 'NONE', #5210, #27070, #27512 ) ;
#20050=CARTESIAN_POINT ( 'NONE',  ( -13.92338919490000038, -74.00000000000000000, 36.27080632649999359 ) ) ;
#20051=CARTESIAN_POINT ( 'NONE',  ( -32.76307242539326836, -79.87735098181109095, -22.39909635432421453 ) ) ;
#20053=ORIENTED_EDGE ( 'NONE', *, *, #5478, .T. ) ;
#20054=CARTESIAN_POINT ( 'NONE',  ( -12.00286543741112766, -72.31233190808829647, -26.16426295086472820 ) ) ;
#20057=CIRCLE ( 'NONE', #1028, 12.00000000000000000 ) ;
#20059=CARTESIAN_POINT ( 'NONE',  ( -40.30310653759999440, -74.34472676629999910, -7.255206491290000059 ) ) ;
#20061=CARTESIAN_POINT ( 'NONE',  ( -31.99658184870000355, -79.50000000000000000, -31.99658184870000355 ) ) ;
#20063=EDGE_CURVE ( 'NONE', #24483, #3233, #5832, .T. ) ;
#20068=CIRCLE ( 'NONE', #8424, 0.5000000000000004441 ) ;
#20070=ORIENTED_EDGE ( 'NONE', *, *, #14908, .F. ) ;
#20075=CARTESIAN_POINT ( 'NONE',  ( 46.59019410810000039, -73.90401672450001058, -3.140090762159999827 ) ) ;
#20076=EDGE_LOOP ( 'NONE', ( #13565, #279, #26935, #26089 ) ) ;
#20078=CARTESIAN_POINT ( 'NONE',  ( -22.22906625010000070, -79.49999999740001044, -32.83566834300000181 ) ) ;
#20080=CARTESIAN_POINT ( 'NONE',  ( 8.855030550580000437, -36.23917065910000446, -21.13310771060000093 ) ) ;
#20082=CARTESIAN_POINT ( 'NONE',  ( 0.000000000000000000, -19.00000000000000000, 0.000000000000000000 ) ) ;
#20086=CARTESIAN_POINT ( 'NONE',  ( -40.34085930499999506, -74.29298176469998793, 7.252015964940000003 ) ) ;
#20087=CARTESIAN_POINT ( 'NONE',  ( -21.85457041760000152, -74.43208506860000284, -32.66023292170000758 ) ) ;
#20088=CARTESIAN_POINT ( 'NONE',  ( -1.451488207819999987, -56.25996389440000200, -23.46934156900000090 ) ) ;
#20089=CIRCLE ( 'NONE', #21938, 1.000000000000000888 ) ;
#20092=CARTESIAN_POINT ( 'NONE',  ( -17.39698466460000148, -18.50000000000000000, 12.78927784919999944 ) ) ;
#20097=FACE_OUTER_BOUND ( 'NONE', #21208, .T. ) ;
#20098=CARTESIAN_POINT ( 'NONE',  ( -10.20110288159999890, -80.50000000000000000, 41.00000000000000000 ) ) ;
#20100=ADVANCED_FACE ( 'NONE', ( #18500 ), #5151, .T. ) ;
#20101=B_SPLINE_SURFACE_WITH_KNOTS ( 'NONE', 5, 5, ( 
 ( #14822, #23726, #2424, #15653, #13471, #25914 ),
 ( #2271, #14959, #11279, #20185, #12489, #3906 ),
 ( #10301, #9099, #15802, #19212, #12772, #3769 ),
 ( #21682, #28101, #12630, #10439, #19357, #28230 ),
 ( #20324, #27043, #11423, #395, #4745, #7087 ),
 ( #13624, #15950, #9244, #18146, #22532, #2574 ) ),
 .UNSPECIFIED., .F., .F., .F.,
 ( 6, 6 ),
 ( 6, 6 ),
 ( 2.788355763089999773, 6.107000906329999701 ),
 ( 0.000000000000000000, 0.5000000000000000000 ),
 .UNSPECIFIED. ) ;
#20105=ORIENTED_EDGE ( 'NONE', *, *, #25738, .F. ) ;
#20107=ORIENTED_EDGE ( 'NONE', *, *, #15749, .F. ) ;
#20108=CARTESIAN_POINT ( 'NONE',  ( -11.45174557200000010, -57.47815920939999756, 20.36405547780000092 ) ) ;
#20110=EDGE_LOOP ( 'NONE', ( #28732, #28528 ) ) ;
#20112=CARTESIAN_POINT ( 'NONE',  ( -3.380646432312965910, -68.17003325777139366, -27.59278602273885994 ) ) ;
#20115=CARTESIAN_POINT ( 'NONE',  ( -35.88566914520000495, -74.50000000000000000, -26.69328098980000163 ) ) ;
#20117=CARTESIAN_POINT ( 'NONE',  ( 21.57540932361363417, -37.72269071045047895, -7.960245178404622202 ) ) ;
#20120=CARTESIAN_POINT ( 'NONE',  ( 40.00000000000000000, -69.00000000000000000, 4.790612351260000516E-15 ) ) ;
#20121=CARTESIAN_POINT ( 'NONE',  ( -13.75178900340000077, -72.82938648530000592, -25.17248092229999656 ) ) ;
#20123=DIRECTION ( 'NONE',  ( 0.000000000000000000, -1.000000000000000000, 0.000000000000000000 ) ) ;
#20125=CARTESIAN_POINT ( 'NONE',  ( 7.700566120479999555, -64.93340739229999770, -23.87431538810000120 ) ) ;
#20126=ORIENTED_EDGE ( 'NONE', *, *, #7421, .T. ) ;
#20127=CARTESIAN_POINT ( 'NONE',  ( 27.43242808539999800, -69.88456486680000523, 1.405611812030000074 ) ) ;
#20128=VECTOR ( 'NONE', #15098, 1000.000000000000000 ) ;
#20130=CARTESIAN_POINT ( 'NONE',  ( 7.362282589679999489, -57.47832521680000184, -22.17287418769999974 ) ) ;
#20131=CARTESIAN_POINT ( 'NONE',  ( 22.18552055780000032, -36.00000000000000000, -11.24205708569999906 ) ) ;
#20132=CARTESIAN_POINT ( 'NONE',  ( -11.77274832230000001, -49.87554870529999818, -19.87235798440000423 ) ) ;
#20135=DIRECTION ( 'NONE',  ( -0.9952295494196654602, 0.000000000000000000, 0.09756097560976760563 ) ) ;
#20136=CARTESIAN_POINT ( 'NONE',  ( -34.11790219230000076, -74.50000000000000000, -24.21840725559999896 ) ) ;
#20138=ADVANCED_FACE ( 'NONE', ( #7591 ), #9555, .T. ) ;
#20142=VECTOR ( 'NONE', #10496, 1000.000000000000000 ) ;
#20145=CARTESIAN_POINT ( 'NONE',  ( 36.29172732829999859, -79.00000000000000000, -14.94947765220000058 ) ) ;
#20147=CARTESIAN_POINT ( 'NONE',  ( 23.74951379730920920, -19.48875272113166446, 1.479235313801489538 ) ) ;
#20149=DIRECTION ( 'NONE',  ( 0.000000000000000000, 1.000000000000000000, 0.000000000000000000 ) ) ;
#20151=CARTESIAN_POINT ( 'NONE',  ( 8.351979489730000594, -36.77152986899999831, -21.41523737049999809 ) ) ;
#20152=CIRCLE ( 'NONE', #9461, 39.75000000000000000 ) ;
#20153=CARTESIAN_POINT ( 'NONE',  ( 9.000933793642678538, -19.49520308528501999, -19.19207797698259910 ) ) ;
#20154=CARTESIAN_POINT ( 'NONE',  ( -23.86485386499999706, -74.50000000000000000, -34.47145558279999733 ) ) ;
#20156=CARTESIAN_POINT ( 'NONE',  ( 2.664535259099999805E-15, -18.50000000000000000, 7.105427357599999217E-15 ) ) ;
#20157=CARTESIAN_POINT ( 'NONE',  ( 10.56351947379999956, -19.46510050329999686, 19.33639269489999890 ) ) ;
#20159=DIRECTION ( 'NONE',  ( 0.000000000000000000, -1.000000000000000000, 0.000000000000000000 ) ) ;
#20160=CARTESIAN_POINT ( 'NONE',  ( -13.18577703620000108, -18.86473241050000027, 19.56302201480000136 ) ) ;
#20162=DIRECTION ( 'NONE',  ( 6.123031769109993025E-17, 0.000000000000000000, -1.000000000000000000 ) ) ;
#20163=B_SPLINE_SURFACE_WITH_KNOTS ( 'NONE', 5, 5, ( 
 ( #23789, #4104, #10224, #19690, #28436, #25844, #10495, #15016, #12549 ),
 ( #16953, #21463, #25975, #8323, #26116, #5866, #1517, #19276, #28162 ),
 ( #5999, #3968, #26267, #10778, #19136, #28025, #15155, #14746, #19410 ),
 ( #3827, #6289, #3554, #14616, #12690, #28581, #21603, #1659, #16809 ),
 ( #28291, #17226, #23930, #12829, #12975, #25704, #11782, #13125, #753 ),
 ( #311, #16008, #16299, #9598, #14126, #20834, #13973, #4253, #2631 ),
 ( #23024, #27245, #5091, #4805, #18497, #2771, #27391, #11626, #7282 ),
 ( #11478, #20384, #3075, #25209, #22588, #5242, #22037, #20693, #7439 ),
 ( #11928, #25057, #22878, #24219, #458, #24913, #8614, #11338, #9151 ) ),
 .UNSPECIFIED., .F., .F., .F.,
 ( 6, 3, 6 ),
 ( 6, 3, 6 ),
 ( 112.4516929440000013, 115.4092999559999981, 122.9563471670000041 ),
 ( 0.000000000000000000, 1.000000000000000000, 2.000000000000000000 ),
 .UNSPECIFIED. ) ;
#20166=CARTESIAN_POINT ( 'NONE',  ( 25.35615114710841311, -58.58931700480601990, 1.380148426380368720 ) ) ;
#20168=LINE ( 'NONE', #241, #20682 ) ;
#20173=AXIS2_PLACEMENT_3D ( 'NONE', #3913, #21686, #5817 ) ;
#20176=CARTESIAN_POINT ( 'NONE',  ( -14.22204520130000027, -64.47177057220000052, 21.80995652580000410 ) ) ;
#20177=CARTESIAN_POINT ( 'NONE',  ( -13.32832959340000123, -60.38621941009999716, 20.74301091450000101 ) ) ;
#20180=FACE_OUTER_BOUND ( 'NONE', #16714, .T. ) ;
#20182=CARTESIAN_POINT ( 'NONE',  ( -11.22677516657805441, -38.85105898695408655, -22.23717618143276198 ) ) ;
#20183=EDGE_LOOP ( 'NONE', ( #6131, #27193, #17892, #26387 ) ) ;
#20185=CARTESIAN_POINT ( 'NONE',  ( -7.323170304809999642, -73.87254094300001839, -39.07240670449999698 ) ) ;
#20188=B_SPLINE_CURVE_WITH_KNOTS ( 'NONE', 5,
 ( #6270, #15135, #21341, #14492, #1263, #26246 ),
 .UNSPECIFIED., .F., .F.,
 ( 6, 6 ),
 ( 0.000000000000000000, 1.000000000000000000 ),
 .UNSPECIFIED. ) ;
#20189=ORIENTED_EDGE ( 'NONE', *, *, #24723, .T. ) ;
#20190=DIRECTION ( 'NONE',  ( 0.6710133869769326909, 0.000000000000000000, 0.7414452336469262717 ) ) ;
#20193=CARTESIAN_POINT ( 'NONE',  ( 20.57577040579999661, -39.36011816900000326, 10.15925981210000018 ) ) ;
#20197=CARTESIAN_POINT ( 'NONE',  ( -14.07499735140000041, -74.00781516410000904, 36.22406682180000104 ) ) ;
#20198=CARTESIAN_POINT ( 'NONE',  ( -32.67688019444538838, -79.98725929158342751, -22.59384834802810360 ) ) ;
#20200=ORIENTED_EDGE ( 'NONE', *, *, #12161, .T. ) ;
#20201=FACE_OUTER_BOUND ( 'NONE', #21761, .T. ) ;
#20204=CYLINDRICAL_SURFACE ( 'NONE', #1590, 7.250000000000004441 ) ;
#20206=VERTEX_POINT ( 'NONE', #11285 ) ;
#20209=ORIENTED_EDGE ( 'NONE', *, *, #12776, .F. ) ;
#20210=DIRECTION ( 'NONE',  ( 1.000000000000000000, 0.000000000000000000, 0.000000000000000000 ) ) ;
#20211=CARTESIAN_POINT ( 'NONE',  ( 24.39713799250000292, -19.50000027030000282, 1.459766484860000046 ) ) ;
#20212=CIRCLE ( 'NONE', #7687, 7.250000000000000000 ) ;
#20216=VECTOR ( 'NONE', #7961, 1000.000000000000000 ) ;
#20217=ORIENTED_EDGE ( 'NONE', *, *, #20031, .F. ) ;
#20220=CARTESIAN_POINT ( 'NONE',  ( 45.84677419350000349, -73.50000000000000000, -4.286925650119999709 ) ) ;
#20221=EDGE_LOOP ( 'NONE', ( #17989, #17551, #25185, #14708 ) ) ;
#20223=CARTESIAN_POINT ( 'NONE',  ( -22.43272078519999724, -80.50000000000000000, -32.20769377289999369 ) ) ;
#20225=CARTESIAN_POINT ( 'NONE',  ( 8.472394962660001028, -37.95144078849999403, -21.79230209929999873 ) ) ;
#20229=ORIENTED_EDGE ( 'NONE', *, *, #21146, .T. ) ;
#20232=FACE_OUTER_BOUND ( 'NONE', #7317, .T. ) ;
#20233=CARTESIAN_POINT ( 'NONE',  ( -40.70731707320000226, -74.50000000000000000, 7.215414233289999757 ) ) ;
#20234=DIRECTION ( 'NONE',  ( 0.000000000000000000, -1.000000000000000000, 0.000000000000000000 ) ) ;
#20239=CARTESIAN_POINT ( 'NONE',  ( -46.75000000000000000, -69.00000000000000000, -8.848045483979999792E-16 ) ) ;
#20244=VECTOR ( 'NONE', #4552, 1000.000000000000000 ) ;
#20245=CARTESIAN_POINT ( 'NONE',  ( 7.521517671639999847, -35.00270081890000284, -21.29432416079999868 ) ) ;
#20248=CARTESIAN_POINT ( 'NONE',  ( 46.97084204269999930, -79.78836619429999644, -2.796096378869999732 ) ) ;
#20251=DIRECTION ( 'NONE',  ( 0.000000000000000000, 1.000000000000000000, 0.000000000000000000 ) ) ;
#20252=ORIENTED_EDGE ( 'NONE', *, *, #364, .F. ) ;
#20256=CARTESIAN_POINT ( 'NONE',  ( -21.62384810780000066, -74.29049705580000307, -32.72083640759999668 ) ) ;
#20258=LINE ( 'NONE', #24484, #15465 ) ;
#20260=DIRECTION ( 'NONE',  ( 0.000000000000000000, 1.000000000000000000, 0.000000000000000000 ) ) ;
#20261=CARTESIAN_POINT ( 'NONE',  ( 25.72873358008812872, -69.52303041555084917, -8.753713131236221301 ) ) ;
#20263=CARTESIAN_POINT ( 'NONE',  ( 21.48482217526310478, -36.89204261257724227, -7.440941901731657815 ) ) ;
#20264=ORIENTED_EDGE ( 'NONE', *, *, #5891, .F. ) ;
#20265=EDGE_CURVE ( 'NONE', #27117, #5430, #19539, .T. ) ;
#20268=B_SPLINE_CURVE_WITH_KNOTS ( 'NONE', 5,
 ( #655, #7335, #16202, #16060, #11682, #3261, #9507, #18410, #27733 ),
 .UNSPECIFIED., .F., .F.,
 ( 6, 3, 6 ),
 ( 0.000000000000000000, 1.376935797170000031, 2.292504252660000130 ),
 .UNSPECIFIED. ) ;
#20273=CARTESIAN_POINT ( 'NONE',  ( -14.65665268890000128, -79.65629807879999191, 36.94583904750000158 ) ) ;
#20278=CARTESIAN_POINT ( 'NONE',  ( 24.24283979073125650, -74.17041889795191878, -30.71041006161582132 ) ) ;
#20279=CARTESIAN_POINT ( 'NONE',  ( 32.97008108400000026, -74.00000037499999905, -20.36016513680000273 ) ) ;
#20280=CARTESIAN_POINT ( 'NONE',  ( 22.93659714569999863, -60.39374587409999862, -9.160202142630000210 ) ) ;
#20282=CARTESIAN_POINT ( 'NONE',  ( -10.42741367090000004, -18.61794786490000320, 18.97192220850000055 ) ) ;
#20287=AXIS2_PLACEMENT_3D ( 'NONE', #13418, #11061, #13123 ) ;
#20288=CARTESIAN_POINT ( 'NONE',  ( 7.367397733560000717, -74.05254684259999465, 39.49475000900000765 ) ) ;
#20289=CARTESIAN_POINT ( 'NONE',  ( -32.77174707999999725, -79.50000000000000000, -21.60034937969999902 ) ) ;
#20291=CARTESIAN_POINT ( 'NONE',  ( 20.14104788939999935, -35.73233869100000248, -9.018304108959998899 ) ) ;
#20293=ORIENTED_EDGE ( 'NONE', *, *, #24623, .F. ) ;
#20294=DIRECTION ( 'NONE',  ( 0.000000000000000000, -1.000000000000000000, 0.000000000000000000 ) ) ;
#20295=CARTESIAN_POINT ( 'NONE',  ( 7.854008167109999938, -37.08875413240000540, -21.51812330200000289 ) ) ;
#20299=B_SPLINE_CURVE_WITH_KNOTS ( 'NONE', 5,
 ( #15562, #19793, #11180, #26362, #10590, #15411, #13378, #19648, #24467 ),
 .UNSPECIFIED., .F., .F.,
 ( 6, 3, 6 ),
 ( 0.000000000000000000, 0.5000000000000000000, 1.000000000000000000 ),
 .UNSPECIFIED. ) ;
#20303=DIRECTION ( 'NONE',  ( 0.7071067811865475727, 0.000000000000000000, -0.7071067811865475727 ) ) ;
#20306=DIRECTION ( 'NONE',  ( 0.1708373792999889895, 0.000000000000000000, 0.9852992387259372764 ) ) ;
#20310=CARTESIAN_POINT ( 'NONE',  ( 0.000000000000000000, -18.50000000000000000, 0.000000000000000000 ) ) ;
#20312=CARTESIAN_POINT ( 'NONE',  ( 36.28164458730000064, -74.50000000000000000, -14.97346873770000109 ) ) ;
#20317=CARTESIAN_POINT ( 'NONE',  ( -13.49470405399999962, -57.43018220239999749, 20.74700755119999585 ) ) ;
#20318=CARTESIAN_POINT ( 'NONE',  ( 19.97576656849999921, -74.00000000000000000, -19.97576656849999921 ) ) ;
#20320=CARTESIAN_POINT ( 'NONE',  ( 21.64960747819999654, -36.72219091790000078, -8.748808738199999269 ) ) ;
#20321=DIRECTION ( 'NONE',  ( -2.784231178940000568E-16, 0.000000000000000000, 1.000000000000000000 ) ) ;
#20324=CARTESIAN_POINT ( 'NONE',  ( -7.248115120159999591, -74.24284936579999794, -40.37845838710000379 ) ) ;
#20325=CARTESIAN_POINT ( 'NONE',  ( 30.43430859973134162, -74.20053182656846502, -24.62761277945777749 ) ) ;
#20335=CARTESIAN_POINT ( 'NONE',  ( -7.224658177536289472, -73.64797963450716622, -39.39373284330162051 ) ) ;
#20337=CARTESIAN_POINT ( 'NONE',  ( 19.02471330030000018, -18.50000000000000000, 9.686045925820002012 ) ) ;
#20340=B_SPLINE_SURFACE_WITH_KNOTS ( 'NONE', 5, 5, ( 
 ( #12861, #17118, #4438, #10528, #28474, #20018 ),
 ( #4143, #28331, #2259, #11105, #6185, #8788 ),
 ( #15057, #26007, #6031, #2124, #23822, #26307 ),
 ( #17416, #13016, #1977, #22076, #17700, #23967 ),
 ( #28618, #19730, #3864, #10959, #26588, #8650 ),
 ( #6630, #17552, #6477, #19588, #26444, #19868 ) ),
 .UNSPECIFIED., .F., .F., .F.,
 ( 6, 6 ),
 ( 6, 6 ),
 ( 0.000000000000000000, 2.292504252660000130 ),
 ( 0.000000000000000000, 1.000000000000000000 ),
 .UNSPECIFIED. ) ;
#20342=ADVANCED_FACE ( 'NONE', ( #20934 ), #22365, .F. ) ;
#20344=CARTESIAN_POINT ( 'NONE',  ( -12.95441099080000136, -72.29970937929999764, -25.32226104859999793 ) ) ;
#20348=CARTESIAN_POINT ( 'NONE',  ( 22.75761901743981142, -61.36591909834531577, -7.240633913292683133 ) ) ;
#20353=ADVANCED_FACE ( 'NONE', ( #10103 ), #3437, .F. ) ;
#20356=VECTOR ( 'NONE', #18130, 1000.000000000000000 ) ;
#20362=FACE_OUTER_BOUND ( 'NONE', #18487, .T. ) ;
#20363=CARTESIAN_POINT ( 'NONE',  ( 19.97576656849999921, -36.00000000000000000, -19.97576656849999921 ) ) ;
#20365=ORIENTED_EDGE ( 'NONE', *, *, #13809, .T. ) ;
#20367=CARTESIAN_POINT ( 'NONE',  ( -22.41677045990000394, -79.93903203729999518, -32.75734019789999962 ) ) ;
#20369=CARTESIAN_POINT ( 'NONE',  ( 9.476129726560001743, -36.00000000000000000, -20.06309461059999677 ) ) ;
#20372=EDGE_LOOP ( 'NONE', ( #9602, #7350, #13141, #18179 ) ) ;
#20375=CARTESIAN_POINT ( 'NONE',  ( -40.70731707320000226, -74.50000000000000000, 7.215414233289999757 ) ) ;
#20376=CARTESIAN_POINT ( 'NONE',  ( -22.21587842519999967, -74.29049705580000307, -32.78062842099999585 ) ) ;
#20378=CIRCLE ( 'NONE', #14783, 38.75000000000000000 ) ;
#20379=CARTESIAN_POINT ( 'NONE',  ( -19.20882542639999713, -32.73217875690000511, 11.71052916729999893 ) ) ;
#20381=CARTESIAN_POINT ( 'NONE',  ( -19.01889177740000036, -19.17414499179999865, 13.97303501010000026 ) ) ;
#20384=CARTESIAN_POINT ( 'NONE',  ( 23.67625467909999770, -63.41849336990000552, 10.62412784700000046 ) ) ;
#20385=CARTESIAN_POINT ( 'NONE',  ( 8.805019338579999300, -34.63244828799999908, -20.36793968349999773 ) ) ;
#20387=DIRECTION ( 'NONE',  ( 1.000000000000000000, 0.000000000000000000, 0.000000000000000000 ) ) ;
#20389=CARTESIAN_POINT ( 'NONE',  ( 46.88136687659999779, -79.93788011300000562, -2.717859463149999488 ) ) ;
#20390=CARTESIAN_POINT ( 'NONE',  ( 10.50000000000000000, -19.00000000000000000, -5.828670879280000091E-16 ) ) ;
#20392=CARTESIAN_POINT ( 'NONE',  ( -13.16836258200000209, -18.50000000000000000, 18.78571244450000322 ) ) ;
#20393=CARTESIAN_POINT ( 'NONE',  ( -11.45927840279999899, -61.83365245859999959, -22.14359330659999969 ) ) ;
#20394=ADVANCED_FACE ( 'NONE', ( #3300 ), #3394, .T. ) ;
#20395=CARTESIAN_POINT ( 'NONE',  ( 26.52608433400000010, -70.67711320560000843, -11.10241135090000064 ) ) ;
#20397=EDGE_CURVE ( 'NONE', #14954, #3210, #13017, .T. ) ;
#20398=ORIENTED_EDGE ( 'NONE', *, *, #2892, .F. ) ;
#20399=CARTESIAN_POINT ( 'NONE',  ( -35.88566914520000495, -74.50000000000000000, -26.69328098980000163 ) ) ;
#20402=CARTESIAN_POINT ( 'NONE',  ( 23.03829042120000281, -52.56313962710000709, 10.32398954119999956 ) ) ;
#20403=CARTESIAN_POINT ( 'NONE',  ( -21.60034937969999902, -74.50000000000000000, -32.77174707999999725 ) ) ;
#20406=CARTESIAN_POINT ( 'NONE',  ( 1.678657213230000024E-14, -74.00000000000000000, 7.838174553849999450E-15 ) ) ;
#20412=CARTESIAN_POINT ( 'NONE',  ( 21.59890840851629079, -37.78281444658050958, -8.035513333422169779 ) ) ;
#20417=CARTESIAN_POINT ( 'NONE',  ( -31.99064106590000023, -74.00000000000000000, -21.95840602359999849 ) ) ;
#20425=CARTESIAN_POINT ( 'NONE',  ( 7.356933064080000584, -36.56811125840000187, -21.47791245320000186 ) ) ;
#20426=DIRECTION ( 'NONE',  ( 1.000000000000000000, 0.000000000000000000, 0.000000000000000000 ) ) ;
#20427=CARTESIAN_POINT ( 'NONE',  ( -14.76448906705501862, -74.23471952222740811, 36.28496449933966517 ) ) ;
#20428=CARTESIAN_POINT ( 'NONE',  ( 26.28708038020000259, -67.57003242129999876, 0.4743469720099999787 ) ) ;
#20430=TOROIDAL_SURFACE ( 'NONE', #26474, 6.750000000000000000, 0.5000000000000000000 ) ;
#20431=CARTESIAN_POINT ( 'NONE',  ( -7.713029007999999465, -80.00000000000000000, 40.75609756099999714 ) ) ;
#20432=AXIS2_PLACEMENT_3D ( 'NONE', #5756, #6024, #15046 ) ;
#20433=EDGE_CURVE ( 'NONE', #10833, #16440, #13982, .T. ) ;
#20436=CARTESIAN_POINT ( 'NONE',  ( 9.926410842420001046, -36.18196426709999969, -21.60058389869999829 ) ) ;
#20438=VECTOR ( 'NONE', #23875, 1000.000000000000000 ) ;
#20441=CARTESIAN_POINT ( 'NONE',  ( 36.47289904669996474, -79.00000000000000000, -14.78463635570000001 ) ) ;
#20444=LINE ( 'NONE', #13880, #9314 ) ;
#20445=CARTESIAN_POINT ( 'NONE',  ( 27.02159208476454566, -72.26331251235005482, -11.39394181573582188 ) ) ;
#20447=CARTESIAN_POINT ( 'NONE',  ( 8.090026142010000143, -37.42980753870000399, -21.59874174039999772 ) ) ;
#20449=ORIENTED_EDGE ( 'NONE', *, *, #27784, .T. ) ;
#20452=CARTESIAN_POINT ( 'NONE',  ( 21.51316594792547576, -36.56981903696397751, -7.049162187537676871 ) ) ;
#20453=CIRCLE ( 'NONE', #6482, 10.50000000000000000 ) ;
#20456=FACE_OUTER_BOUND ( 'NONE', #24799, .T. ) ;
#20458=AXIS2_PLACEMENT_3D ( 'NONE', #16089, #18442, #27328 ) ;
#20459=CIRCLE ( 'NONE', #24165, 2.000000000000000888 ) ;
#20464=DIRECTION ( 'NONE',  ( -0.2414462220490755373, 0.000000000000000000, 0.9704142011833032377 ) ) ;
#20466=CARTESIAN_POINT ( 'NONE',  ( -32.51056936577126066, -80.00000002169532820, -22.64367424041782684 ) ) ;
#20467=CARTESIAN_POINT ( 'NONE',  ( -22.22906643738334154, -79.56075417968409624, -32.83566815571666098 ) ) ;
#20468=EDGE_CURVE ( 'NONE', #1165, #19506, #3740, .T. ) ;
#20469=CARTESIAN_POINT ( 'NONE',  ( -12.07107500047315263, -68.72948970806329783, -25.24773251016443965 ) ) ;
#20470=CARTESIAN_POINT ( 'NONE',  ( -13.89821210610000080, -61.67838661550000268, 21.35051843089999934 ) ) ;
#20471=CARTESIAN_POINT ( 'NONE',  ( 10.50000000000000000, -18.50000000000000000, 0.000000000000000000 ) ) ;
#20472=CARTESIAN_POINT ( 'NONE',  ( 26.30230850345395766, -72.70510570382117521, 11.30503913471621935 ) ) ;
#20473=CARTESIAN_POINT ( 'NONE',  ( 19.35995903480842983, -19.20927481205639964, 10.50154324412826412 ) ) ;
#20478=CARTESIAN_POINT ( 'NONE',  ( -11.03619930328196297, -25.78856419394296040, -21.97741589576630616 ) ) ;
#20480=CARTESIAN_POINT ( 'NONE',  ( 29.13907669020199265, -74.34630382065689957, -26.26003855043551738 ) ) ;
#20482=ORIENTED_EDGE ( 'NONE', *, *, #20397, .T. ) ;
#20487=CARTESIAN_POINT ( 'NONE',  ( -11.90443957499999961, -64.24504445130001784, -23.68393584109999850 ) ) ;
#20488=CARTESIAN_POINT ( 'NONE',  ( -7.198125313996778907, -73.54003775238706453, -39.10791602294204239 ) ) ;
#20489=CARTESIAN_POINT ( 'NONE',  ( 20.22453322670000020, -19.46723765599999822, 9.600718987880000554 ) ) ;
#20490=CARTESIAN_POINT ( 'NONE',  ( -24.63993737860000266, -74.00000000000000000, 17.98210258840000009 ) ) ;
#20493=CARTESIAN_POINT ( 'NONE',  ( -13.13779125880000009, -70.67790319679998845, -24.39064998879999635 ) ) ;
#20497=CARTESIAN_POINT ( 'NONE',  ( -39.04162410960000074, -73.95638562449998687, -7.432628554119999897 ) ) ;
#20498=ORIENTED_EDGE ( 'NONE', *, *, #23244, .T. ) ;
#20504=ADVANCED_FACE ( 'NONE', ( #15177 ), #5172, .F. ) ;
#20510=ORIENTED_EDGE ( 'NONE', *, *, #10054, .F. ) ;
#20513=CARTESIAN_POINT ( 'NONE',  ( 47.15182475600000345, -74.55832059870000705, -1.380511777149999952 ) ) ;
#20515=CIRCLE ( 'NONE', #18184, 7.750000000000000000 ) ;
#20516=CARTESIAN_POINT ( 'NONE',  ( 7.188997797770536380, -73.53996501802382113, -39.06010443590120218 ) ) ;
#20517=CARTESIAN_POINT ( 'NONE',  ( 23.14416696340000001, -57.40875702419999982, 10.37855830930000067 ) ) ;
#20518=VECTOR ( 'NONE', #2189, 1000.000000000000000 ) ;
#20520=VECTOR ( 'NONE', #22693, 1000.000000000000114 ) ;
#20521=CARTESIAN_POINT ( 'NONE',  ( 34.89999999999999858, -82.50000000000000000, 4.273876174839999917E-15 ) ) ;
#20523=CARTESIAN_POINT ( 'NONE',  ( -2.994983700900000212, -67.58705842039999823, -26.99846661069999953 ) ) ;
#20524=CARTESIAN_POINT ( 'NONE',  ( -16.85275212700000225, -72.18744872199999918, 23.44936106520000152 ) ) ;
#20528=CARTESIAN_POINT ( 'NONE',  ( 25.19716909789999804, -60.27227161350000273, 1.367805385619999869 ) ) ;
#20529=CARTESIAN_POINT ( 'NONE',  ( -21.83908241200000333, -74.03505044649999434, -32.25228936610000119 ) ) ;
#20531=CARTESIAN_POINT ( 'NONE',  ( -36.23922253580000330, -74.00000000000000000, -27.04683438039999999 ) ) ;
#20533=DIRECTION ( 'NONE',  ( 0.000000000000000000, -1.000000000000000000, 0.000000000000000000 ) ) ;
#20537=CARTESIAN_POINT ( 'NONE',  ( 7.573069789530000762, -34.86444500489999854, -21.26629628179999898 ) ) ;
#20540=VERTEX_POINT ( 'NONE', #26574 ) ;
#20541=CARTESIAN_POINT ( 'NONE',  ( 47.25000000000000000, -79.00000000000000000, -7.713829575100000215E-13 ) ) ;
#20542=CIRCLE ( 'NONE', #3348, 7.750000000000000000 ) ;
#20548=CARTESIAN_POINT ( 'NONE',  ( -11.25020521769999959, -58.97460807019999862, -21.16435021079999856 ) ) ;
#20549=CARTESIAN_POINT ( 'NONE',  ( 23.74273760109999998, -65.04364753569998925, -8.271557007380000215 ) ) ;
#20552=CARTESIAN_POINT ( 'NONE',  ( 46.74583929422170314, -73.84834818087099961, -2.656434933962762202 ) ) ;
#20555=CARTESIAN_POINT ( 'NONE',  ( -5.679770007689999289, -80.00000000000000000, 46.75000000000000000 ) ) ;
#20559=CARTESIAN_POINT ( 'NONE',  ( -10.97062381167865830, -19.46488312546199850, -19.21093139428075602 ) ) ;
#20560=DIRECTION ( 'NONE',  ( -0.03516156865429562878, -0.000000000000000000, -0.9993816408608722224 ) ) ;
#20564=B_SPLINE_CURVE_WITH_KNOTS ( 'NONE', 3,
 ( #18006, #4751, #18150, #24999 ),
 .UNSPECIFIED., .F., .F.,
 ( 4, 4 ),
 ( 0.000000000000000000, 1.000000000000000000 ),
 .UNSPECIFIED. ) ;
#20565=ORIENTED_EDGE ( 'NONE', *, *, #26618, .F. ) ;
#20569=EDGE_CURVE ( 'NONE', #2204, #11892, #4754, .T. ) ;
#20572=CARTESIAN_POINT ( 'NONE',  ( -5.679770007689999289, -79.50000000000000000, 46.75000000000000000 ) ) ;
#20573=CARTESIAN_POINT ( 'NONE',  ( 19.36781163719999910, -19.46510053389999939, 10.50580276810000058 ) ) ;
#20574=CARTESIAN_POINT ( 'NONE',  ( 7.066909182079999852, -57.47855601759999900, -22.26662627820000040 ) ) ;
#20578=CARTESIAN_POINT ( 'NONE',  ( -19.80233708279999760, -45.95149559400000072, 14.32903646219999949 ) ) ;
#20580=CARTESIAN_POINT ( 'NONE',  ( 22.43277176080000146, -36.00000000000000000, -11.31764183710000005 ) ) ;
#20581=EDGE_CURVE ( 'NONE', #14378, #25468, #24228, .T. ) ;
#20582=CARTESIAN_POINT ( 'NONE',  ( -14.93121066290857080, -74.45417263471367164, 36.29905574722082662 ) ) ;
#20584=CARTESIAN_POINT ( 'NONE',  ( 26.45575263930000176, -65.75576304679998429, 1.499652290349999806 ) ) ;
#20586=ORIENTED_EDGE ( 'NONE', *, *, #22000, .T. ) ;
#20587=B_SPLINE_CURVE_WITH_KNOTS ( 'NONE', 3,
 ( #23175, #7154, #18219, #9162 ),
 .UNSPECIFIED., .F., .F.,
 ( 4, 4 ),
 ( 0.000000000000000000, 1.000000000000000000 ),
 .UNSPECIFIED. ) ;
#20590=CARTESIAN_POINT ( 'NONE',  ( 20.28517606429999987, -35.95611764439999547, -9.102375980000001476 ) ) ;
#20592=ORIENTED_EDGE ( 'NONE', *, *, #14361, .T. ) ;
#20598=CARTESIAN_POINT ( 'NONE',  ( 19.97576656849999921, -35.50000000000000000, -19.97576656849999921 ) ) ;
#20600=CARTESIAN_POINT ( 'NONE',  ( 8.705919335430001738, -36.40841211670000632, -21.16839176649999743 ) ) ;
#20602=ORIENTED_EDGE ( 'NONE', *, *, #12855, .F. ) ;
#20603=CARTESIAN_POINT ( 'NONE',  ( -39.85457864242477655, -73.88534697531770234, 7.248542667680531792 ) ) ;
#20605=CARTESIAN_POINT ( 'NONE',  ( 23.47728460589999955, -18.62107971969999909, 1.886514288650000148 ) ) ;
#20611=AXIS2_PLACEMENT_3D ( 'NONE', #6086, #14694, #14825 ) ;
#20614=ADVANCED_FACE ( 'NONE', ( #4715 ), #6767, .T. ) ;
#20615=FACE_OUTER_BOUND ( 'NONE', #19065, .T. ) ;
#20617=CARTESIAN_POINT ( 'NONE',  ( 21.88571563610000226, -49.10861551290000193, -7.914382952229998658 ) ) ;
#20619=CARTESIAN_POINT ( 'NONE',  ( -40.00441865919010098, -74.28334043021989430, -7.315281843715277788 ) ) ;
#20622=EDGE_CURVE ( 'NONE', #22934, #15684, #5124, .T. ) ;
#20623=CARTESIAN_POINT ( 'NONE',  ( 36.24656953779999924, -74.89763148439999441, -15.05817772819999867 ) ) ;
#20625=CARTESIAN_POINT ( 'NONE',  ( 7.734359568749999525, -19.46510050329999686, -20.63161913629999944 ) ) ;
#20627=CARTESIAN_POINT ( 'NONE',  ( -14.69770337990000009, -66.39466164420001348, 22.32636990160000323 ) ) ;
#20628=CARTESIAN_POINT ( 'NONE',  ( 8.993405562710000467, -35.68342189879999893, -20.12810762659999853 ) ) ;
#20632=AXIS2_PLACEMENT_3D ( 'NONE', #11979, #22940, #16361 ) ;
#20637=CARTESIAN_POINT ( 'NONE',  ( -11.24329055421529766, -40.03422670525277738, -22.26111247093807322 ) ) ;
#20641=ORIENTED_EDGE ( 'NONE', *, *, #10612, .T. ) ;
#20642=CARTESIAN_POINT ( 'NONE',  ( 8.526512829119999691E-15, -89.50000000000000000, -5.107025913280000248E-16 ) ) ;
#20643=DIRECTION ( 'NONE',  ( -0.7414452336469260496, 0.000000000000000000, 0.6710133869769331350 ) ) ;
#20645=AXIS2_PLACEMENT_3D ( 'NONE', #9557, #5191, #11731 ) ;
#20647=CARTESIAN_POINT ( 'NONE',  ( 47.19280574540000117, -74.66665734379999719, -1.149945984370000174 ) ) ;
#20649=CARTESIAN_POINT ( 'NONE',  ( -14.63774944959999935, -74.36723410090000641, 36.92911291229999904 ) ) ;
#20650=CARTESIAN_POINT ( 'NONE',  ( -21.10814673490000004, -64.47177029070000742, 15.24425172959999841 ) ) ;
#20653=CARTESIAN_POINT ( 'NONE',  ( -12.75356989989999867, -71.11103304360000266, -24.81876632530000037 ) ) ;
#20655=DIRECTION ( 'NONE',  ( 0.000000000000000000, -1.000000000000000000, 0.000000000000000000 ) ) ;
#20656=AXIS2_PLACEMENT_3D ( 'NONE', #19128, #28017, #8055 ) ;
#20657=CARTESIAN_POINT ( 'NONE',  ( 7.347638122930000545E-15, -79.00000000000000000, -40.00000000000000000 ) ) ;
#20659=VERTEX_POINT ( 'NONE', #20157 ) ;
#20660=EDGE_CURVE ( 'NONE', #25644, #321, #28416, .T. ) ;
#20662=CARTESIAN_POINT ( 'NONE',  ( 7.215414233289999757, -82.25000000000000000, 40.70731707320000226 ) ) ;
#20664=DIRECTION ( 'NONE',  ( 1.000000000000000000, 0.000000000000000000, 0.000000000000000000 ) ) ;
#20666=ORIENTED_EDGE ( 'NONE', *, *, #6604, .T. ) ;
#20667=ORIENTED_EDGE ( 'NONE', *, *, #28575, .F. ) ;
#20669=CARTESIAN_POINT ( 'NONE',  ( 20.33566493280000032, -36.00000000000000000, -9.885503726129998725 ) ) ;
#20670=CARTESIAN_POINT ( 'NONE',  ( 47.13476942299999450, -74.39425306939999416, -1.308869127139999922 ) ) ;
#20672=CARTESIAN_POINT ( 'NONE',  ( 7.247217007263055955, -73.85166138358573562, -39.79858521572417374 ) ) ;
#20675=EDGE_CURVE ( 'NONE', #8713, #12207, #3717, .T. ) ;
#20676=CARTESIAN_POINT ( 'NONE',  ( -2.472996982579999781, -66.23852357979998828, -26.10313830509999988 ) ) ;
#20679=ADVANCED_FACE ( 'NONE', ( #18712 ), #27956, .T. ) ;
#20680=CARTESIAN_POINT ( 'NONE',  ( 27.02683049547185234, -18.50000000000000000, 2.817888817433861881 ) ) ;
#20682=VECTOR ( 'NONE', #15186, 1000.000000000000000 ) ;
#20684=CARTESIAN_POINT ( 'NONE',  ( -22.00249031550000112, -74.43208506860000284, -32.67527180340000825 ) ) ;
#20688=DIRECTION ( 'NONE',  ( 0.000000000000000000, 1.000000000000000000, 0.000000000000000000 ) ) ;
#20693=CARTESIAN_POINT ( 'NONE',  ( 21.83772201000000024, -64.02328494229999478, 11.48627575220000097 ) ) ;
#20696=DIRECTION ( 'NONE',  ( 0.000000000000000000, -1.000000000000000000, 0.000000000000000000 ) ) ;
#20698=CARTESIAN_POINT ( 'NONE',  ( 22.89432163829999922, -45.92926717529999792, 10.24748840149999829 ) ) ;
#20701=CARTESIAN_POINT ( 'NONE',  ( -11.70763318529999886, -59.02987586149999544, -20.35466320700000153 ) ) ;
#20707=CARTESIAN_POINT ( 'NONE',  ( 46.73034331009336739, -73.83477249655828700, -2.695375482873064943 ) ) ;
#20709=TOROIDAL_SURFACE ( 'NONE', #9520, 38.75000000000000000, 0.5000000000000000000 ) ;
#20710=CARTESIAN_POINT ( 'NONE',  ( 23.06458040940000132, -53.77454410920000072, 10.33795933400000067 ) ) ;
#20714=CARTESIAN_POINT ( 'NONE',  ( -2.583988331150000040, -57.40875702419999982, -25.23271569440000306 ) ) ;
#20715=CARTESIAN_POINT ( 'NONE',  ( 21.21808891099999883, -34.59820414320000026, -7.670974023059999425 ) ) ;
#20717=DIRECTION ( 'NONE',  ( -0.3687499999999802047, 0.000000000000000000, 0.9295286103719532234 ) ) ;
#20718=DIRECTION ( 'NONE',  ( 0.9828852004421827493, 0.06995790998171046160, -0.1704188181590321205 ) ) ;
#20720=CARTESIAN_POINT ( 'NONE',  ( 46.70302539038219436, -79.89150110136301919, -3.470455026150449651 ) ) ;
#20721=ORIENTED_EDGE ( 'NONE', *, *, #6399, .F. ) ;
#20722=CARTESIAN_POINT ( 'NONE',  ( -32.36019060869999464, -80.06168530479999390, -22.53893507739999791 ) ) ;
#20724=CARTESIAN_POINT ( 'NONE',  ( -20.20157662561761214, -60.34340089795642115, 12.31263473384953322 ) ) ;
#20726=ORIENTED_EDGE ( 'NONE', *, *, #17999, .T. ) ;
#20728=DIRECTION ( 'NONE',  ( 0.000000000000000000, -1.000000000000000000, 0.000000000000000000 ) ) ;
#20730=CARTESIAN_POINT ( 'NONE',  ( 2.842170943039999687E-14, -72.00000000000000000, 1.776356839399999804E-15 ) ) ;
#20732=CARTESIAN_POINT ( 'NONE',  ( 37.05123091498987264, -80.05388659141317476, -13.65971926633490163 ) ) ;
#20734=CARTESIAN_POINT ( 'NONE',  ( -19.06307702970000051, -26.06274386020000122, 13.87368263639999988 ) ) ;
#20735=DIRECTION ( 'NONE',  ( 1.000000000000000000, 0.000000000000000000, 9.436895709309994757E-16 ) ) ;
#20736=CARTESIAN_POINT ( 'NONE',  ( -8.256726973129998370, -80.00000000000000000, 39.42856679209999982 ) ) ;
#20737=CARTESIAN_POINT ( 'NONE',  ( 23.23309277569999765, -57.41957472270000551, -9.464544134220000515 ) ) ;
#20738=CARTESIAN_POINT ( 'NONE',  ( 26.84354920890000074, -67.87586094739999965, 1.442210595809999996 ) ) ;
#20741=CARTESIAN_POINT ( 'NONE',  ( 20.46633117200000029, -56.50943265579999775, 11.19343934389999973 ) ) ;
#20742=CARTESIAN_POINT ( 'NONE',  ( -38.90877162625164232, -73.50999119021167871, -7.168130346706902856 ) ) ;
#20744=EDGE_CURVE ( 'NONE', #6032, #26457, #11183, .T. ) ;
#20746=ORIENTED_EDGE ( 'NONE', *, *, #8960, .T. ) ;
#20747=CARTESIAN_POINT ( 'NONE',  ( -11.16118678780000018, -80.00000000000000000, 46.75000000000000000 ) ) ;
#20749=CARTESIAN_POINT ( 'NONE',  ( -18.67939945255520229, -18.95847994161255912, 11.45706375696013524 ) ) ;
#20753=DIRECTION ( 'NONE',  ( 0.000000000000000000, 1.000000000000000000, 0.000000000000000000 ) ) ;
#20754=ORIENTED_EDGE ( 'NONE', *, *, #1923, .F. ) ;
#20757=CARTESIAN_POINT ( 'NONE',  ( -12.53622301170538123, -19.47630496351773033, 19.30239230919325166 ) ) ;
#20759=VERTEX_POINT ( 'NONE', #26104 ) ;
#20760=CARTESIAN_POINT ( 'NONE',  ( -2.295868756434714442, -19.47636826821743483, -22.90451916462247439 ) ) ;
#20762=CARTESIAN_POINT ( 'NONE',  ( -2.508141046650000039, -45.95149559400000072, -24.31384519909999753 ) ) ;
#20766=DIRECTION ( 'NONE',  ( 0.3687499999999825917, 0.000000000000000000, -0.9295286103719523352 ) ) ;
#20767=CARTESIAN_POINT ( 'NONE',  ( 22.46437391599999955, -49.07760086100000052, -9.030336851770002227 ) ) ;
#20769=FACE_OUTER_BOUND ( 'NONE', #23301, .T. ) ;
#20775=CARTESIAN_POINT ( 'NONE',  ( -14.52637129600000065, -65.75479088560000207, 22.16126353170000129 ) ) ;
#20776=CARTESIAN_POINT ( 'NONE',  ( 8.363364595560000225, -35.90622649329999660, -21.15739189799999664 ) ) ;
#20777=CARTESIAN_POINT ( 'NONE',  ( 7.248796347620719338, -73.89318255930692203, 39.86740956980206363 ) ) ;
#20778=CARTESIAN_POINT ( 'NONE',  ( 2.042810365310000056E-12, -74.50000000000000000, -2.458477865729999957E-12 ) ) ;
#20790=EDGE_CURVE ( 'NONE', #13129, #17905, #25607, .T. ) ;
#20792=DIRECTION ( 'NONE',  ( 0.000000000000000000, 1.000000000000000000, 0.000000000000000000 ) ) ;
#20793=CARTESIAN_POINT ( 'NONE',  ( -7.400691967549999362, -74.17650256410000509, 39.62483793549999689 ) ) ;
#20795=CARTESIAN_POINT ( 'NONE',  ( -7.219194746715977828, -73.62392792452344281, -39.33235237970639986 ) ) ;
#20796=CARTESIAN_POINT ( 'NONE',  ( 1.065814103639999922E-14, -19.50000000000000000, 2.664535259099999805E-15 ) ) ;
#20798=ORIENTED_EDGE ( 'NONE', *, *, #25700, .T. ) ;
#20801=CARTESIAN_POINT ( 'NONE',  ( -21.87551306609999813, -79.25000000000000000, -33.18922156509999866 ) ) ;
#20802=DIRECTION ( 'NONE',  ( 0.1770468907230372535, 0.000000000000000000, 0.9842024174352067556 ) ) ;
#20806=CARTESIAN_POINT ( 'NONE',  ( -0.5413073883429999622, -57.47855574479999774, -23.35488927860000175 ) ) ;
#20809=VERTEX_POINT ( 'NONE', #20121 ) ;
#20811=CARTESIAN_POINT ( 'NONE',  ( 20.82958082409999889, -36.06003250059999488, -9.510880482430000171 ) ) ;
#20813=CARTESIAN_POINT ( 'NONE',  ( 7.246819345882899555, -74.12723354427720324, -40.21639064511597184 ) ) ;
#20814=CARTESIAN_POINT ( 'NONE',  ( -11.45050398651610735, -61.30079904130542445, 20.94026329283510535 ) ) ;
#20815=EDGE_CURVE ( 'NONE', #18945, #16909, #9954, .T. ) ;
#20818=CARTESIAN_POINT ( 'NONE',  ( -3.203052480429999793, -67.37930764479999368, -27.34961382279999853 ) ) ;
#20819=CARTESIAN_POINT ( 'NONE',  ( -15.22881500629999962, -71.94538141299999268, 23.83405028770000200 ) ) ;
#20823=CARTESIAN_POINT ( 'NONE',  ( 23.95396754599999767, -58.97460807019999862, 0.8392115891270000017 ) ) ;
#20824=CARTESIAN_POINT ( 'NONE',  ( -21.35786030099999877, -65.07443093669999712, 13.27975315080000129 ) ) ;
#20825=VERTEX_POINT ( 'NONE', #4528 ) ;
#20829=CARTESIAN_POINT ( 'NONE',  ( -2.619606448679999922, -19.18584080579999807, -24.29997799329999708 ) ) ;
#20830=CARTESIAN_POINT ( 'NONE',  ( 36.43448083739620813, -74.04079074338399380, -14.03271623279055724 ) ) ;
#20834=CARTESIAN_POINT ( 'NONE',  ( 21.58303642010000090, -61.82150526550000080, 10.78270930949999951 ) ) ;
#20835=AXIS2_PLACEMENT_3D ( 'NONE', #23229, #16078, #16374 ) ;
#20836=CARTESIAN_POINT ( 'NONE',  ( 7.472179712070000868, -35.14393334239999689, -21.32187190240000163 ) ) ;
#20839=ORIENTED_EDGE ( 'NONE', *, *, #26923, .F. ) ;
#20840=B_SPLINE_SURFACE_WITH_KNOTS ( 'NONE', 5, 5, ( 
 ( #16584, #7274, #5512, #2910, #597, #1035, #7424, #5231, #22721 ),
 ( #25202, #16141, #25045, #18921, #5078, #12056, #9873, #9590, #3334 ),
 ( #12198, #7579, #18787, #9441, #14116, #23015, #16725, #21113, #25621 ),
 ( #7717, #20528, #1168, #13965, #27381, #10007, #22869, #27801, #11772 ),
 ( #25478, #745, #18640, #5377, #20823, #3065, #11920, #885, #27536 ),
 ( #16443, #14260, #23153, #25758, #23435, #5786, #12463, #25891, #19334 ) ),
 .UNSPECIFIED., .F., .F., .F.,
 ( 6, 6 ),
 ( 6, 3, 6 ),
 ( 8.242378609670000245, 18.74558921149999691 ),
 ( 0.000000000000000000, 1.000000000000000000, 2.000000000000000000 ),
 .UNSPECIFIED. ) ;
#20841=CARTESIAN_POINT ( 'NONE',  ( -10.97235754340000113, -18.50000000000000000, 18.39710783539999994 ) ) ;
#20843=CARTESIAN_POINT ( 'NONE',  ( 24.98429922149999882, -68.01082593649999808, -9.444232459920000267 ) ) ;
#20845=VECTOR ( 'NONE', #15846, 1000.000000000000000 ) ;
#20847=EDGE_CURVE ( 'NONE', #23425, #28710, #12143, .T. ) ;
#20850=CYLINDRICAL_SURFACE ( 'NONE', #11863, 7.249999999999999112 ) ;
#20851=ORIENTED_EDGE ( 'NONE', *, *, #23539, .T. ) ;
#20852=CARTESIAN_POINT ( 'NONE',  ( -13.52482488829999951, -26.99661847659999836, 20.57476094929999633 ) ) ;
#20855=EDGE_CURVE ( 'NONE', #20206, #300, #15864, .T. ) ;
#20857=CARTESIAN_POINT ( 'NONE',  ( 39.49501612680000306, -74.05258142290000478, 7.367357169019999930 ) ) ;
#20858=CARTESIAN_POINT ( 'NONE',  ( -10.48421507011602927, -19.48210984065671880, -20.91038783075365970 ) ) ;
#20859=DIRECTION ( 'NONE',  ( 0.000000000000000000, -1.000000000000000000, 0.000000000000000000 ) ) ;
#20861=CARTESIAN_POINT ( 'NONE',  ( 9.917934831007896079, -63.16257045312386964, -24.43292808095910118 ) ) ;
#20863=CARTESIAN_POINT ( 'NONE',  ( -32.69645379630000548, -79.50000000000000000, -21.71458329359999695 ) ) ;
#20864=CARTESIAN_POINT ( 'NONE',  ( -36.23922253580000330, -79.50000000000000000, -26.33972759919999973 ) ) ;
#20867=ORIENTED_EDGE ( 'NONE', *, *, #10927, .T. ) ;
#20868=CARTESIAN_POINT ( 'NONE',  ( -3.807886452449999570, -79.99999996820000092, 46.75000006680000553 ) ) ;
#20875=CARTESIAN_POINT ( 'NONE',  ( -19.24564007919999753, -39.36582103120000653, 12.09558240470000179 ) ) ;
#20877=CARTESIAN_POINT ( 'NONE',  ( 28.91021413440000032, -73.86467020649999426, -26.59947370389999932 ) ) ;
#20878=CARTESIAN_POINT ( 'NONE',  ( 22.33353861309999999, -57.45905989829999783, -8.600015579559999068 ) ) ;
#20879=CARTESIAN_POINT ( 'NONE',  ( 25.73809814099999826, -66.36684605059998887, -0.2162503729670000041 ) ) ;
#20880=CARTESIAN_POINT ( 'NONE',  ( -10.60992277839999964, -18.50000000000000000, 18.52090900019999964 ) ) ;
#20881=ADVANCED_FACE ( 'NONE', ( #206 ), #28742, .T. ) ;
#20884=ORIENTED_EDGE ( 'NONE', *, *, #7763, .T. ) ;
#20885=ADVANCED_FACE ( 'NONE', ( #12236 ), #9625, .F. ) ;
#20886=CARTESIAN_POINT ( 'NONE',  ( -39.68146194298503815, -73.78481856947901463, -7.243236069910341968 ) ) ;
#20887=CARTESIAN_POINT ( 'NONE',  ( 21.69038160389999703, -37.92210000699999739, -8.278728714260001453 ) ) ;
#20888=ORIENTED_EDGE ( 'NONE', *, *, #22890, .F. ) ;
#20889=CARTESIAN_POINT ( 'NONE',  ( 40.70731707320000226, -80.50000000000000000, -7.215414233289999757 ) ) ;
#20892=CARTESIAN_POINT ( 'NONE',  ( -17.13033212710000086, -72.00000000000000000, 23.49748962700000021 ) ) ;
#20900=CARTESIAN_POINT ( 'NONE',  ( -27.04683438039999999, -74.00000000000000000, -36.23922253580000330 ) ) ;
#20902=CARTESIAN_POINT ( 'NONE',  ( -2.631833427070000120, -26.03958238299999906, -24.12317078430000095 ) ) ;
#20905=CARTESIAN_POINT ( 'NONE',  ( 11.31764174110000098, -36.00000000000000000, -22.43277175240000076 ) ) ;
#20906=EDGE_CURVE ( 'NONE', #17644, #16909, #2380, .T. ) ;
#20908=CARTESIAN_POINT ( 'NONE',  ( 21.99751943120000064, -53.29445792020000283, -7.633405283620000148 ) ) ;
#20910=CARTESIAN_POINT ( 'NONE',  ( -13.66168260340000096, -72.00000000000000000, -27.27344781959999764 ) ) ;
#20911=ORIENTED_EDGE ( 'NONE', *, *, #16811, .F. ) ;
#20913=VECTOR ( 'NONE', #17355, 1000.000000000000000 ) ;
#20916=AXIS2_PLACEMENT_3D ( 'NONE', #21906, #3985, #6450 ) ;
#20918=CARTESIAN_POINT ( 'NONE',  ( 21.23424069599999697, -35.30313414209999934, -7.936589188299999265 ) ) ;
#20919=CARTESIAN_POINT ( 'NONE',  ( 23.34294251050530988, -60.17793182509785055, 10.47223221149565653 ) ) ;
#20924=VERTEX_POINT ( 'NONE', #14296 ) ;
#20926=CARTESIAN_POINT ( 'NONE',  ( 30.67749406165812687, -74.17397605894404933, -24.28944146970528450 ) ) ;
#20927=DIRECTION ( 'NONE',  ( 0.7071067811865475727, 0.000000000000000000, -0.7071067811865475727 ) ) ;
#20928=VERTEX_POINT ( 'NONE', #14435 ) ;
#20929=DIRECTION ( 'NONE',  ( 0.000000000000000000, -1.000000000000000000, 0.000000000000000000 ) ) ;
#20934=FACE_OUTER_BOUND ( 'NONE', #21166, .T. ) ;
#20935=CARTESIAN_POINT ( 'NONE',  ( -10.17458377400000025, -18.50000000000000000, -22.50859265919999785 ) ) ;
#20936=CARTESIAN_POINT ( 'NONE',  ( 21.93840406509999852, -73.88712764410000489, -31.96455063700000210 ) ) ;
#20937=LINE ( 'NONE', #23121, #9005 ) ;
#20940=CARTESIAN_POINT ( 'NONE',  ( -11.93607363350000128, -70.93453115479999838, -26.12370071229999979 ) ) ;
#20941=CARTESIAN_POINT ( 'NONE',  ( 8.807493968779999349, -25.53205038710000352, -20.04401236839999711 ) ) ;
#20942=CARTESIAN_POINT ( 'NONE',  ( -2.353367408830994378, -57.44036977208730121, -24.34032937392296603 ) ) ;
#20943=CARTESIAN_POINT ( 'NONE',  ( 7.990241584909999695, -34.99644672609999674, -21.18700924519999873 ) ) ;
#20944=EDGE_LOOP ( 'NONE', ( #12911, #19244, #11117, #1842 ) ) ;
#20949=ADVANCED_FACE ( 'NONE', ( #3238 ), #5126, .T. ) ;
#20950=TOROIDAL_SURFACE ( 'NONE', #20458, 7.750000000000000000, 0.5000000000000000000 ) ;
#20951=CARTESIAN_POINT ( 'NONE',  ( -2.565531208409999930, -57.41946943429999806, -24.92671054230000038 ) ) ;
#20952=B_SPLINE_CURVE_WITH_KNOTS ( 'NONE', 5,
 ( #5846, #26247, #1641, #23909, #3947, #12810 ),
 .UNSPECIFIED., .F., .F.,
 ( 6, 6 ),
 ( 0.000000000000000000, 1.000000000000000000 ),
 .UNSPECIFIED. ) ;
#20955=DIRECTION ( 'NONE',  ( 0.9704142011833034598, 0.000000000000000000, 0.2414462220490750377 ) ) ;
#20957=CARTESIAN_POINT ( 'NONE',  ( -20.18078161143439786, -39.33785704641559278, 14.62338064274810634 ) ) ;
#20959=CARTESIAN_POINT ( 'NONE',  ( 22.08525036290000187, -37.96517279220000063, -8.883154216930000402 ) ) ;
#20962=CARTESIAN_POINT ( 'NONE',  ( 7.198781031971043021, -73.55869875168694705, -39.13694367198868918 ) ) ;
#20964=ORIENTED_EDGE ( 'NONE', *, *, #18509, .F. ) ;
#20965=CARTESIAN_POINT ( 'NONE',  ( -14.43245924010000003, -80.10005509740000207, 36.56795405499999418 ) ) ;
#20966=CARTESIAN_POINT ( 'NONE',  ( -3.669439427430000400, -72.55114739969998539, -28.40640588289999968 ) ) ;
#20967=CARTESIAN_POINT ( 'NONE',  ( -16.03641129780000085, -70.40840182630000754, 23.20817888690000075 ) ) ;
#20968=VERTEX_POINT ( 'NONE', #9483 ) ;
#20969=CIRCLE ( 'NONE', #24679, 6.750000000000000000 ) ;
#20972=CARTESIAN_POINT ( 'NONE',  ( -20.21023039549999822, -62.10525983699999841, 13.01158141169999993 ) ) ;
#20973=ORIENTED_EDGE ( 'NONE', *, *, #10612, .F. ) ;
#20974=CYLINDRICAL_SURFACE ( 'NONE', #13879, 3.749999999999996447 ) ;
#20975=CARTESIAN_POINT ( 'NONE',  ( -7.292785445180875570, -73.99991600666669456, 39.60658383038346386 ) ) ;
#20976=CARTESIAN_POINT ( 'NONE',  ( 36.44118056271604189, -74.04359402117586342, -14.04216929337327713 ) ) ;
#20984=CARTESIAN_POINT ( 'NONE',  ( 36.94915360298272589, -79.79696885169119014, -14.35475846226867702 ) ) ;
#20985=AXIS2_PLACEMENT_3D ( 'NONE', #27106, #15564, #24772 ) ;
#20986=CARTESIAN_POINT ( 'NONE',  ( 25.01891871080000129, -68.13686112700000308, -8.889018148439999933 ) ) ;
#20989=VERTEX_POINT ( 'NONE', #16332 ) ;
#20990=VECTOR ( 'NONE', #16594, 1000.000000000000000 ) ;
#20992=ORIENTED_EDGE ( 'NONE', *, *, #10543, .F. ) ;
#20993=DIRECTION ( 'NONE',  ( 0.000000000000000000, -1.000000000000000000, 0.000000000000000000 ) ) ;
#20995=ORIENTED_EDGE ( 'NONE', *, *, #4825, .F. ) ;
#20996=DIRECTION ( 'NONE',  ( 0.000000000000000000, 0.000000000000000000, -1.000000000000000000 ) ) ;
#20997=CARTESIAN_POINT ( 'NONE',  ( 40.70731707320000226, -74.50000000000000000, 7.215414233289999757 ) ) ;
#20998=CARTESIAN_POINT ( 'NONE',  ( -11.17610348543527010, -19.46454334095421146, -19.00959556865977262 ) ) ;
#20999=DIRECTION ( 'NONE',  ( 0.06892947544783696590, -0.9975499440283633890, -0.01195142600257996686 ) ) ;
#21001=CARTESIAN_POINT ( 'NONE',  ( 9.564509902230000193, -57.40875702419999982, -23.52622212079999997 ) ) ;
#21003=CARTESIAN_POINT ( 'NONE',  ( -2.664535259099999805E-15, -72.82938648530000592, -3.552713678799999608E-15 ) ) ;
#21004=CARTESIAN_POINT ( 'NONE',  ( 7.670973119660000172, -34.59820496239999699, -21.21808926809999818 ) ) ;
#21005=FACE_OUTER_BOUND ( 'NONE', #23021, .T. ) ;
#21006=DIRECTION ( 'NONE',  ( 0.000000000000000000, -1.000000000000000000, 0.000000000000000000 ) ) ;
#21007=EDGE_LOOP ( 'NONE', ( #24025, #26050, #21759, #3538 ) ) ;
#21009=AXIS2_PLACEMENT_3D ( 'NONE', #8603, #8311, #23773 ) ;
#21010=CARTESIAN_POINT ( 'NONE',  ( -0.7196032852779999933, -79.77560502979999058, 47.25024237019999873 ) ) ;
#21011=CARTESIAN_POINT ( 'NONE',  ( -15.42363691649999957, -67.46051717960000360, 22.84488648889999851 ) ) ;
#21012=VERTEX_POINT ( 'NONE', #20647 ) ;
#21013=AXIS2_PLACEMENT_3D ( 'NONE', #23136, #9281, #12044 ) ;
#21014=EDGE_CURVE ( 'NONE', #17168, #28456, #20515, .T. ) ;
#21017=CARTESIAN_POINT ( 'NONE',  ( -19.20879816019999708, -32.73130089779999707, 11.71051500439999948 ) ) ;
#21018=CARTESIAN_POINT ( 'NONE',  ( -33.25000000000000000, -69.50000000000000000, 5.481726184089999968E-15 ) ) ;
#21019=CARTESIAN_POINT ( 'NONE',  ( 29.02377468160000262, -74.30612813009999229, -26.48574803420000023 ) ) ;
#21021=CARTESIAN_POINT ( 'NONE',  ( -13.44405788329999929, -68.28990366489999531, 22.97003105929999833 ) ) ;
#21022=EDGE_CURVE ( 'NONE', #3611, #25958, #14155, .T. ) ;
#21023=CARTESIAN_POINT ( 'NONE',  ( 26.87922219139999669, -65.53745956530001138, 1.653266478199999945 ) ) ;
#21024=CARTESIAN_POINT ( 'NONE',  ( -10.80821428159999975, -18.85485912780000106, 19.04257197200000107 ) ) ;
#21027=CARTESIAN_POINT ( 'NONE',  ( 8.721287999440001215, -37.33944922460000271, -21.87060590859999820 ) ) ;
#21029=CARTESIAN_POINT ( 'NONE',  ( 19.96641028149999997, -35.92495628129999830, -9.198931196760000262 ) ) ;
#21031=ORIENTED_EDGE ( 'NONE', *, *, #19239, .T. ) ;
#21032=CARTESIAN_POINT ( 'NONE',  ( -11.05730518689999897, -18.50000000000000000, -18.25363368680000065 ) ) ;
#21033=DIRECTION ( 'NONE',  ( 1.000000000000000000, 0.000000000000000000, 0.000000000000000000 ) ) ;
#21034=AXIS2_PLACEMENT_3D ( 'NONE', #8103, #23418, #6043 ) ;
#21036=CARTESIAN_POINT ( 'NONE',  ( -15.42363691649999957, -67.46051717960000360, 22.84488648889999851 ) ) ;
#21037=DIRECTION ( 'NONE',  ( 1.000000000000000000, 0.000000000000000000, 0.000000000000000000 ) ) ;
#21041=CARTESIAN_POINT ( 'NONE',  ( -39.89765284886984631, -73.91187068862662102, 7.249313954218240319 ) ) ;
#21045=CARTESIAN_POINT ( 'NONE',  ( 18.93437244589999935, -18.87168146930000034, -8.901252599150000222 ) ) ;
#21047=CARTESIAN_POINT ( 'NONE',  ( 19.97576656849999921, -19.50000000000000000, -19.97576656849999921 ) ) ;
#21050=CARTESIAN_POINT ( 'NONE',  ( -2.481178842626576841, -74.00000000000000000, 46.81450634432220426 ) ) ;
#21056=VERTEX_POINT ( 'NONE', #13480 ) ;
#21057=CARTESIAN_POINT ( 'NONE',  ( -32.81694319320000375, -74.37394555080000202, -22.22457704239999998 ) ) ;
#21061=FACE_OUTER_BOUND ( 'NONE', #15067, .T. ) ;
#21062=CARTESIAN_POINT ( 'NONE',  ( 7.248542667680995422, -73.88534697533242479, 39.85457864244732917 ) ) ;
#21064=FACE_OUTER_BOUND ( 'NONE', #14691, .T. ) ;
#21066=AXIS2_PLACEMENT_3D ( 'NONE', #20642, #25309, #6940 ) ;
#21068=FACE_OUTER_BOUND ( 'NONE', #28028, .T. ) ;
#21071=CARTESIAN_POINT ( 'NONE',  ( -32.25000000000000000, -73.50000000000000000, 2.464695114664749979E-15 ) ) ;
#21073=CARTESIAN_POINT ( 'NONE',  ( 7.215414233289999757, -74.50000000000000000, -40.70731707320000226 ) ) ;
#21075=CARTESIAN_POINT ( 'NONE',  ( -11.72000839801819616, -19.46749782351740876, 19.06227229943159429 ) ) ;
#21076=CARTESIAN_POINT ( 'NONE',  ( -7.280256974170000284, -74.15866376920000391, 39.93430878389999350 ) ) ;
#21078=CARTESIAN_POINT ( 'NONE',  ( 3.768036230260000150E-15, -69.50000000000000000, 40.00000000000000000 ) ) ;
#21081=ADVANCED_FACE ( 'NONE', ( #10388 ), #14317, .T. ) ;
#21082=CARTESIAN_POINT ( 'NONE',  ( 10.69287703170000015, -70.89709150720000252, -26.27243468539999682 ) ) ;
#21084=B_SPLINE_SURFACE_WITH_KNOTS ( 'NONE', 5, 5, ( 
 ( #14469, #12536, #17071, #21045, #27868, #28015 ),
 ( #27611, #16652, #8185, #23775, #3817, #9804 ),
 ( #21453, #23363, #19125, #18714, #21311, #5584 ),
 ( #7651, #19263, #1102, #3405, #10350, #16519 ),
 ( #9943, #25693, #1509, #25414, #5718, #1364 ),
 ( #5446, #14330, #23224, #18858, #14737, #14602 ) ),
 .UNSPECIFIED., .F., .F., .F.,
 ( 6, 6 ),
 ( 6, 6 ),
 ( 0.000000000000000000, 2.292501860869999852 ),
 ( 0.000000000000000000, 1.000000000000000000 ),
 .UNSPECIFIED. ) ;
#21091=AXIS2_PLACEMENT_3D ( 'NONE', #1587, #27952, #10426 ) ;
#21095=DIRECTION ( 'NONE',  ( 0.000000000000000000, 1.000000000000000000, 0.000000000000000000 ) ) ;
#21096=DIRECTION ( 'NONE',  ( 1.110223024630000146E-15, 0.000000000000000000, -1.000000000000000000 ) ) ;
#21098=ORIENTED_EDGE ( 'NONE', *, *, #23358, .T. ) ;
#21101=FACE_OUTER_BOUND ( 'NONE', #14780, .T. ) ;
#21103=FACE_OUTER_BOUND ( 'NONE', #28056, .T. ) ;
#21104=ORIENTED_EDGE ( 'NONE', *, *, #14240, .T. ) ;
#21106=CARTESIAN_POINT ( 'NONE',  ( 8.189694586359999917, -36.39795110199999328, -21.29668027459999990 ) ) ;
#21107=CARTESIAN_POINT ( 'NONE',  ( -14.59815773839999942, -79.49999996000001090, 36.63377407710000000 ) ) ;
#21108=EDGE_CURVE ( 'NONE', #17563, #2951, #8420, .T. ) ;
#21109=AXIS2_PLACEMENT_3D ( 'NONE', #5675, #28378, #6234 ) ;
#21111=ORIENTED_EDGE ( 'NONE', *, *, #13073, .F. ) ;
#21113=CARTESIAN_POINT ( 'NONE',  ( 23.98000230750000128, -62.12717499380000419, -0.2704306557409999479 ) ) ;
#21114=CARTESIAN_POINT ( 'NONE',  ( -20.17414664320000028, -60.59603168650000526, 12.28933892000000050 ) ) ;
#21115=EDGE_LOOP ( 'NONE', ( #2446, #24120, #24298, #25875, #4802, #24476, #6964 ) ) ;
#21116=CARTESIAN_POINT ( 'NONE',  ( 23.74273760109999998, -65.04364753569998925, -8.271557007380000215 ) ) ;
#21117=CARTESIAN_POINT ( 'NONE',  ( -1.803985702539999902, -19.15979404320000157, -22.30692425470000373 ) ) ;
#21122=CARTESIAN_POINT ( 'NONE',  ( 36.78261483260000375, -79.80697408650000568, -14.39505880960000006 ) ) ;
#21124=ORIENTED_EDGE ( 'NONE', *, *, #8663, .F. ) ;
#21125=UNCERTAINTY_MEASURE_WITH_UNIT (LENGTH_MEASURE( 1.000000000000000082E-05 ), #27847, 'distance_accuracy_value', 'NONE');
#21126=FACE_OUTER_BOUND ( 'NONE', #14808, .T. ) ;
#21131=ORIENTED_EDGE ( 'NONE', *, *, #2045, .T. ) ;
#21132=CARTESIAN_POINT ( 'NONE',  ( -12.50408296909999883, -42.25464550570000455, 19.83474686469999781 ) ) ;
#21134=ORIENTED_EDGE ( 'NONE', *, *, #23513, .F. ) ;
#21136=CARTESIAN_POINT ( 'NONE',  ( 9.726843560609999884, -36.00000000000000000, -20.21912206349999863 ) ) ;
#21137=ADVANCED_FACE ( 'NONE', ( #1970 ), #86, .T. ) ;
#21139=CIRCLE ( 'NONE', #8100, 13.00000000000000178 ) ;
#21140=CARTESIAN_POINT ( 'NONE',  ( 38.70548920639999579, -73.81415963839999961, 7.196176986149999344 ) ) ;
#21143=CARTESIAN_POINT ( 'NONE',  ( 19.94173275869999884, -39.36577621580000397, 10.90498865049999822 ) ) ;
#21144=CARTESIAN_POINT ( 'NONE',  ( 47.07870869154496063, -79.56040629918834384, -1.981086625768881060 ) ) ;
#21146=EDGE_CURVE ( 'NONE', #24982, #13659, #23327, .T. ) ;
#21147=CARTESIAN_POINT ( 'NONE',  ( -32.45231784149999754, -80.07464407599999845, -22.38373082789999913 ) ) ;
#21150=DIRECTION ( 'NONE',  ( 1.000000000000000000, 0.000000000000000000, 0.000000000000000000 ) ) ;
#21154=DIRECTION ( 'NONE',  ( 0.000000000000000000, -1.000000000000000000, 0.000000000000000000 ) ) ;
#21155=ORIENTED_EDGE ( 'NONE', *, *, #12479, .T. ) ;
#21159=CARTESIAN_POINT ( 'NONE',  ( 30.95803130440000217, -72.48673634319999337, -21.93485012370000220 ) ) ;
#21160=CARTESIAN_POINT ( 'NONE',  ( -13.82310862920000005, -74.00000000000000000, 36.20061004769999613 ) ) ;
#21161=AXIS2_PLACEMENT_3D ( 'NONE', #22827, #3299, #10102 ) ;
#21162=ORIENTED_EDGE ( 'NONE', *, *, #21508, .T. ) ;
#21163=CARTESIAN_POINT ( 'NONE',  ( -39.90536558174056836, -73.91587151486801588, -7.249694362034283301 ) ) ;
#21164=CARTESIAN_POINT ( 'NONE',  ( 21.70178022940000062, -37.60290983899999873, -8.323168728980000708 ) ) ;
#21165=LINE ( 'NONE', #12944, #1416 ) ;
#21166=EDGE_LOOP ( 'NONE', ( #7863, #13474, #8443, #4948 ) ) ;
#21168=CARTESIAN_POINT ( 'NONE',  ( 46.96755458150000351, -74.27975760209999123, -2.596029696810000065 ) ) ;
#21169=EDGE_CURVE ( 'NONE', #12297, #16695, #27003, .T. ) ;
#21170=CARTESIAN_POINT ( 'NONE',  ( -16.35365950510000133, -70.21389208120000092, 23.31707131299999958 ) ) ;
#21171=AXIS2_PLACEMENT_3D ( 'NONE', #9125, #18026, #9275 ) ;
#21173=CARTESIAN_POINT ( 'NONE',  ( 9.205819528820001096, -44.88560226490000105, -22.58640054960000043 ) ) ;
#21179=CARTESIAN_POINT ( 'NONE',  ( 26.85539570430000111, -72.18744871750000414, 10.61487170320000040 ) ) ;
#21181=AXIS2_PLACEMENT_3D ( 'NONE', #11991, #27467, #7513 ) ;
#21184=CARTESIAN_POINT ( 'NONE',  ( -14.01103650240000142, -74.00781516410000904, 36.37014139069999885 ) ) ;
#21188=LINE ( 'NONE', #12278, #1190 ) ;
#21189=CARTESIAN_POINT ( 'NONE',  ( 7.460698725479999927E-15, -73.50000000000000000, 40.00000000000000000 ) ) ;
#21190=CARTESIAN_POINT ( 'NONE',  ( 22.07739135919999640, -36.53304298639999814, -8.940781203140000244 ) ) ;
#21191=CARTESIAN_POINT ( 'NONE',  ( 7.936589523444843586, -35.30313553310306673, -21.23424061165941623 ) ) ;
#21192=EDGE_LOOP ( 'NONE', ( #23924, #7565, #24892, #3096, #24223, #1558 ) ) ;
#21193=CYLINDRICAL_SURFACE ( 'NONE', #21768, 34.89999999999999858 ) ;
#21196=LINE ( 'NONE', #10089, #26562 ) ;
#21197=FACE_OUTER_BOUND ( 'NONE', #18022, .T. ) ;
#21198=CARTESIAN_POINT ( 'NONE',  ( 7.224658177529891034, -73.64797963444465267, 39.39373284322624613 ) ) ;
#21199=CARTESIAN_POINT ( 'NONE',  ( -12.24789267329999909, -65.07443093669999712, 21.96586363990000024 ) ) ;
#21203=CARTESIAN_POINT ( 'NONE',  ( 19.70171045420000056, -28.58309623110000075, -8.968814305740000492 ) ) ;
#21204=DIRECTION ( 'NONE',  ( 0.3889993898738998701, 0.000000000000000000, 0.9212380119587628702 ) ) ;
#21205=ORIENTED_EDGE ( 'NONE', *, *, #15750, .F. ) ;
#21206=CARTESIAN_POINT ( 'NONE',  ( -32.38674382290000153, -80.50000054920000991, -22.17565024390000161 ) ) ;
#21208=EDGE_LOOP ( 'NONE', ( #23342, #4478, #24756, #3242, #16066, #4616, #13542, #13873, #5205 ) ) ;
#21209=DIRECTION ( 'NONE',  ( 0.000000000000000000, -1.000000000000000000, 0.000000000000000000 ) ) ;
#21212=CARTESIAN_POINT ( 'NONE',  ( 20.06309728629999967, -36.00000015629999695, -9.476130053229999461 ) ) ;
#21213=CARTESIAN_POINT ( 'NONE',  ( -7.320980735620000068, -73.89975593090001382, 38.91827670650000215 ) ) ;
#21214=CIRCLE ( 'NONE', #16077, 0.4999999999999982236 ) ;
#21220=PLANE ( 'NONE',  #26336 ) ;
#21225=ORIENTED_EDGE ( 'NONE', *, *, #26512, .F. ) ;
#21226=CARTESIAN_POINT ( 'NONE',  ( -7.713029007999999465, -80.50000000000000000, 40.75609756099999714 ) ) ;
#21229=B_SPLINE_CURVE_WITH_KNOTS ( 'NONE', 3,
 ( #8842, #22828, #27338, #9689, #27492, #1542, #18887, #12431, #25995, #12162, #21075, #14494, #26430, #2111, #11086, #15627, #4563, #10808, #5002, #7348, #20757, #25276, #11545, #22503, #9369, #14191, #14327, #9940, #10347, #28012, #19260, #5442, #9801, #7648, #23360 ),
 .UNSPECIFIED., .F., .F.,
 ( 4, 2, 2, 2, 2, 2, 2, 1, 1, 2, 2, 2, 2, 1, 1, 1, 2, 2, 2, 4 ),
 ( 0.000000000000000000, 0.1249999999999843459, 0.1874999999999762412, 0.2187499999999721889, 0.2499999999999681366, 0.3749999999999550360, 0.4374999999999479305, 0.4687499999999432676, 0.4843749999999405476, 0.4921874999999385492, 0.4999999999999364952, 0.6249999999999171774, 0.6874999999999090727, 0.7187499999999044098, 0.7343749999999011902, 0.7421874999998999689, 0.7460937499999003020, 0.7499999999999007461, 0.8749999999999503730, 1.000000000000000000 ),
 .UNSPECIFIED. ) ;
#21232=EDGE_LOOP ( 'NONE', ( #10062, #774, #17277, #9622 ) ) ;
#21234=EDGE_LOOP ( 'NONE', ( #4556, #1772, #12477, #11453 ) ) ;
#21235=CIRCLE ( 'NONE', #16104, 0.5000000000000004441 ) ;
#21236=CARTESIAN_POINT ( 'NONE',  ( -32.39999999999999858, -82.50000000000000000, 0.000000000000000000 ) ) ;
#21237=CARTESIAN_POINT ( 'NONE',  ( 8.002629315070000970, -36.69307580889999798, -21.43727073079999812 ) ) ;
#21238=CARTESIAN_POINT ( 'NONE',  ( -14.78710422270000002, -79.49999982570000157, 36.35833235879999847 ) ) ;
#21241=ORIENTED_EDGE ( 'NONE', *, *, #17334, .F. ) ;
#21244=CARTESIAN_POINT ( 'NONE',  ( -32.20753451023040270, -74.02757818730215433, -22.07633857551952161 ) ) ;
#21245=CARTESIAN_POINT ( 'NONE',  ( 19.43643804750000115, -34.66800313659999944, -8.988996126470000902 ) ) ;
#21248=DIRECTION ( 'NONE',  ( 0.000000000000000000, 1.000000000000000000, 0.000000000000000000 ) ) ;
#21249=CARTESIAN_POINT ( 'NONE',  ( -2.640725192390000142, -18.61940624680000056, -22.57500579379999905 ) ) ;
#21250=CARTESIAN_POINT ( 'NONE',  ( 36.42998798566536323, -74.03894771716547041, -14.02638628026671164 ) ) ;
#21251=EDGE_LOOP ( 'NONE', ( #10339, #7168, #10895, #12539 ) ) ;
#21252=EDGE_CURVE ( 'NONE', #22701, #8141, #14480, .T. ) ;
#21254=CARTESIAN_POINT ( 'NONE',  ( 30.97576656850000276, -55.50000000000000000, -19.97576656849999921 ) ) ;
#21255=CARTESIAN_POINT ( 'NONE',  ( 8.988513471540001021, -34.97532534249999259, -19.44627031849999810 ) ) ;
#21256=CARTESIAN_POINT ( 'NONE',  ( 7.135467526410000261, -73.65707963269998970, 38.71641004229999794 ) ) ;
#21257=EDGE_LOOP ( 'NONE', ( #25828, #1904, #24048, #23768 ) ) ;
#21259=CARTESIAN_POINT ( 'NONE',  ( -0.6093759117718606788, -79.73250874465735194, 47.22473603108858953 ) ) ;
#21260=ORIENTED_EDGE ( 'NONE', *, *, #21552, .T. ) ;
#21261=CARTESIAN_POINT ( 'NONE',  ( 47.25000000000000000, -75.00000000000000000, -1.242228542250000064E-12 ) ) ;
#21269=CARTESIAN_POINT ( 'NONE',  ( 39.69297836850000039, -73.74954830100000436, 7.260231713059999592 ) ) ;
#21271=DIRECTION ( 'NONE',  ( 0.000000000000000000, -1.000000000000000000, 0.000000000000000000 ) ) ;
#21272=ORIENTED_EDGE ( 'NONE', *, *, #22372, .T. ) ;
#21273=CARTESIAN_POINT ( 'NONE',  ( 26.46310988749999993, -64.24504445130001784, 1.532420830840000026 ) ) ;
#21278=CARTESIAN_POINT ( 'NONE',  ( -2.677516332570000006E-13, -79.50000000000000000, 47.25000000000000000 ) ) ;
#21279=CARTESIAN_POINT ( 'NONE',  ( -14.70960788549999876, -64.89138858019998679, 22.30467294780000032 ) ) ;
#21281=LINE ( 'NONE', #19098, #18814 ) ;
#21282=DIRECTION ( 'NONE',  ( 1.000000000000000000, 0.000000000000000000, 0.000000000000000000 ) ) ;
#21285=CARTESIAN_POINT ( 'NONE',  ( -14.29601107782766611, -74.04677398807629629, 36.24402428269467435 ) ) ;
#21289=DIRECTION ( 'NONE',  ( 1.000000000000000000, 0.000000000000000000, 0.000000000000000000 ) ) ;
#21290=ADVANCED_FACE ( 'NONE', ( #3678 ), #22406, .T. ) ;
#21294=CARTESIAN_POINT ( 'NONE',  ( 20.52569424749999882, -35.38531401670000065, -8.770435444200000319 ) ) ;
#21295=AXIS2_PLACEMENT_3D ( 'NONE', #18281, #25135, #20766 ) ;
#21296=CARTESIAN_POINT ( 'NONE',  ( 19.84586683699999909, -35.72979163229999955, -9.028475981840001552 ) ) ;
#21298=EDGE_LOOP ( 'NONE', ( #6232, #13243, #14396, #4087 ) ) ;
#21301=CARTESIAN_POINT ( 'NONE',  ( -20.91226881666572623, -64.69849613357062879, 14.77252284388811709 ) ) ;
#21303=CARTESIAN_POINT ( 'NONE',  ( 8.472395100179999972, -37.95144078439999902, -21.79230218340000036 ) ) ;
#21311=CARTESIAN_POINT ( 'NONE',  ( 19.82299317300000041, -19.17198320609999840, -8.810535036470000136 ) ) ;
#21312=PLANE ( 'NONE',  #12086 ) ;
#21313=CARTESIAN_POINT ( 'NONE',  ( -14.78710411640000011, -74.45413981500000489, 36.35833236359999887 ) ) ;
#21314=CARTESIAN_POINT ( 'NONE',  ( -1.610129840139999935, -19.46163090469999801, -22.22448219650000212 ) ) ;
#21317=CARTESIAN_POINT ( 'NONE',  ( -1.136716282782229914, -74.21413368979379754, 47.16040998064198675 ) ) ;
#21319=CARTESIAN_POINT ( 'NONE',  ( 9.753828195949997948, -63.05466297450000468, -24.08172833849999961 ) ) ;
#21321=CARTESIAN_POINT ( 'NONE',  ( -10.20110288159999890, -74.00000000000000000, 41.00000000000000000 ) ) ;
#21322=CYLINDRICAL_SURFACE ( 'NONE', #15484, 1.000000000000000888 ) ;
#21324=ADVANCED_FACE ( 'NONE', ( #27746 ), #23093, .T. ) ;
#21327=EDGE_CURVE ( 'NONE', #5681, #16038, #13553, .T. ) ;
#21330=CARTESIAN_POINT ( 'NONE',  ( 20.82960294989999994, -24.50935766780000336, -7.708047809820000040 ) ) ;
#21332=AXIS2_PLACEMENT_3D ( 'NONE', #14958, #18551, #2974 ) ;
#21335=DIRECTION ( 'NONE',  ( 0.6033158263509921237, 0.000000000000000000, -0.7975023596669915671 ) ) ;
#21337=DIRECTION ( 'NONE',  ( 1.000000000000000000, 0.000000000000000000, 0.000000000000000000 ) ) ;
#21340=ORIENTED_EDGE ( 'NONE', *, *, #297, .T. ) ;
#21341=CARTESIAN_POINT ( 'NONE',  ( -13.18623751009999978, -69.39685719070000403, -23.69831535020000146 ) ) ;
#21342=ORIENTED_EDGE ( 'NONE', *, *, #5181, .T. ) ;
#21344=DIRECTION ( 'NONE',  ( -0.000000000000000000, 1.000000000000000000, 0.000000000000000000 ) ) ;
#21346=CARTESIAN_POINT ( 'NONE',  ( 26.47162268830000187, -74.36200393670000608, -29.03680661989999834 ) ) ;
#21348=CARTESIAN_POINT ( 'NONE',  ( -22.44117711659999870, -70.82666672430001142, 16.89270182850000168 ) ) ;
#21350=DIRECTION ( 'NONE',  ( -0.9704142011833033488, 0.000000000000000000, 0.2414462220490755373 ) ) ;
#21351=CARTESIAN_POINT ( 'NONE',  ( -18.59271594794251570, -19.47322495657686403, 13.20546376242789499 ) ) ;
#21352=DIRECTION ( 'NONE',  ( 0.000000000000000000, -1.000000000000000000, 0.000000000000000000 ) ) ;
#21354=CARTESIAN_POINT ( 'NONE',  ( -13.15041533549999997, -18.50000000000000000, 18.48778311079999881 ) ) ;
#21357=EDGE_LOOP ( 'NONE', ( #8872, #8983, #19878, #18030 ) ) ;
#21360=CARTESIAN_POINT ( 'NONE',  ( -2.483024534920000193, -60.10032509980000270, -24.81723791200000306 ) ) ;
#21366=VERTEX_POINT ( 'NONE', #10077 ) ;
#21367=CYLINDRICAL_SURFACE ( 'NONE', #6513, 0.5000000000000012212 ) ;
#21368=ORIENTED_EDGE ( 'NONE', *, *, #18003, .F. ) ;
#21369=CARTESIAN_POINT ( 'NONE',  ( 7.563321429468666146, -37.15172930439049281, -21.49750332032474986 ) ) ;
#21370=CARTESIAN_POINT ( 'NONE',  ( 9.127337073059999639, -35.86526714520000070, -19.87708224909999899 ) ) ;
#21372=CARTESIAN_POINT ( 'NONE',  ( -14.78710393409999924, -79.76388319610001076, 36.35833235529999996 ) ) ;
#21376=DIRECTION ( 'NONE',  ( 0.7071067811865475727, 0.000000000000000000, 0.7071067811865475727 ) ) ;
#21377=VERTEX_POINT ( 'NONE', #27872 ) ;
#21380=CARTESIAN_POINT ( 'NONE',  ( 7.670973119660000172, -34.59820496239999699, -21.21808926809999818 ) ) ;
#21381=CARTESIAN_POINT ( 'NONE',  ( -1.470084592559999903, -18.85499412049999890, -21.97723017330000417 ) ) ;
#21386=EDGE_CURVE ( 'NONE', #25224, #21714, #28442, .T. ) ;
#21390=CARTESIAN_POINT ( 'NONE',  ( 36.47289904670000027, -79.20535029740000255, -14.78463635570000001 ) ) ;
#21391=ORIENTED_EDGE ( 'NONE', *, *, #23341, .F. ) ;
#21395=CARTESIAN_POINT ( 'NONE',  ( -2.629725044940439016, -80.38171235789693014, 46.75630123315725939 ) ) ;
#21397=CARTESIAN_POINT ( 'NONE',  ( 47.16974817210000026, -74.50000513039999817, -1.075739376850000095 ) ) ;
#21398=VERTEX_POINT ( 'NONE', #12965 ) ;
#21404=CARTESIAN_POINT ( 'NONE',  ( 2.486899575159999765E-14, -80.00000000000000000, 7.105427357599999217E-15 ) ) ;
#21408=DIRECTION ( 'NONE',  ( 0.6710140631236515274, 0.000000000000000000, -0.7414446217286144725 ) ) ;
#21409=DIRECTION ( 'NONE',  ( 0.000000000000000000, -1.000000000000000000, 0.000000000000000000 ) ) ;
#21410=CARTESIAN_POINT ( 'NONE',  ( -2.239413966154953695, -79.87344868178468005, 47.08826786916112184 ) ) ;
#21412=CARTESIAN_POINT ( 'NONE',  ( 0.000000000000000000, -82.25000000000000000, -40.00000000000000000 ) ) ;
#21416=CARTESIAN_POINT ( 'NONE',  ( -1.156463699030000125, -55.05312981980000586, -23.31578321539999976 ) ) ;
#21418=CARTESIAN_POINT ( 'NONE',  ( -2.573828320119999624, -39.33785708389999769, -24.78875986600000303 ) ) ;
#21419=EDGE_LOOP ( 'NONE', ( #16429, #16573, #5670, #28685 ) ) ;
#21424=CARTESIAN_POINT ( 'NONE',  ( 28.99618183149999950, -74.19519567169999164, -26.51509840489999803 ) ) ;
#21425=CARTESIAN_POINT ( 'NONE',  ( 8.472395020760000506, -37.95144078679999922, -21.79230213740000011 ) ) ;
#21428=AXIS2_PLACEMENT_3D ( 'NONE', #17686, #8633, #17831 ) ;
#21432=CARTESIAN_POINT ( 'NONE',  ( 20.14104788939999935, -35.73233869100000248, -9.018304108959998899 ) ) ;
#21434=CARTESIAN_POINT ( 'NONE',  ( 19.54973049059999823, -35.76277645470000266, -9.056828148970000214 ) ) ;
#21435=CARTESIAN_POINT ( 'NONE',  ( -22.14844716308801864, -79.50000004209999815, -32.75504888958925420 ) ) ;
#21438=EDGE_CURVE ( 'NONE', #18300, #12333, #17744, .T. ) ;
#21441=CARTESIAN_POINT ( 'NONE',  ( 8.998660423299998712, -44.89607406070000195, -22.33592606139999859 ) ) ;
#21444=ORIENTED_EDGE ( 'NONE', *, *, #419, .F. ) ;
#21446=EDGE_CURVE ( 'NONE', #18925, #13695, #26124, .T. ) ;
#21450=CARTESIAN_POINT ( 'NONE',  ( 26.43538883849999976, -72.55114739969998539, 11.02537517960000102 ) ) ;
#21453=CARTESIAN_POINT ( 'NONE',  ( 19.29218169219999979, -18.50000000000000000, -7.924293390789999947 ) ) ;
#21455=CARTESIAN_POINT ( 'NONE',  ( -14.77250568370000039, -74.40829841730000282, 36.35986053050000066 ) ) ;
#21456=CARTESIAN_POINT ( 'NONE',  ( -2.535581654609999624, -19.42987840509999842, -23.25781427689999958 ) ) ;
#21461=CARTESIAN_POINT ( 'NONE',  ( 7.442798598269999566, -60.60073824219999494, -22.42221163419999996 ) ) ;
#21463=CARTESIAN_POINT ( 'NONE',  ( 22.87891866909999905, -57.82174915179999886, 10.24673290389999991 ) ) ;
#21465=VERTEX_POINT ( 'NONE', #6425 ) ;
#21468=CIRCLE ( 'NONE', #556, 7.750000000000000000 ) ;
#21474=B_SPLINE_SURFACE_WITH_KNOTS ( 'NONE', 5, 5, ( 
 ( #12520, #21432, #28402, #3389, #26085, #1490 ),
 ( #21710, #19382, #14988, #25674, #19110, #12383 ),
 ( #19243, #5569, #3525, #17196, #12660, #10329 ),
 ( #3936, #1759, #25944, #8166, #28259, #17053 ),
 ( #19517, #14451, #27995, #12253, #25815, #1218 ),
 ( #21571, #10059, #21294, #1346, #10194, #16921 ) ),
 .UNSPECIFIED., .F., .F., .F.,
 ( 6, 6 ),
 ( 6, 6 ),
 ( 1.601061932509999952, 3.163829236780000276 ),
 ( 0.000000000000000000, 2.000000000000000000 ),
 .UNSPECIFIED. ) ;
#21481=EDGE_CURVE ( 'NONE', #17168, #10513, #23348, .T. ) ;
#21482=EDGE_CURVE ( 'NONE', #14724, #2204, #21468, .T. ) ;
#21485=CIRCLE ( 'NONE', #6114, 0.5000000000000004441 ) ;
#21487=EDGE_CURVE ( 'NONE', #10298, #24581, #19266, .T. ) ;
#21489=CARTESIAN_POINT ( 'NONE',  ( 26.60005552420000186, -73.86497505609999337, -28.90969314500000209 ) ) ;
#21490=EDGE_CURVE ( 'NONE', #10529, #26232, #8879, .T. ) ;
#21494=CARTESIAN_POINT ( 'NONE',  ( -11.81899278030000033, -64.69849622489999774, -22.71259345900000071 ) ) ;
#21495=CARTESIAN_POINT ( 'NONE',  ( 7.316573060279999652, -35.82074236369999909, -21.43354451849999975 ) ) ;
#21496=CARTESIAN_POINT ( 'NONE',  ( -41.00000000000000000, -74.00000000000000000, 10.20110288159999890 ) ) ;
#21497=ORIENTED_EDGE ( 'NONE', *, *, #22344, .F. ) ;
#21499=EDGE_LOOP ( 'NONE', ( #281, #24008 ) ) ;
#21500=CARTESIAN_POINT ( 'NONE',  ( 22.72991323779999817, -37.99098077740000434, -9.322992626879999634 ) ) ;
#21502=CARTESIAN_POINT ( 'NONE',  ( -1.512642400649999885, -63.93339545899999621, -24.75805884960000114 ) ) ;
#21504=TOROIDAL_SURFACE ( 'NONE', #15927, 2.500000000000000000, 0.5000000000000000000 ) ;
#21506=ORIENTED_EDGE ( 'NONE', *, *, #663, .T. ) ;
#21507=CARTESIAN_POINT ( 'NONE',  ( 21.18059972589999873, -34.84004059659999797, -7.857545738520000711 ) ) ;
#21508=EDGE_CURVE ( 'NONE', #23613, #21377, #20542, .T. ) ;
#21509=LINE ( 'NONE', #19329, #24139 ) ;
#21510=EDGE_LOOP ( 'NONE', ( #16311, #15925, #27501, #15173 ) ) ;
#21513=PLANE ( 'NONE',  #5789 ) ;
#21514=DIRECTION ( 'NONE',  ( 0.000000000000000000, 1.000000000000000000, 0.000000000000000000 ) ) ;
#21515=EDGE_CURVE ( 'NONE', #13115, #5438, #25657, .T. ) ;
#21516=CARTESIAN_POINT ( 'NONE',  ( 21.88147998950000073, -19.49009541680000268, 9.576298402129999943 ) ) ;
#21519=ORIENTED_EDGE ( 'NONE', *, *, #24844, .T. ) ;
#21529=CARTESIAN_POINT ( 'NONE',  ( 11.21511754571216990, -69.74181458266943423, -26.64805835954446067 ) ) ;
#21531=CARTESIAN_POINT ( 'NONE',  ( 36.60240428190000017, -80.39630767040000592, -14.17343997929999944 ) ) ;
#21537=ORIENTED_EDGE ( 'NONE', *, *, #10717, .F. ) ;
#21538=CARTESIAN_POINT ( 'NONE',  ( 47.17354815139999857, -74.60193236360001379, -1.119565185129999918 ) ) ;
#21539=ORIENTED_EDGE ( 'NONE', *, *, #24715, .T. ) ;
#21540=CARTESIAN_POINT ( 'NONE',  ( 22.51417952139999912, -55.00753887609999992, 10.12166766410000029 ) ) ;
#21546=B_SPLINE_CURVE_WITH_KNOTS ( 'NONE', 3,
 ( #13193, #8670, #21955, #20054, #21801, #2144 ),
 .UNSPECIFIED., .F., .F.,
 ( 4, 2, 4 ),
 ( 0.000000000000000000, 0.5000000000000000000, 1.000000000000000000 ),
 .UNSPECIFIED. ) ;
#21548=CARTESIAN_POINT ( 'NONE',  ( -21.91703890630000018, -80.37806415250000214, -32.56305777900000464 ) ) ;
#21549=CARTESIAN_POINT ( 'NONE',  ( 20.14180970569999829, -45.99935878759999497, 11.02192488110000035 ) ) ;
#21552=EDGE_CURVE ( 'NONE', #16196, #3267, #14931, .T. ) ;
#21557=CARTESIAN_POINT ( 'NONE',  ( -1.452960264739999952, -55.04870336940000186, -23.42848252749999816 ) ) ;
#21558=AXIS2_PLACEMENT_3D ( 'NONE', #13597, #3133, #5004 ) ;
#21559=CARTESIAN_POINT ( 'NONE',  ( 10.61988563626112558, -72.59634600277628635, -26.81031528543675435 ) ) ;
#21561=ORIENTED_EDGE ( 'NONE', *, *, #23587, .T. ) ;
#21567=AXIS2_PLACEMENT_3D ( 'NONE', #15147, #4530, #13411 ) ;
#21571=CARTESIAN_POINT ( 'NONE',  ( 19.49544327699999968, -35.50000000000000000, -8.986258411389998813 ) ) ;
#21573=AXIS2_PLACEMENT_3D ( 'NONE', #80, #9080, #20162 ) ;
#21574=CARTESIAN_POINT ( 'NONE',  ( 21.57170138819999750, -37.33907283540000321, -8.016383387539999461 ) ) ;
#21575=CARTESIAN_POINT ( 'NONE',  ( 9.038647564319999717, -35.72724395809999720, -19.55068592700000352 ) ) ;
#21578=EDGE_CURVE ( 'NONE', #5350, #2148, #236, .T. ) ;
#21579=DIRECTION ( 'NONE',  ( 0.000000000000000000, 1.000000000000000000, 0.000000000000000000 ) ) ;
#21582=CARTESIAN_POINT ( 'NONE',  ( 7.233371418730000002, -44.93343662230000035, -21.75421831149999718 ) ) ;
#21587=CARTESIAN_POINT ( 'NONE',  ( 23.90606501070000078, -57.45864775100000088, 0.8443138621939999533 ) ) ;
#21588=CARTESIAN_POINT ( 'NONE',  ( 24.84525630199999924, -69.52108470319998901, 11.33455677210000090 ) ) ;
#21591=CARTESIAN_POINT ( 'NONE',  ( -39.85912817270000374, -74.23958658479999428, 7.332335648789999993 ) ) ;
#21592=CARTESIAN_POINT ( 'NONE',  ( -14.52836087100000029, -74.22231530550000400, 36.83217634790000261 ) ) ;
#21596=CONICAL_SURFACE ( 'NONE', #25345, 21.99999999999999645, 0.03490658503990158590 ) ;
#21599=B_SPLINE_CURVE_WITH_KNOTS ( 'NONE', 3,
 ( #2201, #26681, #13706, #2503, #11357, #20261, #3364, #14428, #27706, #9620, #1063, #23319, #7871 ),
 .UNSPECIFIED., .F., .F.,
 ( 4, 2, 1, 1, 1, 2, 2, 4 ),
 ( 0.000000000000000000, 0.2499999999999817923, 0.3749999999999705236, 0.4374999999999647504, 0.4687499999999620859, 0.4843749999999605316, 0.4999999999999589217, 1.000000000000000000 ),
 .UNSPECIFIED. ) ;
#21601=DIRECTION ( 'NONE',  ( 0.000000000000000000, 0.000000000000000000, -1.000000000000000000 ) ) ;
#21603=CARTESIAN_POINT ( 'NONE',  ( 20.91274138339999666, -58.78702526330000211, 10.73875272749999965 ) ) ;
#21609=EDGE_CURVE ( 'NONE', #9115, #27225, #2405, .T. ) ;
#21610=CARTESIAN_POINT ( 'NONE',  ( 7.595444726729600567E-15, -74.00000000000000000, 32.25000000000000000 ) ) ;
#21613=CARTESIAN_POINT ( 'NONE',  ( 21.51248591490000095, -18.50000000000000000, 1.147234204320000117 ) ) ;
#21614=VECTOR ( 'NONE', #21095, 1000.000000000000000 ) ;
#21616=CARTESIAN_POINT ( 'NONE',  ( -32.75000000000000000, -73.00000000000000000, 2.464695114669999848E-15 ) ) ;
#21617=ORIENTED_EDGE ( 'NONE', *, *, #10924, .T. ) ;
#21619=LINE ( 'NONE', #26418, #10219 ) ;
#21622=AXIS2_PLACEMENT_3D ( 'NONE', #22954, #22802, #18572 ) ;
#21623=( NAMED_UNIT ( * ) PLANE_ANGLE_UNIT ( ) SI_UNIT ( $, .RADIAN. ) );
#21625=ORIENTED_EDGE ( 'NONE', *, *, #26319, .F. ) ;
#21627=CARTESIAN_POINT ( 'NONE',  ( -38.67409491847346459, -73.94611239985914608, -7.370697001239630453 ) ) ;
#21628=B_SPLINE_CURVE_WITH_KNOTS ( 'NONE', 5,
 ( #23051, #17939, #919, #22461, #18080, #7017 ),
 .UNSPECIFIED., .F., .F.,
 ( 6, 6 ),
 ( 0.000000000000000000, 1.000000000000000000 ),
 .UNSPECIFIED. ) ;
#21632=CARTESIAN_POINT ( 'NONE',  ( -22.52693219800000080, -70.43934371539999972, 17.54847698860000094 ) ) ;
#21633=CIRCLE ( 'NONE', #8130, 2.500000000000002220 ) ;
#21635=CARTESIAN_POINT ( 'NONE',  ( -18.64599988254608220, -19.47504441210472592, 13.34621241184425244 ) ) ;
#21636=CARTESIAN_POINT ( 'NONE',  ( 6.944365432299999696, -36.14100883020000055, -21.52374318029999856 ) ) ;
#21637=DIRECTION ( 'NONE',  ( 0.000000000000000000, -1.000000000000000000, 0.000000000000000000 ) ) ;
#21639=CARTESIAN_POINT ( 'NONE',  ( 22.02882315030000271, -19.46510050329999686, -0.4636558402470000173 ) ) ;
#21640=AXIS2_PLACEMENT_3D ( 'NONE', #23095, #24977, #16220 ) ;
#21641=ORIENTED_EDGE ( 'NONE', *, *, #22000, .F. ) ;
#21644=CARTESIAN_POINT ( 'NONE',  ( -2.486260167500000229, -58.65571127909999660, -24.68408288270000028 ) ) ;
#21645=EDGE_CURVE ( 'NONE', #27146, #22782, #9899, .T. ) ;
#21647=DIRECTION ( 'NONE',  ( 0.000000000000000000, -1.000000000000000000, 0.000000000000000000 ) ) ;
#21648=EDGE_CURVE ( 'NONE', #1165, #5725, #17229, .T. ) ;
#21649=CARTESIAN_POINT ( 'NONE',  ( -19.51583823490001279, -52.61368720150016998, 13.56962763330000676 ) ) ;
#21652=VERTEX_POINT ( 'NONE', #7028 ) ;
#21653=CARTESIAN_POINT ( 'NONE',  ( 21.47059222220000052, -36.19499449340000297, -7.248977034690000210 ) ) ;
#21656=DIRECTION ( 'NONE',  ( 0.000000000000000000, -1.000000000000000000, 0.000000000000000000 ) ) ;
#21657=B_SPLINE_CURVE_WITH_KNOTS ( 'NONE', 3,
 ( #28140, #12950, #8174, #17060, #28411, #4081 ),
 .UNSPECIFIED., .F., .F.,
 ( 4, 2, 4 ),
 ( 0.000000000000000000, 0.5000000000000000000, 1.000000000000000000 ),
 .UNSPECIFIED. ) ;
#21658=CARTESIAN_POINT ( 'NONE',  ( 39.31221710949670012, -74.09469053480707146, 7.479534729103155755 ) ) ;
#21660=CARTESIAN_POINT ( 'NONE',  ( -31.89935321680000158, -74.00000000000000000, -21.99985828019999801 ) ) ;
#21661=CARTESIAN_POINT ( 'NONE',  ( -24.21840725559999896, -79.50000000000000000, -34.11790219230000076 ) ) ;
#21662=ORIENTED_EDGE ( 'NONE', *, *, #12515, .T. ) ;
#21663=DIRECTION ( 'NONE',  ( 0.000000000000000000, 1.000000000000000000, 0.000000000000000000 ) ) ;
#21666=ORIENTED_EDGE ( 'NONE', *, *, #7093, .F. ) ;
#21668=CARTESIAN_POINT ( 'NONE',  ( -32.33029131960000058, -74.08184093439999174, -21.92820895030000017 ) ) ;
#21669=CARTESIAN_POINT ( 'NONE',  ( 36.61516926800000249, -79.38053706460000569, -14.70489075899999953 ) ) ;
#21674=CARTESIAN_POINT ( 'NONE',  ( -1.067886454847412958, -79.90307488451320239, 47.17292579724168888 ) ) ;
#21675=ADVANCED_FACE ( 'NONE', ( #18241 ), #12622, .T. ) ;
#21677=CARTESIAN_POINT ( 'NONE',  ( -12.08584015489836183, -69.49854784199777669, -25.11440668764106121 ) ) ;
#21679=VERTEX_POINT ( 'NONE', #25659 ) ;
#21682=CARTESIAN_POINT ( 'NONE',  ( -7.260248548399999891, -73.97917265380000629, -40.03821526680000176 ) ) ;
#21685=CARTESIAN_POINT ( 'NONE',  ( 22.60430443959684510, -36.06167118559999807, -10.71318590909911528 ) ) ;
#21686=DIRECTION ( 'NONE',  ( 0.7071067811865470176, 0.000000000000000000, 0.7071067811865480168 ) ) ;
#21692=CARTESIAN_POINT ( 'NONE',  ( -8.841308419197195789, -80.50000000000000000, 38.90215371868703187 ) ) ;
#21696=DIRECTION ( 'NONE',  ( -0.000000000000000000, 1.000000000000000000, 0.000000000000000000 ) ) ;
#21701=CARTESIAN_POINT ( 'NONE',  ( 19.09701464850000008, -18.50000000000000000, 9.226637575699999871 ) ) ;
#21705=DIRECTION ( 'NONE',  ( 0.9295286103719527793, 0.000000000000000000, 0.3687499999999814260 ) ) ;
#21706=EDGE_CURVE ( 'NONE', #1954, #3056, #11230, .T. ) ;
#21707=ADVANCED_FACE ( 'NONE', ( #5130 ), #15404, .F. ) ;
#21708=ORIENTED_EDGE ( 'NONE', *, *, #9238, .T. ) ;
#21710=CARTESIAN_POINT ( 'NONE',  ( 19.55164490770000185, -35.69157978159999800, -9.020399939569999859 ) ) ;
#21711=VERTEX_POINT ( 'NONE', #3515 ) ;
#21712=CARTESIAN_POINT ( 'NONE',  ( 19.55068585879999787, -35.72724450129999951, -9.038647844319999791 ) ) ;
#21713=FACE_OUTER_BOUND ( 'NONE', #9685, .T. ) ;
#21714=VERTEX_POINT ( 'NONE', #9628 ) ;
#21720=DIRECTION ( 'NONE',  ( 1.000000000000000000, 0.000000000000000000, 0.000000000000000000 ) ) ;
#21721=CARTESIAN_POINT ( 'NONE',  ( -9.752576846380001996, -18.50000000000000000, -19.83503857510000046 ) ) ;
#21725=CARTESIAN_POINT ( 'NONE',  ( 23.42943742290000131, -42.25468912520000231, 0.9114797856909999663 ) ) ;
#21726=CARTESIAN_POINT ( 'NONE',  ( 22.90783306289999999, -66.63438074019998680, 12.00069599370000084 ) ) ;
#21728=VERTEX_POINT ( 'NONE', #27582 ) ;
#21730=DIRECTION ( 'NONE',  ( 0.000000000000000000, 1.000000000000000000, 0.000000000000000000 ) ) ;
#21731=LINE ( 'NONE', #1368, #21808 ) ;
#21732=DIRECTION ( 'NONE',  ( 1.000000000000000000, 0.000000000000000000, 0.000000000000000000 ) ) ;
#21735=VECTOR ( 'NONE', #1395, 1000.000000000000000 ) ;
#21736=FACE_OUTER_BOUND ( 'NONE', #12966, .T. ) ;
#21737=DIRECTION ( 'NONE',  ( 1.000000000000000000, 0.000000000000000000, 0.000000000000000000 ) ) ;
#21740=DIRECTION ( 'NONE',  ( -0.9852992387259376095, 0.000000000000000000, 0.1708373792999886009 ) ) ;
#21742=VERTEX_POINT ( 'NONE', #19096 ) ;
#21747=CARTESIAN_POINT ( 'NONE',  ( 20.63161943080000071, -19.46510050319999863, -7.734358783100000245 ) ) ;
#21749=DIRECTION ( 'NONE',  ( 0.9704142011833034598, 0.000000000000000000, -0.2414462220490750377 ) ) ;
#21753=CIRCLE ( 'NONE', #9186, 7.750000000000000000 ) ;
#21755=DIRECTION ( 'NONE',  ( 1.000000000000000000, 0.000000000000000000, -1.665334536939999828E-16 ) ) ;
#21757=CARTESIAN_POINT ( 'NONE',  ( -12.17175180279999935, -57.47855601759999900, -19.93971687999999887 ) ) ;
#21759=ORIENTED_EDGE ( 'NONE', *, *, #24577, .F. ) ;
#21761=EDGE_LOOP ( 'NONE', ( #19153, #22463, #25990, #6011 ) ) ;
#21764=DIRECTION ( 'NONE',  ( 0.000000000000000000, 1.000000000000000000, 0.000000000000000000 ) ) ;
#21765=DIRECTION ( 'NONE',  ( 0.1237356522920125546, 0.000000000000000000, -0.9923152162251016595 ) ) ;
#21767=DIRECTION ( 'NONE',  ( 0.000000000000000000, 1.000000000000000000, 0.000000000000000000 ) ) ;
#21768=AXIS2_PLACEMENT_3D ( 'NONE', #9670, #11861, #1245 ) ;
#21769=ORIENTED_EDGE ( 'NONE', *, *, #3002, .F. ) ;
#21771=CARTESIAN_POINT ( 'NONE',  ( -22.67747013279999990, -69.73397779950001052, 15.15635250419999913 ) ) ;
#21775=CARTESIAN_POINT ( 'NONE',  ( -19.02940910017253273, -19.48522775728694612, 13.93404945096885683 ) ) ;
#21776=CARTESIAN_POINT ( 'NONE',  ( 7.146354963110000291, -36.17740051239999843, -21.48176990560000021 ) ) ;
#21778=VERTEX_POINT ( 'NONE', #14438 ) ;
#21779=CARTESIAN_POINT ( 'NONE',  ( 36.62466543389999885, -74.65121094670000446, -14.68734461939999925 ) ) ;
#21780=CARTESIAN_POINT ( 'NONE',  ( 21.78369645919999797, -36.06096454580000454, -10.41102218880000052 ) ) ;
#21781=CARTESIAN_POINT ( 'NONE',  ( -1.156338024719999913, -58.78702526330000211, -23.48034166449999915 ) ) ;
#21784=CARTESIAN_POINT ( 'NONE',  ( -19.87158930579999705, -56.22908209860000284, 14.19280044929999995 ) ) ;
#21786=ORIENTED_EDGE ( 'NONE', *, *, #8960, .F. ) ;
#21789=ORIENTED_EDGE ( 'NONE', *, *, #4069, .T. ) ;
#21794=CARTESIAN_POINT ( 'NONE',  ( 22.16575857890000023, -39.31812514059999586, 9.877484424130001273 ) ) ;
#21795=CARTESIAN_POINT ( 'NONE',  ( -22.12521137138542215, -74.07932799455450379, -32.40737826886834938 ) ) ;
#21796=EDGE_CURVE ( 'NONE', #22782, #11457, #3376, .T. ) ;
#21797=CARTESIAN_POINT ( 'NONE',  ( 21.61044917590000480, -19.17414499179999865, 9.484325925899998566 ) ) ;
#21798=CARTESIAN_POINT ( 'NONE',  ( -32.42291149912640691, -74.08416876105088988, -22.12919252830631933 ) ) ;
#21799=CARTESIAN_POINT ( 'NONE',  ( -20.08103059729999984, -57.43018248439999951, 14.46712379729999931 ) ) ;
#21801=CARTESIAN_POINT ( 'NONE',  ( -11.86518140747143235, -72.15620726827764031, -26.36366794161594385 ) ) ;
#21807=EDGE_CURVE ( 'NONE', #6300, #8623, #3657, .T. ) ;
#21808=VECTOR ( 'NONE', #28283, 1000.000000000000000 ) ;
#21810=CARTESIAN_POINT ( 'NONE',  ( -31.99064106590000023, -74.00000000000000000, -21.95840602359999849 ) ) ;
#21811=ORIENTED_EDGE ( 'NONE', *, *, #13377, .F. ) ;
#21812=CIRCLE ( 'NONE', #12947, 38.75000000000000000 ) ;
#21814=CIRCLE ( 'NONE', #14346, 3.750000000000000000 ) ;
#21822=CARTESIAN_POINT ( 'NONE',  ( 22.84303034490000073, -56.20810645120000260, 10.22595161340000125 ) ) ;
#21823=ORIENTED_EDGE ( 'NONE', *, *, #24144, .T. ) ;
#21824=CARTESIAN_POINT ( 'NONE',  ( 9.885503723209998483, -36.00000000000000000, -20.33566493420000043 ) ) ;
#21825=CARTESIAN_POINT ( 'NONE',  ( -3.108624468950000298E-16, -74.00000000000000000, -1.554312234480000048E-16 ) ) ;
#21827=CARTESIAN_POINT ( 'NONE',  ( 8.685017520700000659, -37.33819206249999922, -21.91842612469999807 ) ) ;
#21829=CARTESIAN_POINT ( 'NONE',  ( 24.70601165868461990, -65.70112750257325729, 10.85168987944911656 ) ) ;
#21831=CIRCLE ( 'NONE', #27463, 3.749999999999996447 ) ;
#21834=CARTESIAN_POINT ( 'NONE',  ( -32.20769381560000255, -80.34292075950000367, -22.43272066100000117 ) ) ;
#21836=CARTESIAN_POINT ( 'NONE',  ( 4.426600958609999879E-15, -69.00000000000000000, 43.75000000000000000 ) ) ;
#21837=CARTESIAN_POINT ( 'NONE',  ( -1.993723132830000244, -52.61368720150000655, -23.68602550419999986 ) ) ;
#21838=EDGE_CURVE ( 'NONE', #14636, #10981, #930, .T. ) ;
#21840=CARTESIAN_POINT ( 'NONE',  ( -19.12703695859999797, -18.50000000000000000, 14.91269771249999998 ) ) ;
#21842=EDGE_CURVE ( 'NONE', #7826, #19383, #25900, .T. ) ;
#21843=DIRECTION ( 'NONE',  ( 1.000000000000000000, 0.000000000000000000, 0.000000000000000000 ) ) ;
#21844=CARTESIAN_POINT ( 'NONE',  ( 20.30102379280000235, -72.00000000000000000, -30.97095677779999789 ) ) ;
#21845=CARTESIAN_POINT ( 'NONE',  ( 4.656214649959999954E-15, -79.00000000000000000, 40.00000000000000000 ) ) ;
#21846=CARTESIAN_POINT ( 'NONE',  ( 21.00696503170000184, -18.50000000000000000, 8.444293349240000524 ) ) ;
#21847=CARTESIAN_POINT ( 'NONE',  ( -40.00000000000000000, -82.25000000000000000, 0.000000000000000000 ) ) ;
#21855=ORIENTED_EDGE ( 'NONE', *, *, #27910, .F. ) ;
#21856=CARTESIAN_POINT ( 'NONE',  ( 21.50685431550000004, -37.36994930320000208, -7.661821680550000124 ) ) ;
#21858=ORIENTED_EDGE ( 'NONE', *, *, #27055, .F. ) ;
#21860=CARTESIAN_POINT ( 'NONE',  ( -3.378235408309124388, -68.15838326003131442, -27.58918776656260619 ) ) ;
#21864=EDGE_CURVE ( 'NONE', #8967, #11422, #14450, .T. ) ;
#21866=CARTESIAN_POINT ( 'NONE',  ( 40.65853658540000026, -84.00000000000000000, 6.717799458580000049 ) ) ;
#21867=CARTESIAN_POINT ( 'NONE',  ( -10.53872106220000049, -18.50000000000000000, -18.20862928879999743 ) ) ;
#21870=EDGE_CURVE ( 'NONE', #24612, #26673, #4206, .T. ) ;
#21872=CARTESIAN_POINT ( 'NONE',  ( 23.29682936289999873, -49.86909869750000013, 0.3487798571490000055 ) ) ;
#21873=CARTESIAN_POINT ( 'NONE',  ( 22.77339862950000082, -64.89165510060000486, 10.97889282110000053 ) ) ;
#21874=CARTESIAN_POINT ( 'NONE',  ( 38.90877162584872906, -73.50999119020812600, 7.168130346644877804 ) ) ;
#21877=CARTESIAN_POINT ( 'NONE',  ( -38.68350751799999898, -73.93831497249999529, 7.318372426699999878 ) ) ;
#21880=ORIENTED_EDGE ( 'NONE', *, *, #23715, .F. ) ;
#21883=CARTESIAN_POINT ( 'NONE',  ( 27.79198761910000215, -68.38614792650000140, 2.092073158110000275 ) ) ;
#21885=CARTESIAN_POINT ( 'NONE',  ( 9.368358256079998725, -60.33817349190000101, -23.16693853690000182 ) ) ;
#21888=CARTESIAN_POINT ( 'NONE',  ( -11.90025794910000023, -42.27249569760000014, -19.48331447349999834 ) ) ;
#21889=ORIENTED_EDGE ( 'NONE', *, *, #23981, .F. ) ;
#21890=B_SPLINE_CURVE_WITH_KNOTS ( 'NONE', 5,
 ( #28386, #5951, #17470, #15247, #8417, #14835 ),
 .UNSPECIFIED., .F., .F.,
 ( 6, 6 ),
 ( 0.000000000000000000, 1.000000000000000000 ),
 .UNSPECIFIED. ) ;
#21896=ORIENTED_EDGE ( 'NONE', *, *, #28767, .T. ) ;
#21898=CIRCLE ( 'NONE', #17264, 0.5000000000000004441 ) ;
#21900=CARTESIAN_POINT ( 'NONE',  ( 20.42956111930000063, -25.51643932219999655, -8.516251604709999867 ) ) ;
#21901=CARTESIAN_POINT ( 'NONE',  ( -8.841308419149999764, -80.00000000000000000, 38.90215371869999927 ) ) ;
#21904=CARTESIAN_POINT ( 'NONE',  ( -11.58789126345519982, -27.06771711593889407, -19.05193615919498740 ) ) ;
#21906=CARTESIAN_POINT ( 'NONE',  ( -36.23922253580000330, -79.50000000000000000, -27.04683438039999999 ) ) ;
#21908=CARTESIAN_POINT ( 'NONE',  ( 9.056984553609998656, -35.76308213440000117, -19.54972227260000039 ) ) ;
#21909=CARTESIAN_POINT ( 'NONE',  ( 19.97576656849999921, -72.00000000000000000, -19.97576656849999921 ) ) ;
#21912=CARTESIAN_POINT ( 'NONE',  ( 21.03849606329999844, -18.50000000000000000, -0.02248551888909999796 ) ) ;
#21913=DIRECTION ( 'NONE',  ( 1.000000000000000000, 0.000000000000000000, 0.000000000000000000 ) ) ;
#21919=CYLINDRICAL_SURFACE ( 'NONE', #21573, 7.249999999999999112 ) ;
#21924=CARTESIAN_POINT ( 'NONE',  ( 19.26850085170000071, -29.42970386789999893, -8.998040626839999945 ) ) ;
#21925=AXIS2_PLACEMENT_3D ( 'NONE', #969, #10216, #16656 ) ;
#21927=AXIS2_PLACEMENT_3D ( 'NONE', #4818, #13696, #22598 ) ;
#21928=CARTESIAN_POINT ( 'NONE',  ( -10.85248982675889273, -18.97801304286212343, -21.92849394884687086 ) ) ;
#21929=CIRCLE ( 'NONE', #24258, 0.4999999999999982236 ) ;
#21930=CARTESIAN_POINT ( 'NONE',  ( 22.15413943410000286, -37.05706116329999134, -9.219199529280000860 ) ) ;
#21932=ADVANCED_FACE ( 'NONE', ( #10453, #28247 ), #19788, .T. ) ;
#21933=CARTESIAN_POINT ( 'NONE',  ( -0.8798048959290000193, -61.87790347820000392, -23.94595848790000048 ) ) ;
#21935=CARTESIAN_POINT ( 'NONE',  ( -19.84861352869999962, -53.84434310259999279, 12.07737518400000098 ) ) ;
#21936=DIRECTION ( 'NONE',  ( -0.2414462220490755373, 0.000000000000000000, -0.9704142011833032377 ) ) ;
#21938=AXIS2_PLACEMENT_3D ( 'NONE', #26136, #28176, #12842 ) ;
#21939=CARTESIAN_POINT ( 'NONE',  ( 21.28729238020000025, -35.15980207439999816, -7.664900974450000071 ) ) ;
#21940=CARTESIAN_POINT ( 'NONE',  ( -16.67828388959999941, -74.00000000000000000, 44.75374114529999758 ) ) ;
#21943=CARTESIAN_POINT ( 'NONE',  ( 7.693905362600673925, -37.38950372099960617, -21.51648389446061316 ) ) ;
#21945=ORIENTED_EDGE ( 'NONE', *, *, #22654, .F. ) ;
#21946=ADVANCED_FACE ( 'NONE', ( #1744 ), #14840, .F. ) ;
#21947=FACE_OUTER_BOUND ( 'NONE', #27305, .T. ) ;
#21948=CARTESIAN_POINT ( 'NONE',  ( 20.85236623999999850, -26.08233090739999938, 9.582502883489999235 ) ) ;
#21950=CARTESIAN_POINT ( 'NONE',  ( 22.13285133049999587, -19.49504784870000051, 9.709488547299999439 ) ) ;
#21951=CARTESIAN_POINT ( 'NONE',  ( 9.438993784210000015, -64.72767716790001202, -23.93801147259999951 ) ) ;
#21955=CARTESIAN_POINT ( 'NONE',  ( -12.36776282346795597, -72.59721320749554252, -25.84214607925492402 ) ) ;
#21958=CARTESIAN_POINT ( 'NONE',  ( 22.36688849876826168, -59.04651452996991878, -7.100983198977605326 ) ) ;
#21959=EDGE_LOOP ( 'NONE', ( #21444, #25579 ) ) ;
#21960=CARTESIAN_POINT ( 'NONE',  ( 47.25000000000000000, -69.50000000000000000, 2.433892081919999696E-15 ) ) ;
#21961=CARTESIAN_POINT ( 'NONE',  ( -32.51469473070000049, -74.18397341870000616, -21.79791327519999911 ) ) ;
#21964=EDGE_CURVE ( 'NONE', #25324, #27945, #25552, .T. ) ;
#21965=CARTESIAN_POINT ( 'NONE',  ( 24.88097934669864131, -39.24428776213493109, 1.395120059140831037 ) ) ;
#21966=ORIENTED_EDGE ( 'NONE', *, *, #6717, .F. ) ;
#21971=CARTESIAN_POINT ( 'NONE',  ( 25.32712259480000228, -57.40875702469999453, 1.379782074460000230 ) ) ;
#21972=ADVANCED_FACE ( 'NONE', ( #6388 ), #9885, .T. ) ;
#21975=CARTESIAN_POINT ( 'NONE',  ( 1.678657213230000024E-14, -74.00000000000000000, 7.838174553849999450E-15 ) ) ;
#21978=CARTESIAN_POINT ( 'NONE',  ( 9.237424541170000225, -36.00000000019999646, -20.64008957659999766 ) ) ;
#21979=CARTESIAN_POINT ( 'NONE',  ( -11.46863496920000003, -57.40875702469999453, -22.62382260909999943 ) ) ;
#21980=VECTOR ( 'NONE', #4011, 1000.000000000000000 ) ;
#21986=CARTESIAN_POINT ( 'NONE',  ( -2.583988345239999873, -57.40875702400000336, -25.23271569159999927 ) ) ;
#21988=CARTESIAN_POINT ( 'NONE',  ( 11.31200901364189448, -72.30581792555656762, -26.97931566277052795 ) ) ;
#21989=CARTESIAN_POINT ( 'NONE',  ( -4.439198032609999743E-16, -82.25000000000000000, 47.25000000000000000 ) ) ;
#21990=ORIENTED_EDGE ( 'NONE', *, *, #4415, .F. ) ;
#21991=DIRECTION ( 'NONE',  ( -0.9993816408608721114, 0.000000000000000000, 0.03516156865429537204 ) ) ;
#21994=DIRECTION ( 'NONE',  ( 0.000000000000000000, 1.000000000000000000, 0.000000000000000000 ) ) ;
#21998=VECTOR ( 'NONE', #14251, 1000.000000000000000 ) ;
#21999=DIRECTION ( 'NONE',  ( 0.9995627462972741517, 0.000000000000000000, -0.02956883857460800707 ) ) ;
#22000=EDGE_CURVE ( 'NONE', #26338, #3822, #24909, .T. ) ;
#22001=CIRCLE ( 'NONE', #27614, 39.75000000000000000 ) ;
#22002=FACE_BOUND ( 'NONE', #26165, .T. ) ;
#22003=ADVANCED_FACE ( 'NONE', ( #2765 ), #14951, .T. ) ;
#22008=CARTESIAN_POINT ( 'NONE',  ( 7.491375974803306192, -18.50000000000000000, -19.98345406245123357 ) ) ;
#22010=ORIENTED_EDGE ( 'NONE', *, *, #8866, .F. ) ;
#22011=CARTESIAN_POINT ( 'NONE',  ( 28.89564796280000181, -73.80968813319999811, -26.61317346570000097 ) ) ;
#22012=EDGE_CURVE ( 'NONE', #22934, #12631, #1265, .T. ) ;
#22022=DIRECTION ( 'NONE',  ( 1.000000000000000000, 0.000000000000000000, 0.000000000000000000 ) ) ;
#22023=CARTESIAN_POINT ( 'NONE',  ( 23.66743934140000150, -49.85663837279999910, 0.8718307226189999648 ) ) ;
#22024=CARTESIAN_POINT ( 'NONE',  ( 26.26491651929999804, -69.97113394359999461, 10.80126583880000091 ) ) ;
#22025=CARTESIAN_POINT ( 'NONE',  ( 39.31656870519286429, -73.61799623138361426, 7.217717631475800033 ) ) ;
#22026=VERTEX_POINT ( 'NONE', #2627 ) ;
#22035=CARTESIAN_POINT ( 'NONE',  ( 23.80490084257870720, -74.13827441015507702, -31.01263663817537619 ) ) ;
#22036=CARTESIAN_POINT ( 'NONE',  ( -12.07464971489999961, -68.03625990740000873, -24.51877662120000068 ) ) ;
#22037=CARTESIAN_POINT ( 'NONE',  ( 22.00064631549999916, -63.98660223360000288, 11.26240653729999863 ) ) ;
#22038=CARTESIAN_POINT ( 'NONE',  ( -10.91297770669999956, -42.23583340100000072, -21.40387953429999968 ) ) ;
#22040=CARTESIAN_POINT ( 'NONE',  ( 23.52622212079999997, -57.40875702419999982, -9.564509902230000193 ) ) ;
#22041=CARTESIAN_POINT ( 'NONE',  ( -11.45174557199970522, -57.47815920938258216, 20.36405547779946090 ) ) ;
#22043=EDGE_CURVE ( 'NONE', #21377, #26756, #14094, .T. ) ;
#22049=AXIS2_PLACEMENT_3D ( 'NONE', #13964, #11012, #19927 ) ;
#22055=CARTESIAN_POINT ( 'NONE',  ( 27.19724826568005227, -72.11187000725442431, -11.65709713041382578 ) ) ;
#22058=CARTESIAN_POINT ( 'NONE',  ( 8.125022609680000230, -36.17810633829999745, -21.26282345639999605 ) ) ;
#22062=CARTESIAN_POINT ( 'NONE',  ( 23.09686208289999954, -18.86159979430000178, 1.490590284119999831 ) ) ;
#22068=DIRECTION ( 'NONE',  ( 1.000000000000000000, 0.000000000000000000, 0.000000000000000000 ) ) ;
#22070=CARTESIAN_POINT ( 'NONE',  ( 10.20110288159999890, -82.25000000000000000, 41.00000000000000000 ) ) ;
#22072=CIRCLE ( 'NONE', #16484, 7.249999999999999112 ) ;
#22075=ORIENTED_EDGE ( 'NONE', *, *, #2333, .F. ) ;
#22076=CARTESIAN_POINT ( 'NONE',  ( 8.697936417900001160, -18.86343732329999767, -19.75624699629999981 ) ) ;
#22077=CIRCLE ( 'NONE', #23032, 10.00000000000000000 ) ;
#22079=CARTESIAN_POINT ( 'NONE',  ( 21.93668104079999992, -36.18298320059999895, -10.15270841880000141 ) ) ;
#22080=EDGE_CURVE ( 'NONE', #18106, #28649, #8497, .T. ) ;
#22081=CARTESIAN_POINT ( 'NONE',  ( -12.57842660070000029, -63.53964550370000097, 21.17786332950000272 ) ) ;
#22082=CIRCLE ( 'NONE', #5333, 6.750000000000000000 ) ;
#22083=CARTESIAN_POINT ( 'NONE',  ( 9.504972818060000606, -36.53320237809999327, -21.93059852529999887 ) ) ;
#22084=DIRECTION ( 'NONE',  ( 0.03516156865429550388, 0.000000000000000000, 0.9993816408608722224 ) ) ;
#22085=CARTESIAN_POINT ( 'NONE',  ( -19.49041480450000208, -52.62618816520016196, 12.93508487010000785 ) ) ;
#22089=CARTESIAN_POINT ( 'NONE',  ( 21.53806856769999811, -36.56992524600000394, -6.948750440460000455 ) ) ;
#22090=CARTESIAN_POINT ( 'NONE',  ( -40.70731707320000226, -74.50000000000000000, -7.215414233289999757 ) ) ;
#22094=CARTESIAN_POINT ( 'NONE',  ( -14.24339565470000224, -80.06075086779999594, 36.77521474840000337 ) ) ;
#22095=CARTESIAN_POINT ( 'NONE',  ( -9.824387680670000123, -18.50000000000000000, -22.02292149959999890 ) ) ;
#22096=DIRECTION ( 'NONE',  ( 0.000000000000000000, 1.000000000000000000, 0.000000000000000000 ) ) ;
#22097=CARTESIAN_POINT ( 'NONE',  ( -13.94900084250000027, -74.00000000000000000, 36.21247097760000599 ) ) ;
#22098=CARTESIAN_POINT ( 'NONE',  ( -32.74642262723747876, -79.90759221510043631, -22.43672242427770769 ) ) ;
#22102=AXIS2_PLACEMENT_3D ( 'NONE', #24214, #17368, #10773 ) ;
#22106=CARTESIAN_POINT ( 'NONE',  ( -7.173755656178061102, -73.51389412123563716, 38.94432755061352225 ) ) ;
#22107=CARTESIAN_POINT ( 'NONE',  ( -40.70731707320000226, -74.50000000000000000, -7.215414233289999757 ) ) ;
#22110=CARTESIAN_POINT ( 'NONE',  ( -32.17538889770000310, -74.02659082439998883, -21.91468059299999993 ) ) ;
#22111=CARTESIAN_POINT ( 'NONE',  ( -22.71848792900000191, -80.00000000000000000, -32.61798286559999838 ) ) ;
#22112=ORIENTED_EDGE ( 'NONE', *, *, #26572, .F. ) ;
#22115=CARTESIAN_POINT ( 'NONE',  ( 7.105427357599999217E-15, -69.00000000000000000, -40.00000000000000000 ) ) ;
#22117=CARTESIAN_POINT ( 'NONE',  ( -0.5459402786740000790, -58.79569603810000444, -23.43709083150000083 ) ) ;
#22118=EDGE_LOOP ( 'NONE', ( #10859, #68, #1291, #7981 ) ) ;
#22119=CARTESIAN_POINT ( 'NONE',  ( 0.000000000000000000, -82.25000000000000000, 40.00000000000000000 ) ) ;
#22120=CARTESIAN_POINT ( 'NONE',  ( 41.00000000000000000, -82.25000000000000000, 10.20110288159999890 ) ) ;
#22126=CARTESIAN_POINT ( 'NONE',  ( -22.09862634569999784, -80.12422039649999306, -32.50322686590000387 ) ) ;
#22128=DIRECTION ( 'NONE',  ( -0.3687499999999814260, 0.000000000000000000, 0.9295286103719527793 ) ) ;
#22137=TOROIDAL_SURFACE ( 'NONE', #17013, 0.5000000000000000000, 0.5000000000000000000 ) ;
#22138=LINE ( 'NONE', #28667, #13404 ) ;
#22139=CARTESIAN_POINT ( 'NONE',  ( 10.16635616659465136, -72.73332183106052184, -26.84588916250481105 ) ) ;
#22142=CARTESIAN_POINT ( 'NONE',  ( 9.438993784957457223, -64.72767717259272047, -23.93801147444352395 ) ) ;
#22143=CARTESIAN_POINT ( 'NONE',  ( 20.33037861331306217, -73.74757277672107136, -31.96328472817131683 ) ) ;
#22146=FACE_OUTER_BOUND ( 'NONE', #22974, .T. ) ;
#22148=CARTESIAN_POINT ( 'NONE',  ( -15.42363691649999957, -45.73899999920000425, 22.84488648889999851 ) ) ;
#22150=ORIENTED_EDGE ( 'NONE', *, *, #19776, .F. ) ;
#22151=DIRECTION ( 'NONE',  ( 0.000000000000000000, 1.000000000000000000, 0.000000000000000000 ) ) ;
#22156=ORIENTED_EDGE ( 'NONE', *, *, #3977, .F. ) ;
#22158=EDGE_LOOP ( 'NONE', ( #6100, #8437, #6460 ) ) ;
#22159=CARTESIAN_POINT ( 'NONE',  ( 22.29272167938353633, -65.04696937986301464, 11.61829170019522017 ) ) ;
#22163=CARTESIAN_POINT ( 'NONE',  ( 47.19378694702872679, -79.33057058301108100, -1.140171656175917647 ) ) ;
#22164=ORIENTED_EDGE ( 'NONE', *, *, #6470, .F. ) ;
#22166=CARTESIAN_POINT ( 'NONE',  ( 24.76695232029999971, -34.59963798460000106, 1.400254471660000055 ) ) ;
#22167=CARTESIAN_POINT ( 'NONE',  ( -14.25482831575127030, -80.47374551902997553, 36.57016602121424143 ) ) ;
#22170=EDGE_LOOP ( 'NONE', ( #6240, #19550, #1556, #817 ) ) ;
#22181=CARTESIAN_POINT ( 'NONE',  ( -12.04115840220000067, -49.87553805839999654, -19.70837320809999937 ) ) ;
#22183=CARTESIAN_POINT ( 'NONE',  ( 22.95932757850121675, -57.43039251884066942, -9.307781678040345952 ) ) ;
#22185=CARTESIAN_POINT ( 'NONE',  ( -2.987826573587363477, -18.62337006874621181, -24.35058480141394099 ) ) ;
#22190=CARTESIAN_POINT ( 'NONE',  ( 22.71753027169577521, -19.47230399480618246, 1.004254908788112965 ) ) ;
#22192=EDGE_LOOP ( 'NONE', ( #24388, #9734, #17804, #26274, #25232, #14406 ) ) ;
#22193=CARTESIAN_POINT ( 'NONE',  ( -16.49390888960000368, -80.00000000000000000, 44.28897684009999836 ) ) ;
#22196=CARTESIAN_POINT ( 'NONE',  ( 7.642421028099999347, -37.32903481230000153, -21.50491099470000123 ) ) ;
#22199=CARTESIAN_POINT ( 'NONE',  ( 22.02376134869999902, -19.15747282889999781, -0.1818244595100000083 ) ) ;
#22206=EDGE_CURVE ( 'NONE', #19169, #12443, #18590, .T. ) ;
#22209=CARTESIAN_POINT ( 'NONE',  ( -12.68184371739999960, -66.93519943800001215, -22.70010485369999742 ) ) ;
#22213=ADVANCED_FACE ( 'NONE', ( #6660 ), #12214, .T. ) ;
#22214=CARTESIAN_POINT ( 'NONE',  ( -10.17458377400000025, -18.50000000000000000, -22.50859265919999785 ) ) ;
#22218=CARTESIAN_POINT ( 'NONE',  ( -14.55867151890000066, -64.24504444460001196, 22.15151624130000130 ) ) ;
#22219=CARTESIAN_POINT ( 'NONE',  ( 0.000000000000000000, -72.82938648530000592, 0.000000000000000000 ) ) ;
#22221=CARTESIAN_POINT ( 'NONE',  ( -20.53532388389999852, -56.19735282230000450, 14.83773643259999986 ) ) ;
#22222=ORIENTED_EDGE ( 'NONE', *, *, #17062, .T. ) ;
#22224=CARTESIAN_POINT ( 'NONE',  ( 29.28697822896142711, -74.32957653769940976, -26.08612603725635992 ) ) ;
#22225=DIRECTION ( 'NONE',  ( 1.000000000000000000, 0.000000000000000000, 0.000000000000000000 ) ) ;
#22230=CARTESIAN_POINT ( 'NONE',  ( 19.36777041659999554, -19.46363745430000236, 10.50577160559999967 ) ) ;
#22231=EDGE_CURVE ( 'NONE', #9894, #18698, #22690, .T. ) ;
#22235=AXIS2_PLACEMENT_3D ( 'NONE', #5526, #25907, #3623 ) ;
#22236=CARTESIAN_POINT ( 'NONE',  ( 21.31224117700000065, -62.89055566329999891, 11.58369406600000140 ) ) ;
#22239=ORIENTED_EDGE ( 'NONE', *, *, #13271, .T. ) ;
#22240=CARTESIAN_POINT ( 'NONE',  ( 40.00000000000000000, -79.00000000000000000, 4.898587196589999938E-15 ) ) ;
#22242=CARTESIAN_POINT ( 'NONE',  ( 21.42283722234454046, -19.48260761094563520, 9.476082331836883199 ) ) ;
#22243=CARTESIAN_POINT ( 'NONE',  ( -40.34091732139999920, -74.29300278850000439, -7.252014196680000246 ) ) ;
#22248=CARTESIAN_POINT ( 'NONE',  ( -32.52011734909999774, -74.20254482470001278, -21.99161358219999940 ) ) ;
#22256=DIRECTION ( 'NONE',  ( 0.000000000000000000, 1.000000000000000000, 0.000000000000000000 ) ) ;
#22258=CARTESIAN_POINT ( 'NONE',  ( -23.10281210965324306, -72.22683319543493496, 16.53369850595768753 ) ) ;
#22260=DIRECTION ( 'NONE',  ( 0.000000000000000000, 1.000000000000000000, 0.000000000000000000 ) ) ;
#22261=ORIENTED_EDGE ( 'NONE', *, *, #26819, .F. ) ;
#22262=CARTESIAN_POINT ( 'NONE',  ( -36.59277592640000165, -77.00000000000000000, -27.40038777100000189 ) ) ;
#22263=CARTESIAN_POINT ( 'NONE',  ( -21.85457011909999991, -79.72846757719999289, -32.66023316209999905 ) ) ;
#22264=CARTESIAN_POINT ( 'NONE',  ( 20.64374438969968040, -57.47815920198944895, 10.93952083479982740 ) ) ;
#22265=CARTESIAN_POINT ( 'NONE',  ( 8.702650270779999531, -36.72157724030000026, -21.61812616270000120 ) ) ;
#22270=EDGE_CURVE ( 'NONE', #21377, #19473, #12969, .T. ) ;
#22271=CARTESIAN_POINT ( 'NONE',  ( -2.785765053610000042, -64.19655116939999573, -26.34478359919999946 ) ) ;
#22272=CARTESIAN_POINT ( 'NONE',  ( -39.54176628510000313, -73.97626148509999666, 7.314390784519999578 ) ) ;
#22273=CARTESIAN_POINT ( 'NONE',  ( -22.07235328799999863, -74.12815218200000800, -32.48152077880000377 ) ) ;
#22276=CARTESIAN_POINT ( 'NONE',  ( -7.307162633536313123, -73.99981221269277398, 39.53460932750543577 ) ) ;
#22277=CARTESIAN_POINT ( 'NONE',  ( 7.215414233289999757, -74.50000000000000000, -40.70731707320000226 ) ) ;
#22278=ORIENTED_EDGE ( 'NONE', *, *, #10054, .T. ) ;
#22283=CARTESIAN_POINT ( 'NONE',  ( 20.35242036615802519, -74.00000000000477485, -32.70839735534965342 ) ) ;
#22284=CARTESIAN_POINT ( 'NONE',  ( 2.486899575159999765E-14, -80.50000000000000000, 7.105427357599999217E-15 ) ) ;
#22286=CARTESIAN_POINT ( 'NONE',  ( 0.000000000000000000, -82.25000000000000000, 0.000000000000000000 ) ) ;
#22288=DIRECTION ( 'NONE',  ( 1.000000000000000000, 0.000000000000000000, 0.000000000000000000 ) ) ;
#22296=CARTESIAN_POINT ( 'NONE',  ( -21.89190459030000113, -74.01117791779999777, -32.13651045809999829 ) ) ;
#22302=CARTESIAN_POINT ( 'NONE',  ( 22.17953377930000158, -65.07443093669999712, 11.85657293289999892 ) ) ;
#22306=CARTESIAN_POINT ( 'NONE',  ( -10.78318709900000094, -19.46528100780000159, -19.40120878459999787 ) ) ;
#22307=CARTESIAN_POINT ( 'NONE',  ( 47.19667865516128558, -79.32224956671613825, -1.110774814387318177 ) ) ;
#22309=CARTESIAN_POINT ( 'NONE',  ( 1.065814103639999922E-14, -18.50000000000000000, 2.664535259099999805E-15 ) ) ;
#22310=EDGE_CURVE ( 'NONE', #1175, #3141, #10753, .T. ) ;
#22312=CARTESIAN_POINT ( 'NONE',  ( -32.63800352850000053, -74.22019266179999875, -21.66201587429999975 ) ) ;
#22313=ORIENTED_EDGE ( 'NONE', *, *, #3572, .T. ) ;
#22315=CARTESIAN_POINT ( 'NONE',  ( 7.400235822239999983, -63.19606248799999548, -23.19730672580000075 ) ) ;
#22316=VERTEX_POINT ( 'NONE', #26548 ) ;
#22317=ADVANCED_FACE ( 'NONE', ( #12828 ), #27816, .T. ) ;
#22318=CARTESIAN_POINT ( 'NONE',  ( 27.20825738430000129, -68.79186515250000866, 1.585888911440000104 ) ) ;
#22320=CARTESIAN_POINT ( 'NONE',  ( 20.86991714526983088, -74.00000000000196110, -32.73119363184984110 ) ) ;
#22321=CARTESIAN_POINT ( 'NONE',  ( -20.08103059739376306, -57.43018248828013128, 14.46712379734940335 ) ) ;
#22323=CIRCLE ( 'NONE', #6020, 11.00000000000000000 ) ;
#22325=CARTESIAN_POINT ( 'NONE',  ( 22.71963930830125022, -57.44066855174124697, -9.099147364980348485 ) ) ;
#22340=CARTESIAN_POINT ( 'NONE',  ( 27.06175282578147190, -72.22552502750772874, -11.46356654631565597 ) ) ;
#22343=CARTESIAN_POINT ( 'NONE',  ( 7.836612423160000063, -37.59151559440000057, -21.54406958319999887 ) ) ;
#22344=EDGE_CURVE ( 'NONE', #28514, #15872, #9544, .T. ) ;
#22345=AXIS2_PLACEMENT_3D ( 'NONE', #414, #15669, #4467 ) ;
#22346=CARTESIAN_POINT ( 'NONE',  ( 9.024081099289999131, -19.49999992740000110, -18.94592230980000380 ) ) ;
#22347=EDGE_LOOP ( 'NONE', ( #5868, #13698, #19248, #470 ) ) ;
#22348=CIRCLE ( 'NONE', #18142, 0.5000000000000004441 ) ;
#22349=FACE_OUTER_BOUND ( 'NONE', #12427, .T. ) ;
#22356=CARTESIAN_POINT ( 'NONE',  ( 7.066909182079999852, -57.47855601759999900, -22.26662627820000040 ) ) ;
#22358=CARTESIAN_POINT ( 'NONE',  ( -13.05632738709999963, -66.36684605099999601, -22.18172164889999820 ) ) ;
#22360=DIRECTION ( 'NONE',  ( 1.000000000000000000, 0.000000000000000000, 0.000000000000000000 ) ) ;
#22361=FACE_OUTER_BOUND ( 'NONE', #18016, .T. ) ;
#22365=TOROIDAL_SURFACE ( 'NONE', #6051, 7.750000000000000000, 0.5000000000000000000 ) ;
#22366=ORIENTED_EDGE ( 'NONE', *, *, #28364, .F. ) ;
#22367=AXIS2_PLACEMENT_3D ( 'NONE', #6766, #21764, #6456 ) ;
#22370=CARTESIAN_POINT ( 'NONE',  ( -40.00000000000000000, -73.50000000000000000, 3.397282455350000038E-15 ) ) ;
#22372=EDGE_CURVE ( 'NONE', #3493, #21366, #13079, .T. ) ;
#22374=EDGE_CURVE ( 'NONE', #21778, #24612, #16191, .T. ) ;
#22375=CARTESIAN_POINT ( 'NONE',  ( -11.22008280823478010, -57.43018266902328861, -22.06025754104976855 ) ) ;
#22376=EDGE_LOOP ( 'NONE', ( #26137, #8031, #10704 ) ) ;
#22378=CARTESIAN_POINT ( 'NONE',  ( 7.627567457969999687, -74.00000025069999765, -38.62788781560000473 ) ) ;
#22379=VERTEX_POINT ( 'NONE', #15748 ) ;
#22380=EDGE_CURVE ( 'NONE', #6342, #15463, #4326, .T. ) ;
#22382=EDGE_CURVE ( 'NONE', #13629, #25229, #16836, .T. ) ;
#22383=CARTESIAN_POINT ( 'NONE',  ( 23.03829042120000281, -52.56313962710000709, 10.32398954119999956 ) ) ;
#22384=CARTESIAN_POINT ( 'NONE',  ( -12.09704001540000107, -80.00000000000000000, 47.10905722069999513 ) ) ;
#22385=CARTESIAN_POINT ( 'NONE',  ( 22.20719543259999895, -26.03958238319999907, 9.782350785770001167 ) ) ;
#22390=CARTESIAN_POINT ( 'NONE',  ( 21.68405932330000141, -63.95915174670000169, 11.72027971770000043 ) ) ;
#22393=ORIENTED_EDGE ( 'NONE', *, *, #19822, .F. ) ;
#22399=DIRECTION ( 'NONE',  ( 1.000000000000000000, 0.000000000000000000, 0.000000000000000000 ) ) ;
#22400=CARTESIAN_POINT ( 'NONE',  ( 23.44995121140226857, -63.81246114131585045, -7.514631542302712575 ) ) ;
#22401=ORIENTED_EDGE ( 'NONE', *, *, #24510, .T. ) ;
#22405=CARTESIAN_POINT ( 'NONE',  ( 25.13293939673078370, -49.51244866357122021, 1.380189421151490459 ) ) ;
#22406=TOROIDAL_SURFACE ( 'NONE', #18211, 38.75000000000000000, 0.5000000000000000000 ) ;
#22412=VERTEX_POINT ( 'NONE', #9494 ) ;
#22413=CARTESIAN_POINT ( 'NONE',  ( -23.16986609970000188, -72.82938648530000592, 16.90925194980000157 ) ) ;
#22418=CARTESIAN_POINT ( 'NONE',  ( -22.21526612139999912, -80.34842048189999275, -32.35915136539999537 ) ) ;
#22420=CARTESIAN_POINT ( 'NONE',  ( -3.689713002109519024, -69.66052405845533713, -28.05308719045783405 ) ) ;
#22424=ORIENTED_EDGE ( 'NONE', *, *, #663, .F. ) ;
#22427=CARTESIAN_POINT ( 'NONE',  ( -2.585646220079999669, -58.19955242929999883, -25.25977730230000162 ) ) ;
#22428=CARTESIAN_POINT ( 'NONE',  ( -40.32201634399999790, -74.31845592130000000, 7.253647055850000136 ) ) ;
#22429=CARTESIAN_POINT ( 'NONE',  ( -22.22906645670000003, -74.39508596250000494, -32.83566817450000030 ) ) ;
#22430=AXIS2_PLACEMENT_3D ( 'NONE', #1161, #6048, #12742 ) ;
#22432=LINE ( 'NONE', #13372, #4583 ) ;
#22434=CARTESIAN_POINT ( 'NONE',  ( -7.494372175572003414, -73.99988466611407034, 38.93864016370615388 ) ) ;
#22435=CARTESIAN_POINT ( 'NONE',  ( -17.93028678539999987, -18.50000000000000000, 10.99759328500000066 ) ) ;
#22436=ORIENTED_EDGE ( 'NONE', *, *, #834, .T. ) ;
#22440=DIRECTION ( 'NONE',  ( 0.9993816408608721114, 0.000000000000000000, -0.03516156865429537204 ) ) ;
#22441=CARTESIAN_POINT ( 'NONE',  ( 22.14137210370000020, -52.59522851920000619, 10.05377507689999916 ) ) ;
#22442=B_SPLINE_SURFACE_WITH_KNOTS ( 'NONE', 5, 5, ( 
 ( #23216, #9795, #23497, #18558, #5299, #12392, #1355, #18849, #14186 ),
 ( #23082, #7772, #27603, #23354, #3397, #7642, #3265, #12118, #1094 ),
 ( #27736, #16644, #21173, #21441, #28560, #1917, #2065, #21582, #8596 ),
 ( #1502, #28691, #10760, #5982, #19529, #24046, #3809, #14729, #17063 ),
 ( #17206, #17353, #6271, #14862, #12672, #19390, #8304, #26094, #6123 ),
 ( #26384, #19812, #28143, #10342, #24199, #23766, #28414, #19672, #28270 ) ),
 .UNSPECIFIED., .F., .F., .F.,
 ( 6, 6 ),
 ( 6, 3, 6 ),
 ( 36.59856967580000031, 66.18347591719999912 ),
 ( 0.000000000000000000, 1.000000000000000000, 2.000000000000000000 ),
 .UNSPECIFIED. ) ;
#22445=CARTESIAN_POINT ( 'NONE',  ( -12.17175179449999867, -57.47855601710000428, -19.93971688569999756 ) ) ;
#22446=ORIENTED_EDGE ( 'NONE', *, *, #20855, .F. ) ;
#22448=CONICAL_SURFACE ( 'NONE', #26166, 25.14975229270001833, 0.4276056667390000787 ) ;
#22451=CARTESIAN_POINT ( 'NONE',  ( -10.92291579689999992, -42.27245207490000212, 20.04758140150000045 ) ) ;
#22452=DIRECTION ( 'NONE',  ( 1.000000000000000000, 0.000000000000000000, 0.000000000000000000 ) ) ;
#22461=CARTESIAN_POINT ( 'NONE',  ( 26.84355216712550174, -67.87586260162430563, 1.442230305706864169 ) ) ;
#22462=CARTESIAN_POINT ( 'NONE',  ( 21.60334004033046895, -37.79333402771170825, -8.049301293328291251 ) ) ;
#22463=ORIENTED_EDGE ( 'NONE', *, *, #26829, .T. ) ;
#22467=VERTEX_POINT ( 'NONE', #20736 ) ;
#22473=ADVANCED_FACE ( 'NONE', ( #6741 ), #23402, .T. ) ;
#22474=AXIS2_PLACEMENT_3D ( 'NONE', #11421, #18144, #7373 ) ;
#22477=CARTESIAN_POINT ( 'NONE',  ( 7.084351940260000369, -59.04260968250000019, -22.31839619009999964 ) ) ;
#22479=CARTESIAN_POINT ( 'NONE',  ( -10.76543513999999924, -34.63364287790000162, -21.24130719339999729 ) ) ;
#22481=CARTESIAN_POINT ( 'NONE',  ( 27.98858332410410199, -71.34444037274488437, 1.047634458806025126 ) ) ;
#22482=ORIENTED_EDGE ( 'NONE', *, *, #1951, .T. ) ;
#22487=DIRECTION ( 'NONE',  ( 1.000000000000000000, 0.000000000000000000, 0.000000000000000000 ) ) ;
#22489=CARTESIAN_POINT ( 'NONE',  ( 7.562763921490000207, -74.00035141509999903, 39.03055149349999908 ) ) ;
#22490=DIRECTION ( 'NONE',  ( 0.000000000000000000, 1.000000000000000000, 0.000000000000000000 ) ) ;
#22493=CARTESIAN_POINT ( 'NONE',  ( 22.98461340545973641, -19.47630996313253959, 1.205578334398293538 ) ) ;
#22496=CARTESIAN_POINT ( 'NONE',  ( 27.03314449209916859, -72.25218846125086714, -11.41478320253755818 ) ) ;
#22497=CARTESIAN_POINT ( 'NONE',  ( -20.58900368409999970, -58.81362829640000456, 14.87320149399999991 ) ) ;
#22498=CARTESIAN_POINT ( 'NONE',  ( 8.339202836120000129, -36.74552967150000171, -21.40376449809999926 ) ) ;
#22500=CARTESIAN_POINT ( 'NONE',  ( 21.56299924104185095, -36.38197226018986896, -6.848569379388298906 ) ) ;
#22502=CARTESIAN_POINT ( 'NONE',  ( -10.00000000000000000, -42.50000000000000000, 1.224606353819999829E-15 ) ) ;
#22503=CARTESIAN_POINT ( 'NONE',  ( -12.86681839629088131, -19.48210950177368517, 19.53479179472106608 ) ) ;
#22504=CARTESIAN_POINT ( 'NONE',  ( -7.325370793560000315, -45.73899999920000425, -24.94672208400000102 ) ) ;
#22505=DIRECTION ( 'NONE',  ( 0.000000000000000000, -1.000000000000000000, 0.000000000000000000 ) ) ;
#22506=ORIENTED_EDGE ( 'NONE', *, *, #2685, .F. ) ;
#22507=DIRECTION ( 'NONE',  ( 1.000000000000000000, 0.000000000000000000, 0.000000000000000000 ) ) ;
#22508=CARTESIAN_POINT ( 'NONE',  ( -13.81324249570000084, -18.62337005500000231, 20.27492115300000108 ) ) ;
#22511=EDGE_CURVE ( 'NONE', #2951, #6426, #14966, .T. ) ;
#22514=DIRECTION ( 'NONE',  ( 1.000000000000000000, 0.000000000000000000, 0.000000000000000000 ) ) ;
#22516=EDGE_LOOP ( 'NONE', ( #17459, #20229, #11158, #6059 ) ) ;
#22519=ADVANCED_FACE ( 'NONE', ( #8162 ), #28027, .T. ) ;
#22520=CIRCLE ( 'NONE', #24843, 3.750000000000000000 ) ;
#22521=ORIENTED_EDGE ( 'NONE', *, *, #10852, .F. ) ;
#22522=CARTESIAN_POINT ( 'NONE',  ( -12.88897289979999883, -65.65850715019999484, 21.91133662320000042 ) ) ;
#22523=CARTESIAN_POINT ( 'NONE',  ( -13.57564758800000071, -60.33093763760000172, 20.91920646410000018 ) ) ;
#22524=CARTESIAN_POINT ( 'NONE',  ( -38.08875739639999836, -84.00000000000000000, 9.476764215410000247 ) ) ;
#22527=DIRECTION ( 'NONE',  ( -0.9993816408608721114, 0.000000000000000000, 0.03516156865429537204 ) ) ;
#22529=CARTESIAN_POINT ( 'NONE',  ( 19.97062749839314577, -19.47948121987873193, -8.623729410243210936 ) ) ;
#22531=ORIENTED_EDGE ( 'NONE', *, *, #1109, .T. ) ;
#22532=CARTESIAN_POINT ( 'NONE',  ( -7.215414233289999757, -74.50000000000000000, -40.70731707320000226 ) ) ;
#22536=CARTESIAN_POINT ( 'NONE',  ( 23.10863584609999677, -55.79355142130000900, 10.36080582650000004 ) ) ;
#22539=CARTESIAN_POINT ( 'NONE',  ( -11.81899278133277775, -64.69849623153378104, -22.71259346144224978 ) ) ;
#22540=CIRCLE ( 'NONE', #19726, 7.250000000000000000 ) ;
#22543=CARTESIAN_POINT ( 'NONE',  ( 22.17953377930000158, -65.07443093669999712, 11.85657293289999892 ) ) ;
#22551=CARTESIAN_POINT ( 'NONE',  ( -39.85902549739999756, -74.23956954080000514, -7.332363419530000037 ) ) ;
#22557=EDGE_CURVE ( 'NONE', #8623, #7572, #24138, .T. ) ;
#22564=AXIS2_PLACEMENT_3D ( 'NONE', #22115, #2156, #20210 ) ;
#22565=ORIENTED_EDGE ( 'NONE', *, *, #9575, .T. ) ;
#22566=CARTESIAN_POINT ( 'NONE',  ( -22.94912671726251219, -71.22806229626020524, 15.96158107121579661 ) ) ;
#22568=CARTESIAN_POINT ( 'NONE',  ( 47.09015203950000483, -74.29080663029999698, -1.541671319510000027 ) ) ;
#22569=ORIENTED_EDGE ( 'NONE', *, *, #22750, .T. ) ;
#22570=CARTESIAN_POINT ( 'NONE',  ( 7.152485405711615840, -73.50000015768027595, -38.81101221961867509 ) ) ;
#22571=CARTESIAN_POINT ( 'NONE',  ( -21.70609662629999903, -80.13404657770000483, -32.70204620079999813 ) ) ;
#22572=CARTESIAN_POINT ( 'NONE',  ( -3.058911230670000148, -72.82938648530000592, -28.52031834779999997 ) ) ;
#22576=CARTESIAN_POINT ( 'NONE',  ( -32.25000000000000000, -74.00000000000000000, 2.464695114664749584E-15 ) ) ;
#22578=CARTESIAN_POINT ( 'NONE',  ( -39.49475000900000765, -74.05254684259999465, 7.367397733549999828 ) ) ;
#22579=CARTESIAN_POINT ( 'NONE',  ( -21.87483401080000078, -74.28769487450000497, -32.59760389210000397 ) ) ;
#22582=CARTESIAN_POINT ( 'NONE',  ( -7.396579754587796707, -73.99963493658084701, 39.20624479181404354 ) ) ;
#22583=CARTESIAN_POINT ( 'NONE',  ( -18.43157295690000197, -18.85467989400000022, 11.82421860260000024 ) ) ;
#22584=ORIENTED_EDGE ( 'NONE', *, *, #20581, .F. ) ;
#22588=CARTESIAN_POINT ( 'NONE',  ( 22.64274859190000200, -63.79833278959999632, 10.75909410010000045 ) ) ;
#22589=CARTESIAN_POINT ( 'NONE',  ( 8.798272373610000585, -34.78948601350000303, -20.39306157709999923 ) ) ;
#22592=VERTEX_POINT ( 'NONE', #28674 ) ;
#22593=CARTESIAN_POINT ( 'NONE',  ( -14.93121078260000090, -79.49999975080000070, 36.29905569799999654 ) ) ;
#22594=EDGE_CURVE ( 'NONE', #20759, #15974, #24785, .T. ) ;
#22595=DIRECTION ( 'NONE',  ( 0.000000000000000000, -1.000000000000000000, 0.000000000000000000 ) ) ;
#22598=DIRECTION ( 'NONE',  ( 1.000000000000000000, 0.000000000000000000, 0.000000000000000000 ) ) ;
#22599=CARTESIAN_POINT ( 'NONE',  ( 46.99997450946052169, -74.14530279077403918, -1.887577394871021719 ) ) ;
#22600=ORIENTED_EDGE ( 'NONE', *, *, #11403, .T. ) ;
#22601=DIRECTION ( 'NONE',  ( 1.000000000000000000, 0.000000000000000000, 0.000000000000000000 ) ) ;
#22602=CARTESIAN_POINT ( 'NONE',  ( 2.042810365310000056E-12, -74.50000000000000000, -2.458477865729999957E-12 ) ) ;
#22607=DIRECTION ( 'NONE',  ( 1.000000000000000000, 0.000000000000000000, 0.000000000000000000 ) ) ;
#22610=CARTESIAN_POINT ( 'NONE',  ( -10.20110288159999890, -82.25000000000000000, -41.00000000000000000 ) ) ;
#22611=ORIENTED_EDGE ( 'NONE', *, *, #24757, .T. ) ;
#22615=VERTEX_POINT ( 'NONE', #17624 ) ;
#22622=CARTESIAN_POINT ( 'NONE',  ( -18.44190124780000062, -19.46163090479999980, 12.50665444260000037 ) ) ;
#22624=CARTESIAN_POINT ( 'NONE',  ( 31.51289799120000268, -73.45782179829998881, -20.31705881479999931 ) ) ;
#22626=EDGE_CURVE ( 'NONE', #23505, #23386, #10893, .T. ) ;
#22629=ORIENTED_EDGE ( 'NONE', *, *, #25993, .F. ) ;
#22630=CARTESIAN_POINT ( 'NONE',  ( 10.07773541299999920, -36.00000000000000000, -20.87139911950000126 ) ) ;
#22633=CARTESIAN_POINT ( 'NONE',  ( 0.000000000000000000, -82.50000000000000000, 0.000000000000000000 ) ) ;
#22636=CARTESIAN_POINT ( 'NONE',  ( 36.59060436630000623, -79.00000000000000000, -14.75000000000000000 ) ) ;
#22638=CARTESIAN_POINT ( 'NONE',  ( 24.20787553755564048, -19.49659809026794832, 1.495029698088813142 ) ) ;
#22640=CARTESIAN_POINT ( 'NONE',  ( 26.84513186441053989, -72.48886963431783670, -10.90665099628932388 ) ) ;
#22642=CARTESIAN_POINT ( 'NONE',  ( 8.367124212330001143, -37.94838740809999678, -21.73111097249999801 ) ) ;
#22643=CARTESIAN_POINT ( 'NONE',  ( 8.607817759397720536, -19.47905375331706423, -19.99126106825392313 ) ) ;
#22647=DIRECTION ( 'NONE',  ( 0.000000000000000000, -1.000000000000000000, 0.000000000000000000 ) ) ;
#22648=CARTESIAN_POINT ( 'NONE',  ( -14.65665286289999969, -74.50000000000000000, 36.94583910070000599 ) ) ;
#22649=B_SPLINE_CURVE_WITH_KNOTS ( 'NONE', 3,
 ( #8145, #19361, #1734, #10574, #14827, #3775 ),
 .UNSPECIFIED., .F., .F.,
 ( 4, 2, 4 ),
 ( 0.000000000000000000, 0.5000000000000000000, 1.000000000000000000 ),
 .UNSPECIFIED. ) ;
#22651=CARTESIAN_POINT ( 'NONE',  ( -0.5256375577959999656, -45.99906616869999709, -22.95427111080000060 ) ) ;
#22653=ADVANCED_FACE ( 'NONE', ( #9867 ), #14544, .T. ) ;
#22654=EDGE_CURVE ( 'NONE', #14960, #9596, #27038, .T. ) ;
#22655=CARTESIAN_POINT ( 'NONE',  ( 23.50753042992814557, -19.50000000000000000, 9.440918867846139761 ) ) ;
#22659=DIRECTION ( 'NONE',  ( -0.02411449919422837401, -0.9975499440283625008, 0.06567038980866957143 ) ) ;
#22661=CARTESIAN_POINT ( 'NONE',  ( 36.36887021859999436, -74.91502851379999584, -14.85406864730000009 ) ) ;
#22663=CARTESIAN_POINT ( 'NONE',  ( -12.08447405829999965, -59.01570696489999790, 20.27932901980000224 ) ) ;
#22667=CARTESIAN_POINT ( 'NONE',  ( -12.07243358760000085, -67.46050599719998786, -24.77970463289999969 ) ) ;
#22668=EDGE_CURVE ( 'NONE', #19973, #5424, #6619, .T. ) ;
#22674=ORIENTED_EDGE ( 'NONE', *, *, #234, .T. ) ;
#22676=ORIENTED_EDGE ( 'NONE', *, *, #3572, .F. ) ;
#22677=CARTESIAN_POINT ( 'NONE',  ( -40.70731707320000226, -82.25000000000000000, -7.215414233289999757 ) ) ;
#22681=CARTESIAN_POINT ( 'NONE',  ( 19.02936265269999794, -18.61794786970000359, 10.32221580289999885 ) ) ;
#22682=CARTESIAN_POINT ( 'NONE',  ( 11.81986579350000000, -72.00000321289999761, -27.35691362350000233 ) ) ;
#22686=CARTESIAN_POINT ( 'NONE',  ( -12.41137697900000170, -71.49590739120000649, -25.29708909809999895 ) ) ;
#22689=CARTESIAN_POINT ( 'NONE',  ( 22.05314188356497596, -19.49371746077434153, 9.682146897022342102 ) ) ;
#22690=LINE ( 'NONE', #16808, #2428 ) ;
#22691=ORIENTED_EDGE ( 'NONE', *, *, #7763, .F. ) ;
#22692=AXIS2_PLACEMENT_3D ( 'NONE', #5576, #16062, #1226 ) ;
#22693=DIRECTION ( 'NONE',  ( -0.7071067811865474617, 0.000000000000000000, 0.7071067811865474617 ) ) ;
#22694=ORIENTED_EDGE ( 'NONE', *, *, #25039, .T. ) ;
#22697=TOROIDAL_SURFACE ( 'NONE', #19880, 3.500000000000000000, 0.5000000000000000000 ) ;
#22698=CARTESIAN_POINT ( 'NONE',  ( 11.01541626710000088, -36.00000000000000000, -22.51853742030000305 ) ) ;
#22701=VERTEX_POINT ( 'NONE', #22524 ) ;
#22702=EDGE_CURVE ( 'NONE', #7043, #19884, #7113, .T. ) ;
#22703=CARTESIAN_POINT ( 'NONE',  ( -19.73459501710000197, -19.50000000000000000, 14.41863426819999994 ) ) ;
#22704=EDGE_LOOP ( 'NONE', ( #8720, #8372, #11530, #24734, #4620 ) ) ;
#22705=CARTESIAN_POINT ( 'NONE',  ( -22.51871667277407241, -69.15146719725277080, 14.91063228687463749 ) ) ;
#22706=DIRECTION ( 'NONE',  ( 0.000000000000000000, -1.000000000000000000, 0.000000000000000000 ) ) ;
#22707=CARTESIAN_POINT ( 'NONE',  ( 47.03035266999999919, -74.24775846059999651, -1.795655436139999894 ) ) ;
#22708=ORIENTED_EDGE ( 'NONE', *, *, #16271, .F. ) ;
#22709=CARTESIAN_POINT ( 'NONE',  ( 7.232334316196594948, -73.68677077063769332, -39.48689401865327397 ) ) ;
#22711=EDGE_CURVE ( 'NONE', #15706, #27953, #11254, .T. ) ;
#22712=AXIS2_PLACEMENT_3D ( 'NONE', #12560, #14218, #19379 ) ;
#22714=CARTESIAN_POINT ( 'NONE',  ( 9.028475982079999795, -35.72979163269999958, -19.84586683699999909 ) ) ;
#22715=ADVANCED_FACE ( 'NONE', ( #18292 ), #27121, .T. ) ;
#22717=DIRECTION ( 'NONE',  ( 0.000000000000000000, 1.000000000000000000, 0.000000000000000000 ) ) ;
#22718=EDGE_LOOP ( 'NONE', ( #16776, #246, #580 ) ) ;
#22721=CARTESIAN_POINT ( 'NONE',  ( 25.14695223519999701, -65.07442822920000935, -0.3759466136490000054 ) ) ;
#22722=CARTESIAN_POINT ( 'NONE',  ( -22.19594408369999528, -74.22385006870000268, -32.69771557190000522 ) ) ;
#22724=AXIS2_PLACEMENT_3D ( 'NONE', #28539, #6700, #6391 ) ;
#22725=CARTESIAN_POINT ( 'NONE',  ( 26.85107532351766224, -65.44994441702223753, 1.633352019574016101 ) ) ;
#22727=CARTESIAN_POINT ( 'NONE',  ( -18.29779733850000056, -18.85499412049999890, 12.26174568899999962 ) ) ;
#22729=DIRECTION ( 'NONE',  ( 1.000000000000000000, 0.000000000000000000, 0.000000000000000000 ) ) ;
#22731=CARTESIAN_POINT ( 'NONE',  ( 7.623622776310000404, -34.72967069919999972, -21.24008983309999721 ) ) ;
#22733=DIRECTION ( 'NONE',  ( 0.9952295494196654602, 0.000000000000000000, -0.09756097560976760563 ) ) ;
#22735=CARTESIAN_POINT ( 'NONE',  ( 47.25000000000000000, -79.00000000000000000, -7.709388683000000122E-13 ) ) ;
#22738=CARTESIAN_POINT ( 'NONE',  ( -12.04445256950000065, -60.59277760239999822, -20.32308874549999800 ) ) ;
#22739=VECTOR ( 'NONE', #20234, 1000.000000000000000 ) ;
#22740=DIRECTION ( 'NONE',  ( 0.9659258262889443003, 0.000000000000000000, 0.2588190451029837025 ) ) ;
#22743=CARTESIAN_POINT ( 'NONE',  ( 47.00156242777739379, -74.14776025066879583, -1.881670998416149043 ) ) ;
#22744=EDGE_LOOP ( 'NONE', ( #12382, #21131, #27738 ) ) ;
#22745=CARTESIAN_POINT ( 'NONE',  ( -13.07981419989999949, -42.23578978099999404, 20.15285454340000015 ) ) ;
#22748=EDGE_CURVE ( 'NONE', #22866, #14159, #3829, .T. ) ;
#22749=CARTESIAN_POINT ( 'NONE',  ( 32.97008024890000399, -74.00000000000000000, -20.36016474349999683 ) ) ;
#22750=EDGE_CURVE ( 'NONE', #23155, #11892, #9877, .T. ) ;
#22755=CARTESIAN_POINT ( 'NONE',  ( 21.51900322300193125, -37.41278966410947504, -7.708623769554239225 ) ) ;
#22756=VERTEX_POINT ( 'NONE', #20471 ) ;
#22759=CARTESIAN_POINT ( 'NONE',  ( -32.61798276849999922, -80.00000022860000115, -22.71848792340000145 ) ) ;
#22760=CARTESIAN_POINT ( 'NONE',  ( -21.01946775511974153, -64.01693695481982616, 12.95761361222880659 ) ) ;
#22762=CARTESIAN_POINT ( 'NONE',  ( -32.47291160230000173, -74.11800272920001476, -21.73792012110000016 ) ) ;
#22766=CARTESIAN_POINT ( 'NONE',  ( 7.674432201710000179, -64.79179280459999291, -23.81666465429999846 ) ) ;
#22769=CARTESIAN_POINT ( 'NONE',  ( -18.87648895869999777, -32.72716367869999488, 12.65371557960000004 ) ) ;
#22771=CARTESIAN_POINT ( 'NONE',  ( -16.49390888960000368, -74.50000000000000000, 44.28897684009999836 ) ) ;
#22772=CARTESIAN_POINT ( 'NONE',  ( -16.95867319479999935, -80.00000000000000000, 44.10460184009999551 ) ) ;
#22774=AXIS2_PLACEMENT_3D ( 'NONE', #10861, #291, #26490 ) ;
#22777=VERTEX_POINT ( 'NONE', #13912 ) ;
#22782=VERTEX_POINT ( 'NONE', #8793 ) ;
#22783=CARTESIAN_POINT ( 'NONE',  ( -11.41039530250000134, -19.15810975349999978, -18.83652256670000114 ) ) ;
#22784=EDGE_CURVE ( 'NONE', #9115, #25644, #10187, .T. ) ;
#22785=DIRECTION ( 'NONE',  ( -0.7071067811865474617, 0.000000000000000000, -0.7071067811865474617 ) ) ;
#22787=CARTESIAN_POINT ( 'NONE',  ( 9.564509902230000193, -57.40875702419999982, -23.52622212079999997 ) ) ;
#22788=CARTESIAN_POINT ( 'NONE',  ( 8.173922678290001187, -37.03252586920000056, -21.52373127659999952 ) ) ;
#22791=EDGE_CURVE ( 'NONE', #13203, #17392, #5375, .T. ) ;
#22792=LINE ( 'NONE', #20154, #1624 ) ;
#22796=CARTESIAN_POINT ( 'NONE',  ( -1.918209658487193048, -19.46987374641862445, -22.48175606853765274 ) ) ;
#22798=CARTESIAN_POINT ( 'NONE',  ( -1.158253037809999997, -52.63055504180000099, -23.23212522879999753 ) ) ;
#22800=VECTOR ( 'NONE', #14486, 1000.000000000000000 ) ;
#22801=CIRCLE ( 'NONE', #6984, 39.25000000000000000 ) ;
#22802=DIRECTION ( 'NONE',  ( 0.000000000000000000, -1.000000000000000000, 0.000000000000000000 ) ) ;
#22803=CARTESIAN_POINT ( 'NONE',  ( 7.215414233289999757, -84.00000000000000000, 40.70731707320000226 ) ) ;
#22804=CARTESIAN_POINT ( 'NONE',  ( 22.99217564430000138, -49.05622624239999396, -9.391640714770000287 ) ) ;
#22805=CARTESIAN_POINT ( 'NONE',  ( 8.963581071913218068, -35.44265712976643812, -20.01429396093944391 ) ) ;
#22806=CARTESIAN_POINT ( 'NONE',  ( 36.28164458690000060, -74.50000000000000000, -14.97346873880000118 ) ) ;
#22808=CARTESIAN_POINT ( 'NONE',  ( 36.70830950850000107, -75.00000021370000525, -14.75000047660000035 ) ) ;
#22809=CARTESIAN_POINT ( 'NONE',  ( -32.66023294069999849, -74.45928706499999805, -21.85457041699999792 ) ) ;
#22810=CARTESIAN_POINT ( 'NONE',  ( -22.50202996513547049, -79.94734758359761884, -32.71763195124997026 ) ) ;
#22812=CARTESIAN_POINT ( 'NONE',  ( 8.803829365699998633, -35.83655744470000570, -20.72386466589999898 ) ) ;
#22814=CARTESIAN_POINT ( 'NONE',  ( -2.578307999469999778, -52.56313962710000709, -25.11373953509999879 ) ) ;
#22827=CARTESIAN_POINT ( 'NONE',  ( 1.353583911619999998E-12, -74.50000000000000000, 1.342925770590000058E-12 ) ) ;
#22828=CARTESIAN_POINT ( 'NONE',  ( -10.73983547945041472, -19.46468314325315419, 19.23955065568980771 ) ) ;
#22830=DIRECTION ( 'NONE',  ( 0.9295286103719527793, 0.000000000000000000, 0.3687499999999814260 ) ) ;
#22831=CARTESIAN_POINT ( 'NONE',  ( -7.230685509177152248, -74.36482065499500038, -40.53346806266115010 ) ) ;
#22832=CARTESIAN_POINT ( 'NONE',  ( -14.57413617419999952, -74.20280742140000996, 36.34762531509999661 ) ) ;
#22833=CARTESIAN_POINT ( 'NONE',  ( -22.01499327390000005, -68.08608899289998817, 14.79936569140000024 ) ) ;
#22834=CARTESIAN_POINT ( 'NONE',  ( -13.46276276179999876, -19.49999999970000175, 20.39865906480000035 ) ) ;
#22835=ORIENTED_EDGE ( 'NONE', *, *, #4036, .F. ) ;
#22836=CARTESIAN_POINT ( 'NONE',  ( -12.07668570139999886, -70.04473456239999507, -25.34381927969999992 ) ) ;
#22837=DIRECTION ( 'NONE',  ( 1.000000000000000000, 0.000000000000000000, 0.000000000000000000 ) ) ;
#22840=AXIS2_PLACEMENT_3D ( 'NONE', #26431, #23957, #3991 ) ;
#22843=VECTOR ( 'NONE', #21579, 1000.000000000000000 ) ;
#22846=EDGE_LOOP ( 'NONE', ( #319, #23493, #26614, #22436 ) ) ;
#22847=CARTESIAN_POINT ( 'NONE',  ( -1.450351827910000058, -57.47122586340000083, -23.51019412459999813 ) ) ;
#22851=EDGE_CURVE ( 'NONE', #3056, #27919, #5235, .T. ) ;
#22853=ORIENTED_EDGE ( 'NONE', *, *, #27194, .F. ) ;
#22855=CARTESIAN_POINT ( 'NONE',  ( 21.92361644269999843, -37.64807918350000193, -8.681080957089999828 ) ) ;
#22856=CARTESIAN_POINT ( 'NONE',  ( 47.16788169050000334, -74.59616887820000386, -1.399136062990000040 ) ) ;
#22859=CARTESIAN_POINT ( 'NONE',  ( 7.208933142638366043, -73.58711170886618902, -39.22862632807101591 ) ) ;
#22861=CIRCLE ( 'NONE', #18187, 0.4999999999999967804 ) ;
#22863=CARTESIAN_POINT ( 'NONE',  ( 23.50166587798742412, -64.58097839926523420, 10.73601817129581981 ) ) ;
#22864=CARTESIAN_POINT ( 'NONE',  ( -1.546569514440000015, -66.56254540410000686, -25.78631783400000188 ) ) ;
#22865=CARTESIAN_POINT ( 'NONE',  ( -16.35365950510000133, -70.21389208120000092, 23.31707131299999958 ) ) ;
#22866=VERTEX_POINT ( 'NONE', #12004 ) ;
#22868=CARTESIAN_POINT ( 'NONE',  ( -2.587281614239999694, -58.59418584699999855, -25.28476954130000109 ) ) ;
#22869=CARTESIAN_POINT ( 'NONE',  ( 23.68479145319999901, -60.57882006589999691, 0.02928418074640000077 ) ) ;
#22870=CARTESIAN_POINT ( 'NONE',  ( -22.13232332860000184, -74.50000000000000000, -32.73892504640000567 ) ) ;
#22873=CARTESIAN_POINT ( 'NONE',  ( -7.377395436790557426, -73.99965292983208087, 39.26711817943528615 ) ) ;
#22874=CARTESIAN_POINT ( 'NONE',  ( 36.46922389885823890, -74.05666263691847462, -14.08207577745026562 ) ) ;
#22878=CARTESIAN_POINT ( 'NONE',  ( 23.74633046639999989, -64.47177090210000472, 10.70095004270000061 ) ) ;
#22882=ORIENTED_EDGE ( 'NONE', *, *, #13377, .T. ) ;
#22889=CARTESIAN_POINT ( 'NONE',  ( -12.23534022509999986, -63.58862135099999335, -21.26946117359999988 ) ) ;
#22890=EDGE_CURVE ( 'NONE', #5527, #21711, #16139, .T. ) ;
#22892=CARTESIAN_POINT ( 'NONE',  ( -37.60355029590000697, -74.00000000000000000, -9.356041104380000917 ) ) ;
#22893=ORIENTED_EDGE ( 'NONE', *, *, #23477, .T. ) ;
#22894=DIRECTION ( 'NONE',  ( 0.7071067811865475727, 0.000000000000000000, 0.7071067811865475727 ) ) ;
#22895=CARTESIAN_POINT ( 'NONE',  ( 47.14681262259601624, -74.43066600419328438, -1.228599301886279083 ) ) ;
#22897=CARTESIAN_POINT ( 'NONE',  ( 20.49588873660000132, -52.63280639840000674, 10.85734681379999955 ) ) ;
#22898=CARTESIAN_POINT ( 'NONE',  ( -2.578307999469999778, -45.73899999920000425, -25.11373953509999879 ) ) ;
#22899=EDGE_LOOP ( 'NONE', ( #21945, #1499, #14535, #5774, #13067, #26443 ) ) ;
#22900=DIRECTION ( 'NONE',  ( 0.000000000000000000, 1.000000000000000000, 0.000000000000000000 ) ) ;
#22902=CARTESIAN_POINT ( 'NONE',  ( -0.5380693342220000952, -55.86335041469999396, -23.29854462139999782 ) ) ;
#22903=CARTESIAN_POINT ( 'NONE',  ( -10.54477336451839165, -19.46993844407590402, -19.95170415067392256 ) ) ;
#22905=CARTESIAN_POINT ( 'NONE',  ( -10.93437413680000070, -19.50000027030000282, -21.85842452360000010 ) ) ;
#22907=CARTESIAN_POINT ( 'NONE',  ( 9.575769126168214740, -58.58842956003458369, -23.55923831042092331 ) ) ;
#22910=CARTESIAN_POINT ( 'NONE',  ( -32.37889788280000403, -80.19684081550001054, -22.28728604720000206 ) ) ;
#22913=VERTEX_POINT ( 'NONE', #1946 ) ;
#22917=EDGE_LOOP ( 'NONE', ( #18372, #3449, #20964, #3239 ) ) ;
#22919=CARTESIAN_POINT ( 'NONE',  ( -18.99796627190000109, -26.09744228899999996, 11.61130727839999821 ) ) ;
#22920=DIRECTION ( 'NONE',  ( -0.6710129359900831592, 0.000000000000000000, 0.7414456417930908039 ) ) ;
#22921=DIRECTION ( 'NONE',  ( 0.000000000000000000, 1.000000000000000000, 0.000000000000000000 ) ) ;
#22922=CARTESIAN_POINT ( 'NONE',  ( 22.95932757850000172, -57.43039251880000506, -9.307781678039997786 ) ) ;
#22925=CARTESIAN_POINT ( 'NONE',  ( 26.67136988580000079, -64.89183635380001647, 1.586600751119999764 ) ) ;
#22926=ADVANCED_FACE ( 'NONE', ( #23655 ), #10503, .F. ) ;
#22927=AXIS2_PLACEMENT_3D ( 'NONE', #20318, #24703, #2265 ) ;
#22930=CARTESIAN_POINT ( 'NONE',  ( 20.40611818609999872, -54.57118573399999661, 11.16247708059999866 ) ) ;
#22931=DIRECTION ( 'NONE',  ( 1.000000000000000000, 0.000000000000000000, 0.000000000000000000 ) ) ;
#22932=CARTESIAN_POINT ( 'NONE',  ( 21.78580818670000241, -37.64222968090000165, -8.476164596309999411 ) ) ;
#22934=VERTEX_POINT ( 'NONE', #8203 ) ;
#22935=FACE_OUTER_BOUND ( 'NONE', #26852, .T. ) ;
#22937=B_SPLINE_SURFACE_WITH_KNOTS ( 'NONE', 5, 5, ( 
 ( #9051, #2220, #17955, #19978, #6742, #4105, #6590, #24363, #17374 ),
 ( #6884, #51, #4404, #26268, #24506, #13420, #2370, #12976, #1939 ),
 ( #19691, #17517, #26404, #24220, #4254, #25101, #5283, #645, #11964 ),
 ( #9779, #5135, #3111, #498, #14170, #20280, #9192, #27143, #18693 ),
 ( #27588, #13869, #5422, #14016, #937, #7629, #16494, #25397, #14306 ),
 ( #9495, #2964, #9346, #23201, #20878, #347, #22922, #20737, #11823 ) ),
 .UNSPECIFIED., .F., .F., .F.,
 ( 6, 6 ),
 ( 6, 3, 6 ),
 ( 26.76256113009999993, 37.28868011619999834 ),
 ( 0.000000000000000000, 1.000000000000000000, 2.000000000000000000 ),
 .UNSPECIFIED. ) ;
#22940=DIRECTION ( 'NONE',  ( 1.000000000000000000, 0.000000000000000000, 5.788992577199999305E-17 ) ) ;
#22944=VECTOR ( 'NONE', #1398, 1000.000000000000000 ) ;
#22945=CARTESIAN_POINT ( 'NONE',  ( 23.33156623710000233, -18.50000000000000000, 2.512796439940000237 ) ) ;
#22948=PLANE ( 'NONE',  #13179 ) ;
#22951=CARTESIAN_POINT ( 'NONE',  ( -2.567353809430000133, -52.57401960330000179, -24.80239345940000106 ) ) ;
#22952=B_SPLINE_CURVE_WITH_KNOTS ( 'NONE', 5,
 ( #22834, #5343, #13933, #11735, #5043, #11885, #25165, #16690, #7690 ),
 .UNSPECIFIED., .F., .F.,
 ( 6, 3, 6 ),
 ( -86.65534111079999491, -83.85288688999999351, -33.01978394879999712 ),
 .UNSPECIFIED. ) ;
#22954=CARTESIAN_POINT ( 'NONE',  ( -7.325370793560000315, -45.73899999920000425, -24.94672208400000102 ) ) ;
#22956=CARTESIAN_POINT ( 'NONE',  ( 21.56931441200000421, -36.56979899360000275, -6.850353673489999906 ) ) ;
#22957=DIRECTION ( 'NONE',  ( 0.000000000000000000, 1.000000000000000000, 0.000000000000000000 ) ) ;
#22960=EDGE_CURVE ( 'NONE', #13357, #23740, #13341, .T. ) ;
#22961=CARTESIAN_POINT ( 'NONE',  ( -32.69645380010000224, -74.50000000299999670, -21.71458329220000039 ) ) ;
#22962=CARTESIAN_POINT ( 'NONE',  ( -32.66023292159999869, -79.50000000000062528, -21.85457041760000152 ) ) ;
#22964=CARTESIAN_POINT ( 'NONE',  ( -13.78120180950000062, -66.79737695549998477, 22.18107486459999933 ) ) ;
#22965=CARTESIAN_POINT ( 'NONE',  ( 21.19870159919999963, -35.15967237200000284, -7.969913383650000682 ) ) ;
#22966=CARTESIAN_POINT ( 'NONE',  ( 36.75261502460000429, -80.49999978700000725, -13.77875165610000074 ) ) ;
#22967=AXIS2_PLACEMENT_3D ( 'NONE', #18669, #6085, #12632 ) ;
#22972=CARTESIAN_POINT ( 'NONE',  ( 37.60355029590000697, -84.50000000000000000, 9.356041104380000917 ) ) ;
#22974=EDGE_LOOP ( 'NONE', ( #798, #2344, #9470, #21666 ) ) ;
#22978=CARTESIAN_POINT ( 'NONE',  ( -12.09704001540000107, -74.00000000000000000, 47.10905722069999513 ) ) ;
#22982=VERTEX_POINT ( 'NONE', #19987 ) ;
#22983=CARTESIAN_POINT ( 'NONE',  ( -13.09652604470000092, -71.22348525710000899, -24.69511647019999856 ) ) ;
#22985=DIRECTION ( 'NONE',  ( 0.000000000000000000, 1.000000000000000000, 0.000000000000000000 ) ) ;
#22987=CARTESIAN_POINT ( 'NONE',  ( 3.907985046679999924E-15, -73.50000000000000000, -40.00000000000000000 ) ) ;
#22990=ADVANCED_FACE ( 'NONE', ( #57 ), #21504, .F. ) ;
#22993=CARTESIAN_POINT ( 'NONE',  ( -0.8479729843809999945, -57.47815889169999792, -23.34776883199999986 ) ) ;
#22997=EDGE_LOOP ( 'NONE', ( #6911, #14607, #26706 ) ) ;
#22999=CARTESIAN_POINT ( 'NONE',  ( -7.215414233289999757, -84.00000000000000000, -40.70731707320000226 ) ) ;
#23009=CARTESIAN_POINT ( 'NONE',  ( -0.8905213842159999116, -65.59529275500000267, -25.37156472860000278 ) ) ;
#23011=ORIENTED_EDGE ( 'NONE', *, *, #19283, .T. ) ;
#23012=CARTESIAN_POINT ( 'NONE',  ( -14.59815773840000830, -79.49999996002311775, 36.63377407710000000 ) ) ;
#23015=CARTESIAN_POINT ( 'NONE',  ( 24.14381995990000007, -62.06858034060000762, 0.2946074132029999904 ) ) ;
#23016=CARTESIAN_POINT ( 'NONE',  ( 19.47627435319999734, -35.29258001769999709, -8.987105447939999436 ) ) ;
#23018=CIRCLE ( 'NONE', #8542, 3.499999999999999556 ) ;
#23019=CARTESIAN_POINT ( 'NONE',  ( -1.001103094699999918, -19.15716910929999628, -22.00374779629999722 ) ) ;
#23020=CARTESIAN_POINT ( 'NONE',  ( 36.50961708847058418, -74.07907867045096850, -14.14048807786333661 ) ) ;
#23021=EDGE_LOOP ( 'NONE', ( #17863, #22010, #13888, #27238 ) ) ;
#23022=CARTESIAN_POINT ( 'NONE',  ( -11.53828505259999915, -18.50000000000000000, 18.05193266499999893 ) ) ;
#23024=CARTESIAN_POINT ( 'NONE',  ( 23.67927593730000169, -62.35648592489999942, 10.61505170350000071 ) ) ;
#23025=CARTESIAN_POINT ( 'NONE',  ( 8.791129346259999977, -34.94311270309999884, -20.42416734049999860 ) ) ;
#23029=CIRCLE ( 'NONE', #28587, 7.250000000000000000 ) ;
#23030=DIRECTION ( 'NONE',  ( 0.9295286103719527793, 0.000000000000000000, 0.3687499999999814260 ) ) ;
#23031=CARTESIAN_POINT ( 'NONE',  ( -11.20518065289999932, -58.91551295370000219, -21.78293632669999980 ) ) ;
#23032=AXIS2_PLACEMENT_3D ( 'NONE', #7114, #4332, #18326 ) ;
#23033=CARTESIAN_POINT ( 'NONE',  ( 19.97576656849999921, -17.00000000000000000, -19.97576656849999921 ) ) ;
#23037=EDGE_LOOP ( 'NONE', ( #6841, #9020, #28638, #24207 ) ) ;
#23039=CARTESIAN_POINT ( 'NONE',  ( -11.09899533129999938, -34.67032517180000895, 19.64911088110000037 ) ) ;
#23045=B_SPLINE_CURVE_WITH_KNOTS ( 'NONE', 5,
 ( #5806, #10433, #15093, #12766, #21677, #10565 ),
 .UNSPECIFIED., .F., .F.,
 ( 6, 6 ),
 ( 0.000000000000000000, 1.000000000000000000 ),
 .UNSPECIFIED. ) ;
#23047=EDGE_CURVE ( 'NONE', #5390, #20659, #25706, .T. ) ;
#23048=CARTESIAN_POINT ( 'NONE',  ( 39.07223452259999874, -73.87252278319999732, 7.323177335930000531 ) ) ;
#23051=CARTESIAN_POINT ( 'NONE',  ( 26.61465604159999998, -68.28989644159999273, 0.1578853838729999959 ) ) ;
#23052=DIRECTION ( 'NONE',  ( 1.000000000000000000, 0.000000000000000000, 0.000000000000000000 ) ) ;
#23054=CARTESIAN_POINT ( 'NONE',  ( -32.73892504640000567, -79.50000000000000000, -22.13232332860000184 ) ) ;
#23058=ORIENTED_EDGE ( 'NONE', *, *, #26319, .T. ) ;
#23062=CARTESIAN_POINT ( 'NONE',  ( 22.96745989159999723, -18.50000000000000000, 9.091461454319999191 ) ) ;
#23065=VECTOR ( 'NONE', #9375, 1000.000000000000000 ) ;
#23067=CARTESIAN_POINT ( 'NONE',  ( 0.000000000000000000, -84.00000000000000000, 0.000000000000000000 ) ) ;
#23068=CARTESIAN_POINT ( 'NONE',  ( 30.91973185770000043, -72.00365067099998839, -22.05221014440000005 ) ) ;
#23071=CARTESIAN_POINT ( 'NONE',  ( -39.40310785696919282, -73.65029154571925574, -7.225850277565577073 ) ) ;
#23073=CARTESIAN_POINT ( 'NONE',  ( 21.59677465600000090, -37.21264878210000404, -8.299693975220000297 ) ) ;
#23077=CARTESIAN_POINT ( 'NONE',  ( -11.41594931139999858, -19.46510050329999686, -18.84569254350000023 ) ) ;
#23079=CARTESIAN_POINT ( 'NONE',  ( 45.84677419350000349, -80.50000000000000000, -4.286925650119999709 ) ) ;
#23082=CARTESIAN_POINT ( 'NONE',  ( 9.414867375249999171, -40.68175103339999765, -23.05516474710000097 ) ) ;
#23089=CARTESIAN_POINT ( 'NONE',  ( -0.5856137342820000313, -19.46510053389999939, -22.02591827759999887 ) ) ;
#23090=EDGE_CURVE ( 'NONE', #26844, #25324, #24289, .T. ) ;
#23092=CARTESIAN_POINT ( 'NONE',  ( -1.203638492820000128, -32.73099401719999690, -22.54375384349999933 ) ) ;
#23093=CYLINDRICAL_SURFACE ( 'NONE', #10269, 39.24999999999998579 ) ;
#23094=EDGE_CURVE ( 'NONE', #14431, #14119, #7606, .T. ) ;
#23095=CARTESIAN_POINT ( 'NONE',  ( 1.598721155460000041E-15, -84.50000000000000000, 6.905587213169999654E-15 ) ) ;
#23096=CARTESIAN_POINT ( 'NONE',  ( 20.36016146999999776, -74.00000000000000000, -32.97008227039999895 ) ) ;
#23097=CARTESIAN_POINT ( 'NONE',  ( 23.05516474710000097, -40.68175103160000106, -9.414867375240000058 ) ) ;
#23098=DIRECTION ( 'NONE',  ( 0.9995627462972740407, 0.000000000000000000, -0.02956883857460809381 ) ) ;
#23102=CARTESIAN_POINT ( 'NONE',  ( -20.45998242170000125, -19.50000000000000000, 14.78974999389999923 ) ) ;
#23103=AXIS2_PLACEMENT_3D ( 'NONE', #28745, #4290, #13605 ) ;
#23105=CARTESIAN_POINT ( 'NONE',  ( 19.43643868430000410, -34.66800417059999262, -8.988996095199999203 ) ) ;
#23106=DIRECTION ( 'NONE',  ( 0.000000000000000000, 1.000000000000000000, 0.000000000000000000 ) ) ;
#23112=ORIENTED_EDGE ( 'NONE', *, *, #5536, .T. ) ;
#23115=EDGE_CURVE ( 'NONE', #11794, #22379, #1986, .T. ) ;
#23118=FACE_OUTER_BOUND ( 'NONE', #22192, .T. ) ;
#23119=CARTESIAN_POINT ( 'NONE',  ( 20.30284733819999943, -72.62832350799999404, -31.03260099770000124 ) ) ;
#23120=EDGE_CURVE ( 'NONE', #7945, #3120, #6165, .T. ) ;
#23121=CARTESIAN_POINT ( 'NONE',  ( -34.06928787630000244, -74.00000000000000000, -24.16979293970000242 ) ) ;
#23124=CARTESIAN_POINT ( 'NONE',  ( -1.065814103639999922E-14, -36.00000000000000000, 3.552713678799999608E-15 ) ) ;
#23129=ORIENTED_EDGE ( 'NONE', *, *, #499, .T. ) ;
#23130=CARTESIAN_POINT ( 'NONE',  ( -2.565551289909999699, -58.22369335140000146, -24.95564358469999888 ) ) ;
#23136=CARTESIAN_POINT ( 'NONE',  ( 25.26718046270000073, -45.73899999920000425, 6.129403842640000377 ) ) ;
#23141=DIRECTION ( 'NONE',  ( 1.000000000000000000, 0.000000000000000000, 0.000000000000000000 ) ) ;
#23144=CARTESIAN_POINT ( 'NONE',  ( -14.59464643419999952, -80.37541664939999464, 36.43768143699999484 ) ) ;
#23146=CARTESIAN_POINT ( 'NONE',  ( -2.199961190620000284, -69.66720773099999064, -27.15830649919999829 ) ) ;
#23150=ADVANCED_FACE ( 'NONE', ( #15347 ), #26016, .F. ) ;
#23151=CARTESIAN_POINT ( 'NONE',  ( -14.93121078260000090, -79.49999975080000070, 36.29905569799999654 ) ) ;
#23153=CARTESIAN_POINT ( 'NONE',  ( 24.71478484869999903, -57.43018266680000039, 1.313252026010000018 ) ) ;
#23154=CARTESIAN_POINT ( 'NONE',  ( -20.51803184719999962, -63.41300277309999700, 14.12505980070000078 ) ) ;
#23155=VERTEX_POINT ( 'NONE', #14926 ) ;
#23156=CARTESIAN_POINT ( 'NONE',  ( -19.81272040990000249, -52.63293862049999916, 12.05498172269999912 ) ) ;
#23157=CARTESIAN_POINT ( 'NONE',  ( -2.784644191329999963, -18.86932112550000085, -24.02237818909999945 ) ) ;
#23160=DIRECTION ( 'NONE',  ( 0.000000000000000000, 1.000000000000000000, 0.000000000000000000 ) ) ;
#23161=B_SPLINE_CURVE_WITH_KNOTS ( 'NONE', 3,
 ( #17876, #11136, #17733, #15519 ),
 .UNSPECIFIED., .F., .F.,
 ( 4, 4 ),
 ( 12.34870497440000037, 33.81329059570000339 ),
 .UNSPECIFIED. ) ;
#23164=DIRECTION ( 'NONE',  ( -0.4913402003782836314, 0.000000000000000000, 0.8709677419355024153 ) ) ;
#23166=CARTESIAN_POINT ( 'NONE',  ( -12.60252398833393528, -66.16746083529757527, 22.33844947683535409 ) ) ;
#23167=ORIENTED_EDGE ( 'NONE', *, *, #27497, .F. ) ;
#23168=B_SPLINE_SURFACE_WITH_KNOTS ( 'NONE', 5, 5, ( 
 ( #4164, #2437, #21951, #8965, #8668, #2588 ),
 ( #11435, #26467, #8813, #26771, #6652, #19894 ),
 ( #17729, #11291, #6501, #9113, #15664, #24567 ),
 ( #4314, #15814, #13190, #2141, #26612, #10978 ),
 ( #24424, #4462, #21082, #23261, #27343, #5342 ),
 ( #22682, #9845, #7241, #4901, #25314, #11734 ) ),
 .UNSPECIFIED., .F., .F., .F.,
 ( 6, 6 ),
 ( 6, 6 ),
 ( 39.35985658629999762, 51.33494166999999919 ),
 ( 0.000000000000000000, 2.000000000000000000 ),
 .UNSPECIFIED. ) ;
#23169=CARTESIAN_POINT ( 'NONE',  ( -12.30135761330000044, -18.50000000000000000, 18.36349993190000163 ) ) ;
#23170=CARTESIAN_POINT ( 'NONE',  ( 37.09123793775638944, -79.93210607435938186, -14.11230097129613981 ) ) ;
#23171=CARTESIAN_POINT ( 'NONE',  ( 26.38214771250000013, -68.90972708120000334, -11.00107859539999922 ) ) ;
#23172=DIRECTION ( 'NONE',  ( 1.000000000000000000, 0.000000000000000000, 0.000000000000000000 ) ) ;
#23174=CIRCLE ( 'NONE', #1293, 39.25000000000000000 ) ;
#23175=CARTESIAN_POINT ( 'NONE',  ( -11.78425688200000110, -72.00000000000000000, -26.58404760160000180 ) ) ;
#23177=CARTESIAN_POINT ( 'NONE',  ( -13.20732654740000100, -27.02040028920000125, 19.97234870039999777 ) ) ;
#23180=LINE ( 'NONE', #4961, #11271 ) ;
#23181=EDGE_CURVE ( 'NONE', #5907, #5258, #11220, .T. ) ;
#23183=CARTESIAN_POINT ( 'NONE',  ( -10.83440914901318308, -19.46558565663113072, -19.38001281541565390 ) ) ;
#23186=CARTESIAN_POINT ( 'NONE',  ( 3.551183598479999925E-15, -73.50000000000000000, -32.75000000000000000 ) ) ;
#23187=CARTESIAN_POINT ( 'NONE',  ( 47.01293135346697483, -79.64648171702511092, -2.320651118032621252 ) ) ;
#23188=ORIENTED_EDGE ( 'NONE', *, *, #3977, .T. ) ;
#23192=ORIENTED_EDGE ( 'NONE', *, *, #23432, .F. ) ;
#23193=CARTESIAN_POINT ( 'NONE',  ( -0.7293611917560000046, -79.74815767519999099, 47.25048488379999867 ) ) ;
#23194=DIRECTION ( 'NONE',  ( -1.000000000000000000, 0.000000000000000000, 0.000000000000000000 ) ) ;
#23196=CIRCLE ( 'NONE', #25519, 2.000000000000002665 ) ;
#23198=CARTESIAN_POINT ( 'NONE',  ( -18.66186151429999995, -26.09432050510000067, 12.57601491380000169 ) ) ;
#23199=DIRECTION ( 'NONE',  ( 0.000000000000000000, -1.000000000000000000, 0.000000000000000000 ) ) ;
#23200=CARTESIAN_POINT ( 'NONE',  ( 29.97212741979999961, -73.66823234569999101, -25.11762090529999725 ) ) ;
#23201=CARTESIAN_POINT ( 'NONE',  ( 22.16163108380000324, -57.47158985090000272, -7.992697376199999759 ) ) ;
#23202=EDGE_CURVE ( 'NONE', #23575, #23580, #5259, .T. ) ;
#23203=CARTESIAN_POINT ( 'NONE',  ( 25.54892705720000023, -65.52795386139999323, 0.7157854019699999570 ) ) ;
#23204=B_SPLINE_CURVE_WITH_KNOTS ( 'NONE', 5,
 ( #17772, #19507, #6390, #22142, #17184, #15254 ),
 .UNSPECIFIED., .F., .F.,
 ( 6, 6 ),
 ( 0.000000000000000000, 1.000000000000000000 ),
 .UNSPECIFIED. ) ;
#23207=CARTESIAN_POINT ( 'NONE',  ( -19.73459494445757656, -19.18584080450766294, 14.41863469506854045 ) ) ;
#23208=CARTESIAN_POINT ( 'NONE',  ( 21.63730777760000024, -37.52726933430000145, -8.187370782949999537 ) ) ;
#23214=CARTESIAN_POINT ( 'NONE',  ( -21.35786096709999882, -65.07443093669999712, 13.27975207949999970 ) ) ;
#23215=CARTESIAN_POINT ( 'NONE',  ( -18.78219790299999659, -19.46510053389999939, 11.52011550950000007 ) ) ;
#23216=CARTESIAN_POINT ( 'NONE',  ( 9.381593461630000519, -36.50000000249999488, -22.93608650079999833 ) ) ;
#23217=DIRECTION ( 'NONE',  ( 1.000000000000000000, 0.000000000000000000, 0.000000000000000000 ) ) ;
#23218=ORIENTED_EDGE ( 'NONE', *, *, #22748, .F. ) ;
#23219=CARTESIAN_POINT ( 'NONE',  ( -40.29126735535079007, -74.18164516875299341, 7.244146985818024298 ) ) ;
#23221=FACE_OUTER_BOUND ( 'NONE', #13943, .T. ) ;
#23224=CARTESIAN_POINT ( 'NONE',  ( 20.27108563890000070, -18.61794786490000320, -7.599202272009999426 ) ) ;
#23225=DIRECTION ( 'NONE',  ( -0.9295286103719527793, 0.000000000000000000, -0.3687499999999814260 ) ) ;
#23226=CARTESIAN_POINT ( 'NONE',  ( -0.8695967735199999771, -32.73235193869999904, -22.48267697900000428 ) ) ;
#23228=FACE_OUTER_BOUND ( 'NONE', #19358, .T. ) ;
#23229=CARTESIAN_POINT ( 'NONE',  ( -1.776356839399999804E-15, -19.00000000000000000, 0.000000000000000000 ) ) ;
#23230=CARTESIAN_POINT ( 'NONE',  ( 23.11289036089999982, -53.23790003319999897, -9.427231679889999327 ) ) ;
#23231=DIRECTION ( 'NONE',  ( 1.000000000000000000, 0.000000000000000000, 0.000000000000000000 ) ) ;
#23232=CARTESIAN_POINT ( 'NONE',  ( 36.25873697209999591, -74.65899625289999619, -15.02897531189999825 ) ) ;
#23233=EDGE_LOOP ( 'NONE', ( #9226, #11410, #710, #9135, #23791, #7265, #13103, #19267, #12664, #27276, #26720, #13710, #12551, #4077, #9185, #24910, #25883, #14858, #1444, #1829, #2224, #28218 ) ) ;
#23236=ADVANCED_FACE ( 'NONE', ( #28484 ), #14092, .T. ) ;
#23239=AXIS2_PLACEMENT_3D ( 'NONE', #16063, #24965, #13884 ) ;
#23240=ADVANCED_FACE ( 'NONE', ( #4150 ), #12656, .T. ) ;
#23241=DIRECTION ( 'NONE',  ( 0.000000000000000000, -1.000000000000000000, 0.000000000000000000 ) ) ;
#23242=CARTESIAN_POINT ( 'NONE',  ( 21.16123614720000035, -35.01845205400000083, -8.005892107839999383 ) ) ;
#23243=CARTESIAN_POINT ( 'NONE',  ( 7.234868202887432709, -73.70809116058434540, 39.52985788716055993 ) ) ;
#23244=EDGE_CURVE ( 'NONE', #11422, #16727, #23369, .T. ) ;
#23245=CARTESIAN_POINT ( 'NONE',  ( 35.14430554270000329, -74.00000000000000000, -13.75000000000000000 ) ) ;
#23246=CARTESIAN_POINT ( 'NONE',  ( -38.96765197713227025, -74.02518802155771027, 7.561758309935756373 ) ) ;
#23248=ORIENTED_EDGE ( 'NONE', *, *, #12301, .T. ) ;
#23250=CARTESIAN_POINT ( 'NONE',  ( -2.143666143589857853, -70.80051932422085770, -27.67943868423927967 ) ) ;
#23252=VERTEX_POINT ( 'NONE', #27186 ) ;
#23253=DIRECTION ( 'NONE',  ( 0.000000000000000000, -1.000000000000000000, 0.000000000000000000 ) ) ;
#23254=CIRCLE ( 'NONE', #15780, 21.03431122519999974 ) ;
#23256=FACE_OUTER_BOUND ( 'NONE', #10636, .T. ) ;
#23260=CARTESIAN_POINT ( 'NONE',  ( 23.74158351679999868, -72.51566206409999893, -30.51711889939999978 ) ) ;
#23261=CARTESIAN_POINT ( 'NONE',  ( 10.19708627540000023, -71.08735242909999386, -26.16648790640000044 ) ) ;
#23264=CARTESIAN_POINT ( 'NONE',  ( 8.966803191690001285, -31.61664946020000144, -19.80394353770000038 ) ) ;
#23265=PLANE ( 'NONE',  #18436 ) ;
#23272=ADVANCED_FACE ( 'NONE', ( #8947 ), #17339, .T. ) ;
#23273=AXIS2_PLACEMENT_3D ( 'NONE', #28607, #17403, #15180 ) ;
#23277=CARTESIAN_POINT ( 'NONE',  ( 21.34788034980000049, -35.28814072549999281, -7.426815654249999454 ) ) ;
#23279=ORIENTED_EDGE ( 'NONE', *, *, #9972, .F. ) ;
#23280=CARTESIAN_POINT ( 'NONE',  ( -7.188503037714309762, -73.76099369285560670, 38.70686955322251777 ) ) ;
#23281=ORIENTED_EDGE ( 'NONE', *, *, #15954, .T. ) ;
#23283=CARTESIAN_POINT ( 'NONE',  ( -11.77206978281909677, -63.23144003730045171, 21.39278812554018572 ) ) ;
#23285=CARTESIAN_POINT ( 'NONE',  ( -1.800052354129999976, -69.76823842119999597, -27.23143641409999915 ) ) ;
#23287=CARTESIAN_POINT ( 'NONE',  ( -15.78247551950000194, -71.67546720299999663, 23.43991392560000264 ) ) ;
#23289=CARTESIAN_POINT ( 'NONE',  ( 36.39633395910000502, -74.06425117190001117, -14.25343207329999906 ) ) ;
#23291=CARTESIAN_POINT ( 'NONE',  ( -20.66472140539999813, -61.67888006879999807, 14.89894363559999846 ) ) ;
#23293=DIRECTION ( 'NONE',  ( 1.836909530730000976E-16, 0.000000000000000000, -1.000000000000000000 ) ) ;
#23294=CARTESIAN_POINT ( 'NONE',  ( -3.258095469229999708, -18.50000000000000000, -23.26304047400000030 ) ) ;
#23296=ORIENTED_EDGE ( 'NONE', *, *, #23782, .F. ) ;
#23299=CARTESIAN_POINT ( 'NONE',  ( 36.78520401009999574, -79.52803893530000323, -14.62663614230000064 ) ) ;
#23300=CARTESIAN_POINT ( 'NONE',  ( -3.058911230670000148, -72.82938648530000592, -28.52031834779999997 ) ) ;
#23301=EDGE_LOOP ( 'NONE', ( #25660, #3624, #3161, #3724 ) ) ;
#23303=CARTESIAN_POINT ( 'NONE',  ( 37.29611236860000645, -80.00000000000000000, -13.75000000000000000 ) ) ;
#23305=FACE_OUTER_BOUND ( 'NONE', #17747, .T. ) ;
#23309=CIRCLE ( 'NONE', #2832, 3.499999999999999556 ) ;
#23310=CARTESIAN_POINT ( 'NONE',  ( 47.25000000000000000, -75.00000000000000000, -1.242228542250000064E-12 ) ) ;
#23312=CARTESIAN_POINT ( 'NONE',  ( -12.36746679350000022, -27.05111851250000043, 19.36625172230000302 ) ) ;
#23316=CARTESIAN_POINT ( 'NONE',  ( 21.34788034980000049, -35.28814072549999281, -7.426815654249999454 ) ) ;
#23317=B_SPLINE_CURVE_WITH_KNOTS ( 'NONE', 5,
 ( #12611, #10010, #28354, #28081, #21116, #1172 ),
 .UNSPECIFIED., .F., .F.,
 ( 6, 6 ),
 ( 0.000000000000000000, 1.000000000000000000 ),
 .UNSPECIFIED. ) ;
#23318=CARTESIAN_POINT ( 'NONE',  ( -7.215414233289999757, -74.50000000000000000, -40.70731707320000226 ) ) ;
#23319=CARTESIAN_POINT ( 'NONE',  ( 24.46180220976096464, -66.34775779038977817, -7.978790679046251277 ) ) ;
#23320=CARTESIAN_POINT ( 'NONE',  ( -17.94180966909999597, -45.73899999920000425, 18.81731824139999887 ) ) ;
#23323=CARTESIAN_POINT ( 'NONE',  ( -32.56379503299999811, -80.00863944699999308, -22.48295750460000164 ) ) ;
#23325=CARTESIAN_POINT ( 'NONE',  ( 0.000000000000000000, -86.00000000000000000, 0.000000000000000000 ) ) ;
#23326=ORIENTED_EDGE ( 'NONE', *, *, #11110, .F. ) ;
#23327=CIRCLE ( 'NONE', #16354, 0.5000000000000027756 ) ;
#23328=CARTESIAN_POINT ( 'NONE',  ( -1.482066257490000094, -79.94411376969999594, 47.15825498670000115 ) ) ;
#23329=DIRECTION ( 'NONE',  ( -0.9704142011833034598, 0.000000000000000000, 0.2414462220490750932 ) ) ;
#23330=ORIENTED_EDGE ( 'NONE', *, *, #17672, .F. ) ;
#23334=PLANE ( 'NONE',  #25048 ) ;
#23336=CARTESIAN_POINT ( 'NONE',  ( 30.57937519460000075, -72.84979523120000522, -23.65429679820000075 ) ) ;
#23337=CARTESIAN_POINT ( 'NONE',  ( -14.18731548340253035, -69.93408613758896308, 23.39951299694514475 ) ) ;
#23339=B_SPLINE_SURFACE_WITH_KNOTS ( 'NONE', 5, 5, ( 
 ( #25022, #20951, #3177, #13946, #12032, #22847, #16266, #22993, #20806 ),
 ( #2889, #9707, #719, #27511, #7559, #16420, #25327, #5357, #16565 ),
 ( #14242, #23130, #1010, #9855, #18764, #25461, #14379, #4145, #10401 ),
 ( #8517, #8228, #21644, #12447, #19448, #17124, #21781, #12730, #15194 ),
 ( #26310, #3730, #21360, #24111, #13020, #28480, #3585, #25742, #5768 ),
 ( #19319, #17418, #23683, #23550, #8366, #10678, #1418, #21933, #1981 ),
 ( #10824, #12590, #19733, #28195, #28621, #26167, #15059, #10263, #25879 ),
 ( #28335, #1833, #14655, #6332, #26012, #21502, #6037, #16849, #19592 ),
 ( #23969, #19174, #28063, #8099, #16989, #14922, #4005, #17272, #5903 ) ),
 .UNSPECIFIED., .F., .F., .F.,
 ( 6, 3, 6 ),
 ( 6, 3, 6 ),
 ( 112.4516929440000013, 115.4092999559999981, 122.9563471680000077 ),
 ( 0.000000000000000000, 1.000000000000000000, 2.000000000000000000 ),
 .UNSPECIFIED. ) ;
#23341=EDGE_CURVE ( 'NONE', #10820, #8919, #13618, .T. ) ;
#23342=ORIENTED_EDGE ( 'NONE', *, *, #9383, .T. ) ;
#23343=CARTESIAN_POINT ( 'NONE',  ( -40.25190969051858048, -74.15297958058674510, -7.245634850454607978 ) ) ;
#23344=DIRECTION ( 'NONE',  ( 0.000000000000000000, -1.000000000000000000, 0.000000000000000000 ) ) ;
#23345=CARTESIAN_POINT ( 'NONE',  ( 21.11247224599999939, -36.35195199729999871, -8.702043174359999966 ) ) ;
#23348=CIRCLE ( 'NONE', #24254, 3.500000000000003109 ) ;
#23350=CARTESIAN_POINT ( 'NONE',  ( 7.771052952609999345E-15, -82.25000000000000000, -47.25000000000000000 ) ) ;
#23351=CIRCLE ( 'NONE', #21034, 38.75000000000000000 ) ;
#23354=CARTESIAN_POINT ( 'NONE',  ( 8.968806686069999756, -40.71455396189999476, -22.20693316839999909 ) ) ;
#23358=EDGE_CURVE ( 'NONE', #18300, #5668, #18843, .T. ) ;
#23360=CARTESIAN_POINT ( 'NONE',  ( -13.46276276179999876, -19.49999999970000175, 20.39865906480000035 ) ) ;
#23363=CARTESIAN_POINT ( 'NONE',  ( 19.45828891929999926, -18.50000000000000000, -8.201027286100000424 ) ) ;
#23365=CARTESIAN_POINT ( 'NONE',  ( -14.93121066289999987, -74.43375220249998847, 36.29905574720000061 ) ) ;
#23369=B_SPLINE_CURVE_WITH_KNOTS ( 'NONE', 3,
 ( #22667, #17998, #9240, #7084 ),
 .UNSPECIFIED., .F., .F.,
 ( 4, 4 ),
 ( 0.000000000000000000, 1.000000000000000000 ),
 .UNSPECIFIED. ) ;
#23370=CARTESIAN_POINT ( 'NONE',  ( 8.991798710090000313, -35.60470291170000223, -19.53731210289999964 ) ) ;
#23371=CARTESIAN_POINT ( 'NONE',  ( 21.43629755400000292, -36.56833509949999694, -7.482057485250000362 ) ) ;
#23374=EDGE_LOOP ( 'NONE', ( #14002, #21506, #1583, #1591 ) ) ;
#23376=B_SPLINE_CURVE_WITH_KNOTS ( 'NONE', 5,
 ( #13130, #13426, #9055, #22185, #28716, #17960 ),
 .UNSPECIFIED., .F., .F.,
 ( 6, 6 ),
 ( 0.000000000000000000, 1.000000000000000000 ),
 .UNSPECIFIED. ) ;
#23377=CARTESIAN_POINT ( 'NONE',  ( -32.67527182230000449, -74.45928706499999805, -22.00249031449999748 ) ) ;
#23380=CARTESIAN_POINT ( 'NONE',  ( 14.62430634820000108, -74.00000000000000000, 26.76961320899999919 ) ) ;
#23381=CARTESIAN_POINT ( 'NONE',  ( 8.346761719239998101, -35.62468481330000003, -21.07000052020000069 ) ) ;
#23383=CARTESIAN_POINT ( 'NONE',  ( -14.39036416260000095, -64.35840737179999849, 21.98073843050000065 ) ) ;
#23384=CARTESIAN_POINT ( 'NONE',  ( -40.35493623782935657, -74.39269056238592270, 7.250053749311780038 ) ) ;
#23385=CARTESIAN_POINT ( 'NONE',  ( 46.25000000000000000, -80.00000000000000000, -9.166287847479999584 ) ) ;
#23386=VERTEX_POINT ( 'NONE', #9028 ) ;
#23388=CARTESIAN_POINT ( 'NONE',  ( -26.33972759919999973, -79.50000000000000000, -36.23922253580000330 ) ) ;
#23389=ORIENTED_EDGE ( 'NONE', *, *, #21022, .T. ) ;
#23390=AXIS2_PLACEMENT_3D ( 'NONE', #388, #7081, #6783 ) ;
#23392=ORIENTED_EDGE ( 'NONE', *, *, #16533, .F. ) ;
#23398=EDGE_CURVE ( 'NONE', #13829, #15667, #5721, .T. ) ;
#23400=CARTESIAN_POINT ( 'NONE',  ( 27.75394116159999669, -74.50000000000000000, -27.75394116159999669 ) ) ;
#23402=B_SPLINE_SURFACE_WITH_KNOTS ( 'NONE', 5, 5, ( 
 ( #20279, #9344, #13724, #2668, #22624, #7182, #4981, #14443, #3650 ),
 ( #14576, #14305, #10185, #12247, #19101, #12103, #21159, #10048, #23068 ),
 ( #16627, #9778, #25523, #25809, #3382, #3110, #23336, #23606, #14168 ),
 ( #1214, #12514, #7890, #23481, #23200, #27989, #18962, #8024, #27845 ),
 ( #11963, #21019, #1080, #21424, #5835, #3247, #14716, #20877, #1483 ),
 ( #9919, #12376, #5692, #3520, #5281, #18833, #7482, #18691, #18539 ) ),
 .UNSPECIFIED., .F., .F., .F.,
 ( 6, 6 ),
 ( 6, 3, 6 ),
 ( 0.4663536434559999999, 13.03296576320000000 ),
 ( 0.000000000000000000, 1.000000000000000000, 2.000000000000000000 ),
 .UNSPECIFIED. ) ;
#23403=CARTESIAN_POINT ( 'NONE',  ( 0.000000000000000000, -65.07443093669999712, 0.000000000000000000 ) ) ;
#23404=CARTESIAN_POINT ( 'NONE',  ( 8.993760894959999419, -31.63434272479999976, -19.33939736140000321 ) ) ;
#23405=DIRECTION ( 'NONE',  ( 0.000000000000000000, 1.000000000000000000, 0.000000000000000000 ) ) ;
#23407=CARTESIAN_POINT ( 'NONE',  ( 19.98802563500222007, -19.46625705893007563, 9.814437999406528945 ) ) ;
#23409=CARTESIAN_POINT ( 'NONE',  ( -11.35954001540000036, -74.50000000000000000, 47.25000000000000000 ) ) ;
#23412=ORIENTED_EDGE ( 'NONE', *, *, #13382, .F. ) ;
#23414=ORIENTED_EDGE ( 'NONE', *, *, #10628, .F. ) ;
#23417=CARTESIAN_POINT ( 'NONE',  ( 19.49544348199999888, -35.50000000000000000, -8.986258402430001624 ) ) ;
#23418=DIRECTION ( 'NONE',  ( 0.000000000000000000, 1.000000000000000000, 0.000000000000000000 ) ) ;
#23419=ORIENTED_EDGE ( 'NONE', *, *, #16493, .F. ) ;
#23424=CARTESIAN_POINT ( 'NONE',  ( 9.092656154049999273, -35.82930178739999860, -19.86172366460000305 ) ) ;
#23425=VERTEX_POINT ( 'NONE', #11801 ) ;
#23428=B_SPLINE_CURVE_WITH_KNOTS ( 'NONE', 5,
 ( #7342, #11540, #24677, #13591, #11395, #4997 ),
 .UNSPECIFIED., .F., .F.,
 ( 6, 6 ),
 ( 0.000000000000000000, 1.000000000000000000 ),
 .UNSPECIFIED. ) ;
#23429=AXIS2_PLACEMENT_3D ( 'NONE', #9761, #20859, #25505 ) ;
#23430=CARTESIAN_POINT ( 'NONE',  ( -19.16298526259999946, -18.50000000000000000, 15.26553041949999923 ) ) ;
#23431=ORIENTED_EDGE ( 'NONE', *, *, #20847, .F. ) ;
#23432=EDGE_CURVE ( 'NONE', #24445, #15756, #3225, .T. ) ;
#23435=CARTESIAN_POINT ( 'NONE',  ( 23.90606521969999676, -57.45864773929999814, 0.8443132633689999222 ) ) ;
#23436=CARTESIAN_POINT ( 'NONE',  ( -21.04849736790000136, -64.58097846009999898, 14.98503047890000062 ) ) ;
#23437=EDGE_LOOP ( 'NONE', ( #17075, #7965, #20721, #21786 ) ) ;
#23438=DIRECTION ( 'NONE',  ( 1.000000000000000000, 0.000000000000000000, 0.000000000000000000 ) ) ;
#23439=EDGE_CURVE ( 'NONE', #12631, #22913, #10467, .T. ) ;
#23440=CARTESIAN_POINT ( 'NONE',  ( -7.301026670105736471, -73.99985427505767177, 39.56397514584002550 ) ) ;
#23441=CARTESIAN_POINT ( 'NONE',  ( 36.55403876290004916, -74.10879610147962637, -14.20614005299821159 ) ) ;
#23444=CIRCLE ( 'NONE', #10830, 4.750000000000000888 ) ;
#23447=CARTESIAN_POINT ( 'NONE',  ( 36.80029846600000099, -80.01820861420000597, -14.08441020739999949 ) ) ;
#23450=CARTESIAN_POINT ( 'NONE',  ( 36.78022402065349183, -79.46798840176322187, -14.63388022524676657 ) ) ;
#23451=TOROIDAL_SURFACE ( 'NONE', #7174, 30.50381168839999901, 2.000000000000000000 ) ;
#23452=CARTESIAN_POINT ( 'NONE',  ( -1.680150139059958248, -80.11422939166462243, 47.05278015009087511 ) ) ;
#23453=VERTEX_POINT ( 'NONE', #3360 ) ;
#23455=EDGE_LOOP ( 'NONE', ( #7295, #14153, #22112, #2463 ) ) ;
#23463=CARTESIAN_POINT ( 'NONE',  ( 40.34091732210000458, -74.29300278819999903, 7.252014196640000243 ) ) ;
#23466=CARTESIAN_POINT ( 'NONE',  ( 47.14083139015517787, -79.45829804079036762, -1.597024166738013840 ) ) ;
#23474=CARTESIAN_POINT ( 'NONE',  ( -2.675183968039999827E-13, -79.50000000000000000, 47.25000000000000000 ) ) ;
#23475=CARTESIAN_POINT ( 'NONE',  ( 22.42985916568536808, -18.87168151092972934, 9.783895424303356236 ) ) ;
#23477=EDGE_CURVE ( 'NONE', #14668, #27292, #101, .T. ) ;
#23481=CARTESIAN_POINT ( 'NONE',  ( 30.05801312899999900, -73.89113795069999924, -25.09024318069999993 ) ) ;
#23482=CARTESIAN_POINT ( 'NONE',  ( 7.120909764619999412E-15, -69.50000000000000000, 40.00000000000000000 ) ) ;
#23483=CARTESIAN_POINT ( 'NONE',  ( -17.94180966909999597, -72.00000000000000000, 18.81731824139999887 ) ) ;
#23485=ORIENTED_EDGE ( 'NONE', *, *, #11122, .F. ) ;
#23486=CARTESIAN_POINT ( 'NONE',  ( -40.21639064514770467, -74.12723354439698653, -7.246819345882184571 ) ) ;
#23487=CARTESIAN_POINT ( 'NONE',  ( 21.67753623600000168, -37.30770946170000002, -8.432260248800000468 ) ) ;
#23489=ORIENTED_EDGE ( 'NONE', *, *, #6922, .F. ) ;
#23490=AXIS2_PLACEMENT_3D ( 'NONE', #7789, #9667, #23231 ) ;
#23493=ORIENTED_EDGE ( 'NONE', *, *, #20265, .F. ) ;
#23495=CARTESIAN_POINT ( 'NONE',  ( -10.19002250800000020, -74.00000000000000000, 42.30193224820000353 ) ) ;
#23497=CARTESIAN_POINT ( 'NONE',  ( 9.146761579599999692, -36.52243084939999562, -22.33517371059999945 ) ) ;
#23500=EDGE_CURVE ( 'NONE', #8240, #20924, #22001, .T. ) ;
#23502=DIRECTION ( 'NONE',  ( 1.000000000000000000, 0.000000000000000000, 2.220446049250004932E-16 ) ) ;
#23503=CARTESIAN_POINT ( 'NONE',  ( 26.11117489990000351, -71.37991020869999659, 10.95904867260000159 ) ) ;
#23505=VERTEX_POINT ( 'NONE', #23590 ) ;
#23506=CIRCLE ( 'NONE', #5809, 28.68388914670000034 ) ;
#23509=CARTESIAN_POINT ( 'NONE',  ( -14.54102251839999838, -74.30694342880001102, 36.58803169640000164 ) ) ;
#23513=EDGE_CURVE ( 'NONE', #19506, #1569, #25721, .T. ) ;
#23518=CARTESIAN_POINT ( 'NONE',  ( 6.850353625200000351, -36.56979901409999911, -21.56931447779999900 ) ) ;
#23524=CARTESIAN_POINT ( 'NONE',  ( 7.344927635980000424, -35.54843156109999569, -21.39482692749999870 ) ) ;
#23525=CARTESIAN_POINT ( 'NONE',  ( 23.66024254313331454, -62.10681979203287284, 10.59952656403941162 ) ) ;
#23528=CARTESIAN_POINT ( 'NONE',  ( 19.59884367089999913, -25.54957699810000094, -8.972031911080001976 ) ) ;
#23530=ORIENTED_EDGE ( 'NONE', *, *, #27869, .F. ) ;
#23531=DIRECTION ( 'NONE',  ( 0.000000000000000000, 1.000000000000000000, 0.000000000000000000 ) ) ;
#23532=VERTEX_POINT ( 'NONE', #8268 ) ;
#23533=CARTESIAN_POINT ( 'NONE',  ( 24.78974732560000405, -64.24504771300000527, -10.08508462690000052 ) ) ;
#23534=ADVANCED_FACE ( 'NONE', ( #5944 ), #1538, .T. ) ;
#23536=CARTESIAN_POINT ( 'NONE',  ( -7.249922272500000098, -74.00000000000000000, 40.03357376780000010 ) ) ;
#23537=CIRCLE ( 'NONE', #9556, 3.000000000000002665 ) ;
#23539=EDGE_CURVE ( 'NONE', #6357, #21012, #2526, .T. ) ;
#23540=CARTESIAN_POINT ( 'NONE',  ( 27.75394116159999669, -74.50000000000000000, -27.75394116159999669 ) ) ;
#23541=CARTESIAN_POINT ( 'NONE',  ( -22.15796614980000001, -69.30519277740000916, 16.22735913770000238 ) ) ;
#23542=CARTESIAN_POINT ( 'NONE',  ( 20.49657866619999780, -57.47855601759999900, 11.20866246179999948 ) ) ;
#23543=CARTESIAN_POINT ( 'NONE',  ( -11.96164838680000031, -64.89183635400000583, -23.89138425040000158 ) ) ;
#23550=CARTESIAN_POINT ( 'NONE',  ( -2.341796741959999650, -61.59774147150000090, -24.80816657779999801 ) ) ;
#23551=B_SPLINE_CURVE_WITH_KNOTS ( 'NONE', 5,
 ( #16863, #3596, #5644, #14522, #7573, #11911 ),
 .UNSPECIFIED., .F., .F.,
 ( 6, 6 ),
 ( -66.18347591719999912, -36.59856967279999651 ),
 .UNSPECIFIED. ) ;
#23554=CARTESIAN_POINT ( 'NONE',  ( 18.94592261899999741, -19.50000000000000000, -9.024080787800000891 ) ) ;
#23556=CARTESIAN_POINT ( 'NONE',  ( 0.000000000000000000, -56.78056608349999834, 0.000000000000000000 ) ) ;
#23557=CARTESIAN_POINT ( 'NONE',  ( -7.435983481029870390, -74.13941005069941070, -39.48497135291631821 ) ) ;
#23559=CARTESIAN_POINT ( 'NONE',  ( 7.727581852389999284, -65.07443093669999712, -23.93312597839999967 ) ) ;
#23560=CARTESIAN_POINT ( 'NONE',  ( 8.969779973459999667, -35.75711592580000087, -20.13916512639999823 ) ) ;
#23561=CARTESIAN_POINT ( 'NONE',  ( 40.00441865787361451, -74.28334043028284839, 7.315281844182966786 ) ) ;
#23562=ORIENTED_EDGE ( 'NONE', *, *, #203, .F. ) ;
#23565=CARTESIAN_POINT ( 'NONE',  ( -32.31206904232557520, -74.05059202417167796, -22.10200946381351628 ) ) ;
#23566=CARTESIAN_POINT ( 'NONE',  ( -19.86043801069999759, -60.48530148380000071, 13.73936412299999965 ) ) ;
#23570=CARTESIAN_POINT ( 'NONE',  ( -2.741827583460000106, -18.87168151170000030, -24.31677564899999666 ) ) ;
#23574=CARTESIAN_POINT ( 'NONE',  ( 36.49642319969999704, -79.41084811649999153, -14.73518963879999966 ) ) ;
#23575=VERTEX_POINT ( 'NONE', #17166 ) ;
#23576=EDGE_CURVE ( 'NONE', #12207, #28514, #27908, .T. ) ;
#23579=ADVANCED_FACE ( 'NONE', ( #8143 ), #2469, .F. ) ;
#23580=VERTEX_POINT ( 'NONE', #14962 ) ;
#23585=DIRECTION ( 'NONE',  ( 0.000000000000000000, -1.000000000000000000, 0.000000000000000000 ) ) ;
#23587=EDGE_CURVE ( 'NONE', #13587, #9278, #8029, .T. ) ;
#23588=ORIENTED_EDGE ( 'NONE', *, *, #15571, .T. ) ;
#23590=CARTESIAN_POINT ( 'NONE',  ( 7.356933064080000584, -36.56811125840000187, -21.47791245320000186 ) ) ;
#23591=CARTESIAN_POINT ( 'NONE',  ( 8.597788217099999741, -37.95525409580000087, -21.87044398639999798 ) ) ;
#23593=CARTESIAN_POINT ( 'NONE',  ( 25.58626617267352898, -68.16965135175686896, 10.86867477486674183 ) ) ;
#23594=ORIENTED_EDGE ( 'NONE', *, *, #25055, .F. ) ;
#23599=CARTESIAN_POINT ( 'NONE',  ( -2.493447086729999818, -53.79621871020000157, -24.52592544210000014 ) ) ;
#23606=CARTESIAN_POINT ( 'NONE',  ( 30.54128691159999676, -72.68262309459998960, -23.69343438309999783 ) ) ;
#23609=CIRCLE ( 'NONE', #13360, 7.750000000000000000 ) ;
#23613=VERTEX_POINT ( 'NONE', #24011 ) ;
#23615=CARTESIAN_POINT ( 'NONE',  ( -40.70731707320000226, -74.50000000000000000, -7.215414233289999757 ) ) ;
#23617=CARTESIAN_POINT ( 'NONE',  ( 21.48062417799999935, -36.74237083870000475, -7.706980317549999349 ) ) ;
#23619=EDGE_CURVE ( 'NONE', #25273, #2951, #10327, .T. ) ;
#23620=ORIENTED_EDGE ( 'NONE', *, *, #10399, .T. ) ;
#23622=EDGE_CURVE ( 'NONE', #26675, #16955, #6189, .T. ) ;
#23623=B_SPLINE_SURFACE_WITH_KNOTS ( 'NONE', 5, 5, ( 
 ( #4277, #28734, #6169, #13002, #4127, #19431 ),
 ( #21912, #24526, #3990, #13295, #22199, #28315 ),
 ( #2243, #20004, #8771, #1962, #74, #8350 ),
 ( #19716, #17251, #2110, #26291, #28603, #26144 ),
 ( #12849, #10660, #19575, #28461, #8498, #17398 ),
 ( #6316, #15324, #13152, #22062, #10944, #27456 ),
 ( #22945, #24971, #20605, #26868, #4865, #24827 ),
 ( #18564, #15922, #7505, #15771, #5158, #14039 ),
 ( #11845, #18418, #27307, #17976, #13747, #9368 ) ),
 .UNSPECIFIED., .F., .F., .F.,
 ( 6, 3, 6 ),
 ( 6, 6 ),
 ( 3.884102134650000319E-15, 2.251105814029999763, 5.576980695509999642 ),
 ( 0.000000000000000000, 1.000000000000000000 ),
 .UNSPECIFIED. ) ;
#23628=CARTESIAN_POINT ( 'NONE',  ( 9.720255118479999012, -72.82938648530000592, -26.98670296669999757 ) ) ;
#23631=AXIS2_PLACEMENT_3D ( 'NONE', #96, #8368, #11868 ) ;
#23637=CARTESIAN_POINT ( 'NONE',  ( -14.14106740610000124, -74.03779068149999887, 36.36621500920000472 ) ) ;
#23640=EDGE_LOOP ( 'NONE', ( #28145, #4437, #16985, #18550 ) ) ;
#23641=CARTESIAN_POINT ( 'NONE',  ( -0.5663699853978287901, -74.35139840166131364, 47.23114592678867041 ) ) ;
#23644=LINE ( 'NONE', #25702, #27278 ) ;
#23647=CARTESIAN_POINT ( 'NONE',  ( 47.25000000000000000, -74.00000000000000000, 0.000000000000000000 ) ) ;
#23653=AXIS2_PLACEMENT_3D ( 'NONE', #21909, #4273, #10804 ) ;
#23654=CARTESIAN_POINT ( 'NONE',  ( -32.83566817730000054, -74.50000000000000000, -22.22906645950000026 ) ) ;
#23655=FACE_OUTER_BOUND ( 'NONE', #16002, .T. ) ;
#23657=DIRECTION ( 'NONE',  ( -1.000000000000000000, 0.000000000000000000, 0.000000000000000000 ) ) ;
#23662=VERTEX_POINT ( 'NONE', #18039 ) ;
#23663=DIRECTION ( 'NONE',  ( 0.000000000000000000, -1.000000000000000000, 0.000000000000000000 ) ) ;
#23665=CYLINDRICAL_SURFACE ( 'NONE', #14550, 39.24999999999998579 ) ;
#23666=ORIENTED_EDGE ( 'NONE', *, *, #17192, .T. ) ;
#23668=CARTESIAN_POINT ( 'NONE',  ( -7.296770820709999938, -74.06388275500000873, 39.69120874740000460 ) ) ;
#23673=AXIS2_PLACEMENT_3D ( 'NONE', #10379, #19017, #27897 ) ;
#23675=CARTESIAN_POINT ( 'NONE',  ( -12.15457518680000071, -65.52795386159999680, -22.48391257200000126 ) ) ;
#23676=CARTESIAN_POINT ( 'NONE',  ( 7.217842745160000462, -35.78513210170000036, -21.44331575660000055 ) ) ;
#23680=ADVANCED_FACE ( 'NONE', ( #15546 ), #6850, .T. ) ;
#23682=ADVANCED_FACE ( 'NONE', ( #19775 ), #28656, .F. ) ;
#23683=CARTESIAN_POINT ( 'NONE',  ( -2.485331911600000332, -61.52579421249999569, -25.06050290059999952 ) ) ;
#23684=TOROIDAL_SURFACE ( 'NONE', #4618, 12.00000000000000000, 1.000000000000000000 ) ;
#23685=CARTESIAN_POINT ( 'NONE',  ( 9.322992499379999742, -37.99098076110000477, -22.72991278869999832 ) ) ;
#23689=AXIS2_PLACEMENT_3D ( 'NONE', #15245, #6537, #6833 ) ;
#23692=VERTEX_POINT ( 'NONE', #13218 ) ;
#23693=PLANE ( 'NONE',  #27484 ) ;
#23695=CARTESIAN_POINT ( 'NONE',  ( 7.691701944196837282, -37.38596123215534561, -21.51611381909645715 ) ) ;
#23697=CARTESIAN_POINT ( 'NONE',  ( -14.01337416149999981, -80.34292142019999972, 36.66316733609999545 ) ) ;
#23698=CARTESIAN_POINT ( 'NONE',  ( -22.16250285911532814, -74.14342904296044878, -32.55991892830125778 ) ) ;
#23699=CARTESIAN_POINT ( 'NONE',  ( 22.02359273509999937, -18.62181730670000235, 9.222605046309999111 ) ) ;
#23703=ORIENTED_EDGE ( 'NONE', *, *, #7512, .T. ) ;
#23704=CARTESIAN_POINT ( 'NONE',  ( -9.356041104380000917, -84.00000000000000000, 37.60355029590000697 ) ) ;
#23706=CARTESIAN_POINT ( 'NONE',  ( -0.5590517731190000061, -18.50000000000000000, -21.02688049580000040 ) ) ;
#23710=AXIS2_PLACEMENT_3D ( 'NONE', #23556, #14518, #19046 ) ;
#23713=CARTESIAN_POINT ( 'NONE',  ( 36.67694313739999501, -80.46520755129999714, -13.97975614370000130 ) ) ;
#23714=EDGE_LOOP ( 'NONE', ( #25259, #1217, #22691, #6832 ) ) ;
#23715=EDGE_CURVE ( 'NONE', #14159, #5527, #3257, .T. ) ;
#23716=EDGE_CURVE ( 'NONE', #7833, #26140, #2890, .T. ) ;
#23719=CARTESIAN_POINT ( 'NONE',  ( -7.215414233289999757, -77.00000000000000000, -40.70731707320000226 ) ) ;
#23722=CARTESIAN_POINT ( 'NONE',  ( 47.16762437949999764, -74.53411049070001582, -1.089894286769999887 ) ) ;
#23724=CARTESIAN_POINT ( 'NONE',  ( 23.11751862730000084, -56.19735282230000450, 10.36524394209999933 ) ) ;
#23725=CARTESIAN_POINT ( 'NONE',  ( 20.82957722363834918, -36.00000000010000178, -9.510883242529262205 ) ) ;
#23726=CARTESIAN_POINT ( 'NONE',  ( -7.135467526410000261, -73.65707963269998970, -38.71641004229999794 ) ) ;
#23729=DIRECTION ( 'NONE',  ( 0.000000000000000000, -1.000000000000000000, 0.000000000000000000 ) ) ;
#23732=FACE_OUTER_BOUND ( 'NONE', #28272, .T. ) ;
#23733=CARTESIAN_POINT ( 'NONE',  ( -2.557399843751114954, -79.91561779696330348, 47.03678055220303378 ) ) ;
#23734=VERTEX_POINT ( 'NONE', #7571 ) ;
#23735=CARTESIAN_POINT ( 'NONE',  ( 25.12979114312568285, -65.01951069083045809, 0.1513711869631185758 ) ) ;
#23737=DIRECTION ( 'NONE',  ( -0.7071067811865474617, 0.000000000000000000, -0.7071067811865474617 ) ) ;
#23740=VERTEX_POINT ( 'NONE', #14107 ) ;
#23743=CARTESIAN_POINT ( 'NONE',  ( -18.28907245470000120, -18.50000000000000000, 14.67141105099999976 ) ) ;
#23744=ORIENTED_EDGE ( 'NONE', *, *, #574, .T. ) ;
#23748=CARTESIAN_POINT ( 'NONE',  ( 21.63858029419999696, -18.50000000000000000, 8.493246274499998805 ) ) ;
#23750=CARTESIAN_POINT ( 'NONE',  ( 26.61374759190000105, -73.81001964159999318, -28.89513312169999892 ) ) ;
#23756=ORIENTED_EDGE ( 'NONE', *, *, #993, .F. ) ;
#23757=CARTESIAN_POINT ( 'NONE',  ( -39.83391879159715643, -73.87273571728266575, -7.248098695806580949 ) ) ;
#23759=CARTESIAN_POINT ( 'NONE',  ( 20.97515210950000153, -36.16091267649999708, -8.638070979520000137 ) ) ;
#23760=CARTESIAN_POINT ( 'NONE',  ( 9.151216319970000512, -35.87888623290000112, -19.56023227720000079 ) ) ;
#23766=CARTESIAN_POINT ( 'NONE',  ( 7.992697997670000554, -57.47158989559999753, -22.16162922080000186 ) ) ;
#23768=ORIENTED_EDGE ( 'NONE', *, *, #4464, .F. ) ;
#23771=TOROIDAL_SURFACE ( 'NONE', #13534, 10.50000000000000000, 0.5000000000000000000 ) ;
#23772=CARTESIAN_POINT ( 'NONE',  ( 22.38048301969999798, -27.06679042429999882, 0.1658473372300000026 ) ) ;
#23773=DIRECTION ( 'NONE',  ( 1.000000000000000000, 0.000000000000000000, 0.000000000000000000 ) ) ;
#23775=CARTESIAN_POINT ( 'NONE',  ( 19.35192606849999919, -18.86754463369999968, -8.857879772089999548 ) ) ;
#23778=CARTESIAN_POINT ( 'NONE',  ( -14.40064467200000209, -74.16918790970001396, 36.61749309489999860 ) ) ;
#23781=ORIENTED_EDGE ( 'NONE', *, *, #24472, .T. ) ;
#23782=EDGE_CURVE ( 'NONE', #6426, #17770, #11299, .T. ) ;
#23786=CARTESIAN_POINT ( 'NONE',  ( 7.999569604760000452, -65.05903923030000158, -23.83793848660000236 ) ) ;
#23787=CARTESIAN_POINT ( 'NONE',  ( -13.18623751009999978, -69.39685719070000403, -23.69831535020000146 ) ) ;
#23789=CARTESIAN_POINT ( 'NONE',  ( 23.14416773940000027, -57.40875670289999988, 10.37855713959999981 ) ) ;
#23790=CARTESIAN_POINT ( 'NONE',  ( -10.84622327880000014, -27.00851495050000040, -21.73428641559999974 ) ) ;
#23791=ORIENTED_EDGE ( 'NONE', *, *, #27656, .F. ) ;
#23799=CARTESIAN_POINT ( 'NONE',  ( 8.963581071920001975, -35.44265712969999527, -20.01429396089999813 ) ) ;
#23800=CARTESIAN_POINT ( 'NONE',  ( 21.09786747150000252, -18.50000000000000000, 0.1832040240040000156 ) ) ;
#23808=ORIENTED_EDGE ( 'NONE', *, *, #297, .F. ) ;
#23810=CARTESIAN_POINT ( 'NONE',  ( -38.71640881029999548, -73.50000064450000536, -7.135467304789999687 ) ) ;
#23811=CARTESIAN_POINT ( 'NONE',  ( 36.62466543095905536, -74.65121096129686862, -14.68734462481934600 ) ) ;
#23817=CARTESIAN_POINT ( 'NONE',  ( 46.25000000000000000, -75.00000000000000000, -13.75000000000000000 ) ) ;
#23818=CARTESIAN_POINT ( 'NONE',  ( -18.68796107978499776, -19.47636826820795264, 13.44054024894182042 ) ) ;
#23819=CARTESIAN_POINT ( 'NONE',  ( -10.50797418640000025, -18.50000000000000000, 18.24753908359999954 ) ) ;
#23822=CARTESIAN_POINT ( 'NONE',  ( 8.522376746440000872, -19.16582662329999920, -20.19515292700000231 ) ) ;
#23824=CARTESIAN_POINT ( 'NONE',  ( -40.00000000000000000, -74.50000000000000000, 2.464695114669999848E-15 ) ) ;
#23826=CARTESIAN_POINT ( 'NONE',  ( 6.948750312308070498, -36.56992522833583337, -21.53806854013285133 ) ) ;
#23827=B_SPLINE_CURVE_WITH_KNOTS ( 'NONE', 3,
 ( #18832, #18538, #11518, #20425 ),
 .UNSPECIFIED., .F., .F.,
 ( 4, 4 ),
 ( 0.000000000000000000, 1.000000000000000000 ),
 .UNSPECIFIED. ) ;
#23828=DIRECTION ( 'NONE',  ( 1.000000000000000000, 0.000000000000000000, 1.110223024629999160E-15 ) ) ;
#23829=AXIS2_PLACEMENT_3D ( 'NONE', #22219, #9093, #9235 ) ;
#23830=DIRECTION ( 'NONE',  ( 1.000000000000000000, 0.000000000000000000, 0.000000000000000000 ) ) ;
#23832=ORIENTED_EDGE ( 'NONE', *, *, #9403, .F. ) ;
#23833=CARTESIAN_POINT ( 'NONE',  ( 21.49951961919999732, -36.15937190469999507, -7.044630138860000557 ) ) ;
#23836=CARTESIAN_POINT ( 'NONE',  ( -14.25825325729999982, -80.34252531600000680, 36.56956972409999906 ) ) ;
#23838=ADVANCED_FACE ( 'NONE', ( #13147 ), #28730, .T. ) ;
#23840=CARTESIAN_POINT ( 'NONE',  ( -32.79293189096514283, -74.34878806649766148, -22.21871444800659035 ) ) ;
#23841=CARTESIAN_POINT ( 'NONE',  ( -20.56018215729999810, -57.40875686090000585, 14.85415973970000003 ) ) ;
#23843=AXIS2_PLACEMENT_3D ( 'NONE', #19761, #9385, #24986 ) ;
#23844=CIRCLE ( 'NONE', #28058, 39.25000000000000000 ) ;
#23850=ORIENTED_EDGE ( 'NONE', *, *, #12962, .F. ) ;
#23851=ADVANCED_FACE ( 'NONE', ( #8768 ), #12457, .T. ) ;
#23853=CARTESIAN_POINT ( 'NONE',  ( -32.08679448059999828, -74.00994675159999758, -21.96941954280000076 ) ) ;
#23854=CARTESIAN_POINT ( 'NONE',  ( 36.29172732829999859, -79.24889011169999264, -14.94947765220000058 ) ) ;
#23856=B_SPLINE_SURFACE_WITH_KNOTS ( 'NONE', 5, 5, ( 
 ( #1465, #14964, #12778, #6237, #21827, #1883 ),
 ( #10721, #19635, #14698, #17463, #26349, #15241 ),
 ( #24160, #4194, #1325, #10167, #19086, #23591 ),
 ( #8009, #3635, #9286, #22265, #2313, #11166 ),
 ( #24452, #21978, #19777, #11321, #8690, #15844 ),
 ( #20369, #13362, #20080, #27083, #24305, #20225 ) ),
 .UNSPECIFIED., .F., .F., .F.,
 ( 6, 6 ),
 ( 6, 6 ),
 ( 2.709627234730000112, 3.225498864409999999 ),
 ( 0.000000000000000000, 2.000000000000000000 ),
 .UNSPECIFIED. ) ;
#23858=CARTESIAN_POINT ( 'NONE',  ( 36.70830968599999977, -79.00000000000000000, -14.75000000000000000 ) ) ;
#23860=CARTESIAN_POINT ( 'NONE',  ( -3.306822307565103536, -80.49999980012920275, 46.45859196424991211 ) ) ;
#23862=ADVANCED_FACE ( 'NONE', ( #15318 ), #27631, .T. ) ;
#23863=DIRECTION ( 'NONE',  ( 0.000000000000000000, -1.000000000000000000, 0.000000000000000000 ) ) ;
#23864=CARTESIAN_POINT ( 'NONE',  ( 46.60312383370383316, -73.73419539363156616, -2.997193309239198467 ) ) ;
#23866=AXIS2_PLACEMENT_3D ( 'NONE', #27793, #3325, #8108 ) ;
#23868=CARTESIAN_POINT ( 'NONE',  ( 47.25000000000000000, -75.00000000000000000, -7.375000000000000000 ) ) ;
#23871=AXIS2_PLACEMENT_3D ( 'NONE', #21866, #4084, #12953 ) ;
#23873=CARTESIAN_POINT ( 'NONE',  ( 6.015370493379999656E-15, -69.00000000000000000, -40.00000000000000000 ) ) ;
#23875=DIRECTION ( 'NONE',  ( 0.000000000000000000, -1.000000000000000000, 0.000000000000000000 ) ) ;
#23881=ADVANCED_FACE ( 'NONE', ( #26425 ), #2439, .T. ) ;
#23885=CARTESIAN_POINT ( 'NONE',  ( -0.5350069560319999917, -53.84434310269999457, -23.22809113779999990 ) ) ;
#23887=CARTESIAN_POINT ( 'NONE',  ( 10.27942207598835012, -72.70273852363769151, -26.82731210389089327 ) ) ;
#23889=ORIENTED_EDGE ( 'NONE', *, *, #5502, .T. ) ;
#23890=CARTESIAN_POINT ( 'NONE',  ( 2.042810365310000056E-12, -74.50000000000000000, -2.458477865729999957E-12 ) ) ;
#23891=CARTESIAN_POINT ( 'NONE',  ( -19.11827583450000034, -19.41837863929999841, 14.08667248819999962 ) ) ;
#23893=CARTESIAN_POINT ( 'NONE',  ( 22.43858155039999858, -18.50000000000000000, 8.750340092050000962 ) ) ;
#23897=CIRCLE ( 'NONE', #25391, 3.750000000000000000 ) ;
#23902=CARTESIAN_POINT ( 'NONE',  ( 19.85335301099999938, -35.79755265089999483, -9.067520686860000012 ) ) ;
#23903=CARTESIAN_POINT ( 'NONE',  ( 9.212446728010000641, -35.92148816550000134, -19.60212694180000170 ) ) ;
#23909=CARTESIAN_POINT ( 'NONE',  ( 20.36793921129758900, -34.63244748723148092, -8.805019764629991030 ) ) ;
#23911=CARTESIAN_POINT ( 'NONE',  ( -34.11790219230000076, -80.00000000000000000, -24.21840725559999896 ) ) ;
#23913=ORIENTED_EDGE ( 'NONE', *, *, #9345, .T. ) ;
#23915=CARTESIAN_POINT ( 'NONE',  ( 23.99279226960000244, -42.23583340129999897, 1.251023842240000183 ) ) ;
#23916=CARTESIAN_POINT ( 'NONE',  ( 23.67408170059999861, -68.20869413019998717, 12.08289283440000084 ) ) ;
#23918=VERTEX_POINT ( 'NONE', #3124 ) ;
#23919=DIRECTION ( 'NONE',  ( 1.000000000000000000, 0.000000000000000000, 0.000000000000000000 ) ) ;
#23922=DIRECTION ( 'NONE',  ( 0.000000000000000000, 1.000000000000000000, 0.000000000000000000 ) ) ;
#23924=ORIENTED_EDGE ( 'NONE', *, *, #23500, .T. ) ;
#23925=CARTESIAN_POINT ( 'NONE',  ( 28.60859787209999894, -72.37489962920000153, 2.608048168490000318 ) ) ;
#23928=CARTESIAN_POINT ( 'NONE',  ( 8.613456916169999644, -58.97932910050000288, -22.38225487870000308 ) ) ;
#23929=CARTESIAN_POINT ( 'NONE',  ( -12.23046582149999928, -69.33507195810000212, -24.60464239079999871 ) ) ;
#23930=CARTESIAN_POINT ( 'NONE',  ( 22.73387075099999777, -60.10032509980000270, 10.25825663050000003 ) ) ;
#23931=CARTESIAN_POINT ( 'NONE',  ( -11.11926074269999987, -19.46548176030000121, -19.02542913479999953 ) ) ;
#23932=EDGE_LOOP ( 'NONE', ( #4280, #3260 ) ) ;
#23936=CARTESIAN_POINT ( 'NONE',  ( 3.907985046679999924E-15, -73.50000000000000000, -40.00000000000000000 ) ) ;
#23937=CARTESIAN_POINT ( 'NONE',  ( -40.00000000000000000, -79.00000000000000000, 0.000000000000000000 ) ) ;
#23938=TOROIDAL_SURFACE ( 'NONE', #27693, 6.750000000000000000, 0.5000000000000000000 ) ;
#23939=DIRECTION ( 'NONE',  ( 0.000000000000000000, -1.000000000000000000, 0.000000000000000000 ) ) ;
#23943=B_SPLINE_CURVE_WITH_KNOTS ( 'NONE', 5,
 ( #25312, #2724, #7544, #22539, #2584, #20487 ),
 .UNSPECIFIED., .F., .F.,
 ( 6, 6 ),
 ( 0.000000000000000000, 1.000000000000000000 ),
 .UNSPECIFIED. ) ;
#23946=ORIENTED_EDGE ( 'NONE', *, *, #8641, .T. ) ;
#23947=CIRCLE ( 'NONE', #11867, 0.9999999999999996669 ) ;
#23948=DIRECTION ( 'NONE',  ( 1.000000000000000000, 0.000000000000000000, 7.486357007659991815E-17 ) ) ;
#23956=CARTESIAN_POINT ( 'NONE',  ( -3.252988965690000178, -72.00000000000000000, -30.32986301179999700 ) ) ;
#23957=DIRECTION ( 'NONE',  ( 0.000000000000000000, -1.000000000000000000, 0.000000000000000000 ) ) ;
#23960=DIRECTION ( 'NONE',  ( -0.3388747807339287932, -0.000000000000000000, -0.9408314849018032389 ) ) ;
#23963=DIRECTION ( 'NONE',  ( 0.000000000000000000, -1.000000000000000000, 0.000000000000000000 ) ) ;
#23964=CARTESIAN_POINT ( 'NONE',  ( 7.351926511809999454, -36.21205854349999953, -21.46601197540000072 ) ) ;
#23965=DIRECTION ( 'NONE',  ( 1.000000000000000000, 0.000000000000000000, 0.000000000000000000 ) ) ;
#23967=CARTESIAN_POINT ( 'NONE',  ( 8.815784351519999618, -19.48264119070000078, -19.82501765289999796 ) ) ;
#23968=CARTESIAN_POINT ( 'NONE',  ( -13.85848666890000125, -57.40875702409999803, 21.24403892489999990 ) ) ;
#23969=CARTESIAN_POINT ( 'NONE',  ( -2.790536552329999864, -64.24504439390000243, -26.36014980279999875 ) ) ;
#23970=CARTESIAN_POINT ( 'NONE',  ( 10.68317386900000088, -36.00000000000000000, -21.62249396890000241 ) ) ;
#23972=CARTESIAN_POINT ( 'NONE',  ( -19.84037407199999947, -55.01779585689999408, 14.17763065249999954 ) ) ;
#23977=CARTESIAN_POINT ( 'NONE',  ( 19.97576656849999921, -35.50000000000000000, -19.97576656849999921 ) ) ;
#23978=ORIENTED_EDGE ( 'NONE', *, *, #22206, .T. ) ;
#23979=EDGE_CURVE ( 'NONE', #6426, #5907, #11840, .T. ) ;
#23981=EDGE_CURVE ( 'NONE', #23613, #12242, #11767, .T. ) ;
#23982=CARTESIAN_POINT ( 'NONE',  ( 5.329070518200000398E-15, -74.50000000000000000, 0.000000000000000000 ) ) ;
#23983=CIRCLE ( 'NONE', #11413, 22.61111346610000084 ) ;
#23984=CARTESIAN_POINT ( 'NONE',  ( -22.18442533826599217, -74.19997306779613666, -32.65038183209173184 ) ) ;
#23985=CARTESIAN_POINT ( 'NONE',  ( 22.19631186670000034, -18.86932112550000085, 9.599616484340000255 ) ) ;
#23986=CARTESIAN_POINT ( 'NONE',  ( -32.75544218747561587, -74.29667472474076817, -22.20975189080888867 ) ) ;
#23989=SPHERICAL_SURFACE ( 'NONE', #26462, 2.000000000000000000 ) ;
#23991=DIRECTION ( 'NONE',  ( 0.000000000000000000, -1.000000000000000000, 0.000000000000000000 ) ) ;
#23993=EDGE_LOOP ( 'NONE', ( #14867, #28192, #12226, #17384 ) ) ;
#23995=CARTESIAN_POINT ( 'NONE',  ( -25.98617420859999783, -79.50000000000000000, -36.59277592640000165 ) ) ;
#23996=CARTESIAN_POINT ( 'NONE',  ( 37.14872973290000147, -79.99999989399999833, -13.69566407600000169 ) ) ;
#23998=EDGE_CURVE ( 'NONE', #5681, #26675, #14111, .T. ) ;
#24000=CIRCLE ( 'NONE', #3103, 39.25000000000000000 ) ;
#24002=ORIENTED_EDGE ( 'NONE', *, *, #1884, .F. ) ;
#24005=CARTESIAN_POINT ( 'NONE',  ( 21.60392450109999984, -56.24740423709999249, 10.18205705279999940 ) ) ;
#24008=ORIENTED_EDGE ( 'NONE', *, *, #27228, .F. ) ;
#24011=CARTESIAN_POINT ( 'NONE',  ( 3.459338121946999694E-15, -74.00000000000000000, -32.25000000000000000 ) ) ;
#24012=ADVANCED_FACE ( 'NONE', ( #25271 ), #22442, .T. ) ;
#24014=CARTESIAN_POINT ( 'NONE',  ( -21.70609662629999903, -80.13404657770000483, -32.70204620079999813 ) ) ;
#24016=CARTESIAN_POINT ( 'NONE',  ( 26.13974465595868679, -69.66091081680940533, 10.83115750005767097 ) ) ;
#24021=CARTESIAN_POINT ( 'NONE',  ( -2.578307999469999778, -52.56313962730000355, -25.11373953509999879 ) ) ;
#24023=CARTESIAN_POINT ( 'NONE',  ( 11.37934278408159194, -72.27101671311534403, -27.01370042787952030 ) ) ;
#24024=CARTESIAN_POINT ( 'NONE',  ( -19.73459501870000210, -19.50000008899999671, 14.41863475499999936 ) ) ;
#24025=ORIENTED_EDGE ( 'NONE', *, *, #12765, .T. ) ;
#24032=ORIENTED_EDGE ( 'NONE', *, *, #4475, .T. ) ;
#24033=ADVANCED_FACE ( 'NONE', ( #25956 ), #12529, .T. ) ;
#24036=CARTESIAN_POINT ( 'NONE',  ( 21.55284568440000115, -37.11646645979999448, -8.225667895000000840 ) ) ;
#24037=CARTESIAN_POINT ( 'NONE',  ( 9.056984553609998656, -35.76308213440000117, -19.54972227260000039 ) ) ;
#24038=ORIENTED_EDGE ( 'NONE', *, *, #17123, .T. ) ;
#24039=EDGE_CURVE ( 'NONE', #22913, #23692, #20952, .T. ) ;
#24042=CARTESIAN_POINT ( 'NONE',  ( -3.281858763419757352, -67.67702679679626954, -27.44020346820908074 ) ) ;
#24046=CARTESIAN_POINT ( 'NONE',  ( 7.914382952159999540, -49.10861551380000378, -21.88571563610000226 ) ) ;
#24047=CARTESIAN_POINT ( 'NONE',  ( -11.17631027600000060, -19.46429362099999949, -18.99082252140000193 ) ) ;
#24048=ORIENTED_EDGE ( 'NONE', *, *, #8300, .F. ) ;
#24050=CARTESIAN_POINT ( 'NONE',  ( 24.63152983679999863, -42.21394486829999693, 1.405087790390000091 ) ) ;
#24051=CARTESIAN_POINT ( 'NONE',  ( 24.74138143300000081, -65.80499425489999510, 10.85530572179999886 ) ) ;
#24053=EDGE_LOOP ( 'NONE', ( #17578, #3955, #8583, #24569, #21124, #11282, #14596, #16831, #9177, #10790 ) ) ;
#24054=CARTESIAN_POINT ( 'NONE',  ( -38.65569705749999940, -74.00000000000000000, 7.472970580910000216 ) ) ;
#24055=CARTESIAN_POINT ( 'NONE',  ( -20.49364000779999984, -54.17834560379999687, 14.81079386229999884 ) ) ;
#24059=( GEOMETRIC_REPRESENTATION_CONTEXT ( 3 ) GLOBAL_UNCERTAINTY_ASSIGNED_CONTEXT ( ( #14413 ) ) GLOBAL_UNIT_ASSIGNED_CONTEXT ( ( #1808, #21623, #5882 ) ) REPRESENTATION_CONTEXT ( 'NONE', 'WORKASPACE' ) );
#24060=CARTESIAN_POINT ( 'NONE',  ( 26.64667737100000267, -68.06111685179999427, 1.045328632849999995 ) ) ;
#24061=EDGE_CURVE ( 'NONE', #28564, #27146, #20152, .T. ) ;
#24063=CARTESIAN_POINT ( 'NONE',  ( 7.555863278439999497, -62.13670074319999515, -22.76391182080000064 ) ) ;
#24070=TOROIDAL_SURFACE ( 'NONE', #18971, 7.750000000000000000, 0.5000000000000000000 ) ;
#24073=CARTESIAN_POINT ( 'NONE',  ( 8.366907574789999913, -35.47960661259999426, -21.01624086869999886 ) ) ;
#24074=CARTESIAN_POINT ( 'NONE',  ( 23.75187361598589675, -62.52448827938915343, 10.63125306484759847 ) ) ;
#24075=CARTESIAN_POINT ( 'NONE',  ( 2.842170943039999687E-14, -72.00000000000000000, 1.776356839399999804E-15 ) ) ;
#24078=CIRCLE ( 'NONE', #6899, 38.75000000000000000 ) ;
#24082=EDGE_CURVE ( 'NONE', #13829, #19768, #7630, .T. ) ;
#24083=CARTESIAN_POINT ( 'NONE',  ( -38.08875739639999836, -82.25000000000000000, -9.476764215410000247 ) ) ;
#24085=VERTEX_POINT ( 'NONE', #23628 ) ;
#24086=CARTESIAN_POINT ( 'NONE',  ( 7.403496485329999821, -36.74765514679999967, -21.48174179600000144 ) ) ;
#24092=TOROIDAL_SURFACE ( 'NONE', #19434, 6.750000000000000000, 0.5000000000000000000 ) ;
#24099=B_SPLINE_CURVE_WITH_KNOTS ( 'NONE', 3,
 ( #4375, #322, #26824, #20402 ),
 .UNSPECIFIED., .F., .F.,
 ( 4, 4 ),
 ( 0.000000000000000000, 1.000000000000000000 ),
 .UNSPECIFIED. ) ;
#24100=CARTESIAN_POINT ( 'NONE',  ( 36.51232682552267050, -75.00000020506665521, -14.77966825339260382 ) ) ;
#24101=CARTESIAN_POINT ( 'NONE',  ( -18.49652135632734584, -19.46608320370290102, 12.36970486431163074 ) ) ;
#24104=CARTESIAN_POINT ( 'NONE',  ( 19.43643804750000115, -34.66800313659999944, -8.988996126470000902 ) ) ;
#24108=AXIS2_PLACEMENT_3D ( 'NONE', #12502, #18823, #7880 ) ;
#24109=CARTESIAN_POINT ( 'NONE',  ( 21.22142466270000227, -36.00000000000000000, -10.41046144799999951 ) ) ;
#24110=EDGE_CURVE ( 'NONE', #23575, #26844, #16895, .T. ) ;
#24111=CARTESIAN_POINT ( 'NONE',  ( -2.343981719409999886, -60.15167146970000545, -24.54744736600000010 ) ) ;
#24112=ORIENTED_EDGE ( 'NONE', *, *, #20468, .T. ) ;
#24113=CARTESIAN_POINT ( 'NONE',  ( 9.649489330299999779, -36.18102153040000246, -21.30683186290000108 ) ) ;
#24115=CARTESIAN_POINT ( 'NONE',  ( -19.65423707410000276, -57.45864773929999814, 13.63538719409999977 ) ) ;
#24118=CARTESIAN_POINT ( 'NONE',  ( 21.28939746550000223, -35.22612253230000334, -7.745600858799999600 ) ) ;
#24119=CARTESIAN_POINT ( 'NONE',  ( 7.260235792919999653, -73.97913911329999337, -40.03809227349999844 ) ) ;
#24120=ORIENTED_EDGE ( 'NONE', *, *, #14425, .F. ) ;
#24121=CARTESIAN_POINT ( 'NONE',  ( 7.923880834827633279, -37.75688408617100578, -21.55540859128345232 ) ) ;
#24122=AXIS2_PLACEMENT_3D ( 'NONE', #16556, #10253, #5619 ) ;
#24124=AXIS2_PLACEMENT_3D ( 'NONE', #25913, #23585, #25264 ) ;
#24125=CARTESIAN_POINT ( 'NONE',  ( -9.493551874750000508, -18.50000000000000000, -20.00161470729999991 ) ) ;
#24128=CARTESIAN_POINT ( 'NONE',  ( -32.61798281429999946, -80.00000000000000000, -22.71848787769999944 ) ) ;
#24130=ORIENTED_EDGE ( 'NONE', *, *, #9937, .F. ) ;
#24131=CARTESIAN_POINT ( 'NONE',  ( 30.45033996220000105, -72.00000000000000000, 1.805359716810000181 ) ) ;
#24134=DIRECTION ( 'NONE',  ( 1.000000000000000000, 0.000000000000000000, 0.000000000000000000 ) ) ;
#24136=ORIENTED_EDGE ( 'NONE', *, *, #24442, .T. ) ;
#24138=B_SPLINE_CURVE_WITH_KNOTS ( 'NONE', 5,
 ( #3929, #4364, #26510, #23893, #15413, #23748, #13236, #21846, #12793, #13087, #26364, #6393, #25938, #21701, #17187, #8288, #10738, #5962 ),
 .UNSPECIFIED., .F., .F.,
 ( 6, 3, 3, 3, 3, 6 ),
 ( 0.000000000000000000, 1.124498255640000055, 2.252774941560000244, 3.380756636310000118, 4.508382774220000222, 5.576981603820000188 ),
 .UNSPECIFIED. ) ;
#24139=VECTOR ( 'NONE', #28203, 1000.000000000000000 ) ;
#24141=CARTESIAN_POINT ( 'NONE',  ( -32.08195032130000612, -74.00665451570000641, -21.91676683800000092 ) ) ;
#24142=CARTESIAN_POINT ( 'NONE',  ( 36.88485589580000124, -80.18584060519999923, -13.59838148100000055 ) ) ;
#24143=ORIENTED_EDGE ( 'NONE', *, *, #22380, .T. ) ;
#24144=EDGE_CURVE ( 'NONE', #15756, #7849, #13642, .T. ) ;
#24149=CARTESIAN_POINT ( 'NONE',  ( 27.89292634430000106, -72.00000000000000000, 12.34776042340000046 ) ) ;
#24153=EDGE_LOOP ( 'NONE', ( #10418, #26625, #18236 ) ) ;
#24155=DIRECTION ( 'NONE',  ( 1.000000000000000000, 0.000000000000000000, 1.225073682349999956E-16 ) ) ;
#24156=ORIENTED_EDGE ( 'NONE', *, *, #8275, .F. ) ;
#24158=CARTESIAN_POINT ( 'NONE',  ( 20.49657866619999780, -57.47855601759999900, 11.20866246179999948 ) ) ;
#24159=AXIS2_PLACEMENT_3D ( 'NONE', #25836, #23922, #10625 ) ;
#24160=CARTESIAN_POINT ( 'NONE',  ( 9.726843560609999884, -36.00000000000000000, -20.21912206349999863 ) ) ;
#24162=CARTESIAN_POINT ( 'NONE',  ( -3.190509958379999844, -18.50000000000000000, -22.41471204839999842 ) ) ;
#24165=AXIS2_PLACEMENT_3D ( 'NONE', #14704, #10725, #28384 ) ;
#24172=DIRECTION ( 'NONE',  ( 0.000000000000000000, 0.000000000000000000, -1.000000000000000000 ) ) ;
#24177=CARTESIAN_POINT ( 'NONE',  ( 22.35420107259999867, -19.50000000000000000, 9.881343484100000296 ) ) ;
#24182=DIRECTION ( 'NONE',  ( 6.123031769109993025E-17, 0.000000000000000000, -1.000000000000000000 ) ) ;
#24185=VERTEX_POINT ( 'NONE', #30 ) ;
#24189=CARTESIAN_POINT ( 'NONE',  ( 21.56715281920000038, -37.71255813250000699, -7.938702241180000563 ) ) ;
#24196=ORIENTED_EDGE ( 'NONE', *, *, #5972, .T. ) ;
#24199=CARTESIAN_POINT ( 'NONE',  ( 8.600016955360000992, -57.45905992459999823, -22.33353630010000046 ) ) ;
#24203=DIRECTION ( 'NONE',  ( 0.4794255386042040046, 0.000000000000000000, 0.8775825618903722036 ) ) ;
#24204=CARTESIAN_POINT ( 'NONE',  ( 25.02058468999999974, -57.41946978100000365, 1.375913977570000002 ) ) ;
#24206=CARTESIAN_POINT ( 'NONE',  ( 39.22862632788639559, -73.58711170886084574, 7.208933142618684897 ) ) ;
#24207=ORIENTED_EDGE ( 'NONE', *, *, #18163, .F. ) ;
#24208=LINE ( 'NONE', #2211, #26228 ) ;
#24212=AXIS2_PLACEMENT_3D ( 'NONE', #2193, #24631, #15578 ) ;
#24214=CARTESIAN_POINT ( 'NONE',  ( -40.00000000000000000, -73.50000000000000000, 3.397282455350000038E-15 ) ) ;
#24219=CARTESIAN_POINT ( 'NONE',  ( 23.50166587800000073, -64.58097839929999395, 10.73601817129999958 ) ) ;
#24220=CARTESIAN_POINT ( 'NONE',  ( 22.74072897519999970, -62.08051493450000180, -8.166369310169999451 ) ) ;
#24222=DIRECTION ( 'NONE',  ( 1.000000000000000000, 0.000000000000000000, 0.000000000000000000 ) ) ;
#24223=ORIENTED_EDGE ( 'NONE', *, *, #14726, .F. ) ;
#24225=CARTESIAN_POINT ( 'NONE',  ( 23.57414836690000115, -18.50000000000000000, 2.476549100839999795 ) ) ;
#24228=CIRCLE ( 'NONE', #13035, 10.49999999999999822 ) ;
#24230=CIRCLE ( 'NONE', #1453, 4.750000000000000888 ) ;
#24232=EDGE_CURVE ( 'NONE', #7043, #19169, #21599, .T. ) ;
#24237=ORIENTED_EDGE ( 'NONE', *, *, #3971, .F. ) ;
#24238=CARTESIAN_POINT ( 'NONE',  ( 8.862965437350000641, -35.80913068480000305, -20.41714882420000166 ) ) ;
#24244=ORIENTED_EDGE ( 'NONE', *, *, #1331, .F. ) ;
#24246=CARTESIAN_POINT ( 'NONE',  ( -13.65271896930000040, -18.62222160940000037, 19.81146398099999928 ) ) ;
#24248=ADVANCED_FACE ( 'NONE', ( #18522 ), #7150, .F. ) ;
#24250=CARTESIAN_POINT ( 'NONE',  ( -15.46523628789999982, -74.50000000000000000, 38.98408025979999536 ) ) ;
#24251=CARTESIAN_POINT ( 'NONE',  ( 25.66698395754550077, -60.96609256304353153, 1.396244422503700955 ) ) ;
#24252=CARTESIAN_POINT ( 'NONE',  ( 7.456866166569999343, -35.46743057900000196, -21.37275087869999624 ) ) ;
#24254=AXIS2_PLACEMENT_3D ( 'NONE', #13118, #12822, #10917 ) ;
#24256=AXIS2_PLACEMENT_3D ( 'NONE', #2571, #26896, #6933 ) ;
#24257=FACE_OUTER_BOUND ( 'NONE', #10197, .T. ) ;
#24258=AXIS2_PLACEMENT_3D ( 'NONE', #20864, #1203, #27836 ) ;
#24259=CARTESIAN_POINT ( 'NONE',  ( 21.60058908400000277, -36.18196428190000091, -9.926413990670001297 ) ) ;
#24260=CARTESIAN_POINT ( 'NONE',  ( -11.47801891529999985, -59.03823354080000740, 20.41172223289999721 ) ) ;
#24262=CARTESIAN_POINT ( 'NONE',  ( -19.68646692119999742, -57.47571038090000428, 12.70082239459999940 ) ) ;
#24264=ORIENTED_EDGE ( 'NONE', *, *, #24373, .T. ) ;
#24269=DIRECTION ( 'NONE',  ( 0.000000000000000000, -1.000000000000000000, 0.000000000000000000 ) ) ;
#24272=CARTESIAN_POINT ( 'NONE',  ( 7.010390260919999428E-15, -69.00000000000000000, 36.25000000000000000 ) ) ;
#24274=CARTESIAN_POINT ( 'NONE',  ( -13.82310862920000005, -74.00000000000000000, 36.20061004779999791 ) ) ;
#24275=CARTESIAN_POINT ( 'NONE',  ( -32.81624540183023697, -79.75525706503896117, -22.27658736101337666 ) ) ;
#24276=CYLINDRICAL_SURFACE ( 'NONE', #26930, 0.5000000000000004441 ) ;
#24277=B_SPLINE_SURFACE_WITH_KNOTS ( 'NONE', 4, 5, ( 
 ( #24021, #14566, #25798, #12921, #21837, #1891, #8280, #5954, #12505 ),
 ( #1333, #10176, #23599, #14973, #10728, #19094, #27838, #12786, #23885 ),
 ( #8017, #14837, #16907, #25656, #5686, #21557, #21416, #1474, #10315 ),
 ( #17180, #2034, #11014, #17763, #8850, #20088, #13077, #24315, #26503 ),
 ( #21986, #4645, #26649, #24607, #11330, #6837, #6693, #15701, #10875 ) ),
 .UNSPECIFIED., .F., .F., .F.,
 ( 5, 5 ),
 ( 6, 3, 6 ),
 ( 4.938368304360000033E-16, 6.855861996819999860 ),
 ( 0.000000000000000000, 1.000000000000000000, 2.000000000000000000 ),
 .UNSPECIFIED. ) ;
#24278=ORIENTED_EDGE ( 'NONE', *, *, #16719, .F. ) ;
#24279=DIRECTION ( 'NONE',  ( 0.000000000000000000, 1.000000000000000000, 0.000000000000000000 ) ) ;
#24287=CARTESIAN_POINT ( 'NONE',  ( -22.51794828416004890, -79.95513383975661270, -32.71047865149532896 ) ) ;
#24289=CIRCLE ( 'NONE', #5700, 4.750000000000000000 ) ;
#24295=ORIENTED_EDGE ( 'NONE', *, *, #734, .F. ) ;
#24297=CARTESIAN_POINT ( 'NONE',  ( 46.45339896309999261, -74.00000000000000000, -4.166463576890000020 ) ) ;
#24298=ORIENTED_EDGE ( 'NONE', *, *, #607, .T. ) ;
#24300=CARTESIAN_POINT ( 'NONE',  ( -22.21938216790000098, -80.01919940119999808, -32.54924996240000468 ) ) ;
#24302=B_SPLINE_CURVE_WITH_KNOTS ( 'NONE', 3,
 ( #14528, #6056, #10280, #23840, #3471, #23986, #7979, #19188, #15077, #17436, #12882, #14671, #1576, #17287, #12336, #10416, #14936, #12608, #4020, #21798, #10138, #23565, #1854, #10695, #21244, #8245, #3883, #28209, #16869, #1295, #21660 ),
 .UNSPECIFIED., .F., .F.,
 ( 4, 2, 2, 1, 1, 2, 2, 2, 1, 1, 2, 2, 2, 1, 1, 1, 2, 2, 4 ),
 ( 0.000000000000000000, 0.1250000000000730527, 0.1875000000001095790, 0.2187500000001328382, 0.2343750000001279810, 0.2421875000001261768, 0.2500000000001244005, 0.3750000000000689448, 0.4375000000000421330, 0.4687500000000286993, 0.4843750000000281442, 0.5000000000000276446, 0.6249999999998725464, 0.6874999999997949418, 0.7187499999997526423, 0.7343749999997410960, 0.7421874999997390976, 0.7499999999997370992, 1.000000000000000000 ),
 .UNSPECIFIED. ) ;
#24305=CARTESIAN_POINT ( 'NONE',  ( 8.479934984299998035, -37.33301741529999873, -21.77931235099999796 ) ) ;
#24306=EDGE_CURVE ( 'NONE', #26673, #9115, #19705, .T. ) ;
#24308=AXIS2_PLACEMENT_3D ( 'NONE', #17712, #21936, #28624 ) ;
#24310=VERTEX_POINT ( 'NONE', #14558 ) ;
#24312=CARTESIAN_POINT ( 'NONE',  ( 36.36428601960000151, -73.99923028089999377, -13.97901162650000018 ) ) ;
#24315=CARTESIAN_POINT ( 'NONE',  ( -0.8467854781579999823, -56.26681992150000156, -23.30550165100000015 ) ) ;
#24317=CARTESIAN_POINT ( 'NONE',  ( 11.16657025251494417, -72.37633449930413576, -26.91772825060574803 ) ) ;
#24320=FACE_OUTER_BOUND ( 'NONE', #2940, .T. ) ;
#24321=CARTESIAN_POINT ( 'NONE',  ( 20.31287103041500330, -73.22909343996219889, -31.37144790015285167 ) ) ;
#24323=CARTESIAN_POINT ( 'NONE',  ( 7.619628858569999608, -36.43422328860000192, -21.46039065680000135 ) ) ;
#24327=B_SPLINE_CURVE_WITH_KNOTS ( 'NONE', 3,
 ( #13228, #26219, #6387, #4205, #8281, #22139, #19504, #28668, #10583, #23887, #10878, #19643, #21559, #10452, #26068, #28388, #1614, #6098, #19931, #28535, #8570, #24317, #13080, #2178, #21988, #2037, #17181, #24023, #17474, #26652, #5, #17327, #8852 ),
 .UNSPECIFIED., .F., .F.,
 ( 4, 2, 2, 1, 2, 2, 2, 2, 1, 2, 2, 2, 2, 1, 1, 1, 2, 2, 4 ),
 ( 0.000000000000000000, 0.1250000000000635048, 0.1875000000000947020, 0.2187500000001103007, 0.2343750000001184330, 0.2500000000001265654, 0.3750000000001944556, 0.4375000000002257083, 0.4687500000002383094, 0.4843750000002446376, 0.5000000000002509104, 0.6250000000003361755, 0.6875000000003781420, 0.7187500000003974598, 0.7343750000004078959, 0.7421875000004114487, 0.7460937500004124479, 0.7500000000004134471, 1.000000000000000000 ),
 .UNSPECIFIED. ) ;
#24329=VECTOR ( 'NONE', #16510, 1000.000000000000000 ) ;
#24330=PLANE ( 'NONE',  #25146 ) ;
#24331=ORIENTED_EDGE ( 'NONE', *, *, #5451, .F. ) ;
#24334=CARTESIAN_POINT ( 'NONE',  ( -13.56438818361382914, -18.97801334097803760, 20.36277990756491718 ) ) ;
#24335=CARTESIAN_POINT ( 'NONE',  ( 9.364228581315421351, -35.99000303267523293, -19.78658063234450992 ) ) ;
#24337=CARTESIAN_POINT ( 'NONE',  ( 8.855030637886567746, -36.23917065938484683, -21.13310776212970055 ) ) ;
#24338=ADVANCED_FACE ( 'NONE', ( #12362 ), #15493, .T. ) ;
#24345=CARTESIAN_POINT ( 'NONE',  ( -10.95392404250000062, -19.15751145089999952, -19.17041938750000085 ) ) ;
#24348=ADVANCED_FACE ( 'NONE', ( #14289 ), #12089, .F. ) ;
#24349=CARTESIAN_POINT ( 'NONE',  ( 20.78260698670000295, -56.78056608349999834, 38.04230691420000454 ) ) ;
#24351=CARTESIAN_POINT ( 'NONE',  ( 25.15895431540000260, -70.69114014129999646, 11.62372445859999814 ) ) ;
#24352=CARTESIAN_POINT ( 'NONE',  ( -32.72159597179999935, -74.32000120609998817, -21.62349002899999917 ) ) ;
#24353=ORIENTED_EDGE ( 'NONE', *, *, #10084, .F. ) ;
#24354=AXIS2_PLACEMENT_3D ( 'NONE', #7465, #2943, #11806 ) ;
#24357=DIRECTION ( 'NONE',  ( 0.000000000000000000, -1.000000000000000000, 0.000000000000000000 ) ) ;
#24358=VERTEX_POINT ( 'NONE', #777 ) ;
#24359=CARTESIAN_POINT ( 'NONE',  ( 27.79603073779999889, -69.50480368919998853, 2.066568264030000268 ) ) ;
#24361=CARTESIAN_POINT ( 'NONE',  ( 24.20036131582700634, -74.16719602402496037, -30.74030054472169837 ) ) ;
#24363=CARTESIAN_POINT ( 'NONE',  ( 24.55403954519999843, -64.36570418790000758, -9.970356804210000590 ) ) ;
#24364=ORIENTED_EDGE ( 'NONE', *, *, #12887, .T. ) ;
#24366=AXIS2_PLACEMENT_3D ( 'NONE', #25128, #22505, #11696 ) ;
#24370=CARTESIAN_POINT ( 'NONE',  ( 7.479537002301369419, -74.09468416706585003, 39.31219897218797144 ) ) ;
#24373=EDGE_CURVE ( 'NONE', #9035, #6367, #13187, .T. ) ;
#24375=VERTEX_POINT ( 'NONE', #14150 ) ;
#24376=DIRECTION ( 'NONE',  ( 1.000000000000000000, 0.000000000000000000, 0.000000000000000000 ) ) ;
#24378=DIRECTION ( 'NONE',  ( -1.000000000000000000, 0.000000000000000000, 0.000000000000000000 ) ) ;
#24380=ORIENTED_EDGE ( 'NONE', *, *, #607, .F. ) ;
#24381=EDGE_CURVE ( 'NONE', #28257, #7849, #25320, .T. ) ;
#24383=AXIS2_PLACEMENT_3D ( 'NONE', #20910, #22659, #27174 ) ;
#24384=DIRECTION ( 'NONE',  ( 0.7520801565632392327, -0.3326668106484357845, 0.5689536283360986380 ) ) ;
#24388=ORIENTED_EDGE ( 'NONE', *, *, #2849, .F. ) ;
#24390=CARTESIAN_POINT ( 'NONE',  ( 28.24050769817818107, -69.80859171892026893, 2.425102034864300649 ) ) ;
#24391=CARTESIAN_POINT ( 'NONE',  ( -15.95377854864229050, -19.50000000000000000, 21.99697738415282799 ) ) ;
#24393=B_SPLINE_CURVE_WITH_KNOTS ( 'NONE', 5,
 ( #15879, #22011, #8873, #15724, #13250, #28686 ),
 .UNSPECIFIED., .F., .F.,
 ( 6, 6 ),
 ( 0.000000000000000000, 1.000000000000000000 ),
 .UNSPECIFIED. ) ;
#24396=CARTESIAN_POINT ( 'NONE',  ( -12.07617952120000027, -66.61054971539999769, -23.44199634219999950 ) ) ;
#24397=AXIS2_PLACEMENT_3D ( 'NONE', #18429, #22957, #13901 ) ;
#24403=CARTESIAN_POINT ( 'NONE',  ( -14.06310087329999803, -61.59908875819999707, 21.57936076700000072 ) ) ;
#24405=CARTESIAN_POINT ( 'NONE',  ( -13.51150976399999948, -58.88293941810000121, 20.78295126999999809 ) ) ;
#24406=DIRECTION ( 'NONE',  ( 0.3687499999999814260, 0.000000000000000000, -0.9295286103719527793 ) ) ;
#24409=CARTESIAN_POINT ( 'NONE',  ( -19.96385611919999903, -52.58489974430000302, 14.40794232450000045 ) ) ;
#24411=ADVANCED_FACE ( 'NONE', ( #19492 ), #12264, .T. ) ;
#24412=EDGE_LOOP ( 'NONE', ( #19732, #26827, #20586, #3638 ) ) ;
#24415=ORIENTED_EDGE ( 'NONE', *, *, #12515, .F. ) ;
#24416=EDGE_CURVE ( 'NONE', #7866, #10585, #25073, .T. ) ;
#24420=CARTESIAN_POINT ( 'NONE',  ( 19.76472763569999813, -19.46501104069999855, 9.931837840570000964 ) ) ;
#24421=FACE_OUTER_BOUND ( 'NONE', #1276, .T. ) ;
#24424=CARTESIAN_POINT ( 'NONE',  ( 11.38850808709999995, -70.45799658879998617, -26.88027528670000166 ) ) ;
#24427=TOROIDAL_SURFACE ( 'NONE', #22102, 7.750000000000000000, 0.5000000000000000000 ) ;
#24429=CARTESIAN_POINT ( 'NONE',  ( -9.597487326430000465, -80.50000000000000000, 38.57396449699999863 ) ) ;
#24431=CARTESIAN_POINT ( 'NONE',  ( 21.63872345726285928, -19.48618186048361522, 9.527059235570996876 ) ) ;
#24441=ADVANCED_FACE ( 'NONE', ( #19220 ), #23451, .F. ) ;
#24442=EDGE_CURVE ( 'NONE', #12207, #8283, #22649, .T. ) ;
#24443=LINE ( 'NONE', #18032, #5194 ) ;
#24445=VERTEX_POINT ( 'NONE', #25789 ) ;
#24448=CARTESIAN_POINT ( 'NONE',  ( 46.63086251900000434, -74.05159139319999895, -3.730496185299999823 ) ) ;
#24451=CARTESIAN_POINT ( 'NONE',  ( -22.29173994399999970, -79.81702446639999948, -32.80950025890000177 ) ) ;
#24452=CARTESIAN_POINT ( 'NONE',  ( 9.561259125210000320, -36.00000000000000000, -20.11250876450000291 ) ) ;
#24454=CARTESIAN_POINT ( 'NONE',  ( -0.5590517731190000061, -18.50000000000000000, -21.02688049580000040 ) ) ;
#24458=CARTESIAN_POINT ( 'NONE',  ( -21.65925653600000444, -74.22385006870000268, -32.64405417670000276 ) ) ;
#24460=AXIS2_PLACEMENT_3D ( 'NONE', #26527, #6568, #25377 ) ;
#24462=CARTESIAN_POINT ( 'NONE',  ( -7.344253762436438571, -73.99970746456109794, 39.37955618711904293 ) ) ;
#24463=CARTESIAN_POINT ( 'NONE',  ( 7.250043397162129644, -74.39270540171456503, -40.35498444578576738 ) ) ;
#24464=ORIENTED_EDGE ( 'NONE', *, *, #1716, .T. ) ;
#24467=CARTESIAN_POINT ( 'NONE',  ( 9.564509902230000193, -57.40875702419999982, -23.52622212079999997 ) ) ;
#24469=DIRECTION ( 'NONE',  ( 0.09756097560976997873, 0.000000000000000000, -0.9952295494196653491 ) ) ;
#24470=DIRECTION ( 'NONE',  ( 0.000000000000000000, 1.000000000000000000, 0.000000000000000000 ) ) ;
#24471=AXIS2_PLACEMENT_3D ( 'NONE', #18897, #27779, #18464 ) ;
#24472=EDGE_CURVE ( 'NONE', #5884, #15706, #6205, .T. ) ;
#24474=ADVANCED_FACE ( 'NONE', ( #26059 ), #23856, .F. ) ;
#24476=ORIENTED_EDGE ( 'NONE', *, *, #12736, .T. ) ;
#24477=B_SPLINE_CURVE_WITH_KNOTS ( 'NONE', 3,
 ( #16881, #21255, #5798, #12210 ),
 .UNSPECIFIED., .F., .F.,
 ( 4, 4 ),
 ( 1.645588054440000114, 2.780179228649999779 ),
 .UNSPECIFIED. ) ;
#24478=FACE_OUTER_BOUND ( 'NONE', #14897, .T. ) ;
#24481=CARTESIAN_POINT ( 'NONE',  ( -11.74919335509999918, -57.47571039350000177, 20.26880008290000035 ) ) ;
#24482=FACE_OUTER_BOUND ( 'NONE', #18183, .T. ) ;
#24483=VERTEX_POINT ( 'NONE', #22572 ) ;
#24484=CARTESIAN_POINT ( 'NONE',  ( -6.903469049429999949, -74.00000000000000000, 46.75000000000000000 ) ) ;
#24486=CARTESIAN_POINT ( 'NONE',  ( 22.55816085667000692, -34.67040743918621359, -0.5428485797609520214 ) ) ;
#24487=CARTESIAN_POINT ( 'NONE',  ( 9.510880446319999848, -36.06003250090000023, -20.82958080039999871 ) ) ;
#24488=DIRECTION ( 'NONE',  ( 0.000000000000000000, 1.000000000000000000, 0.000000000000000000 ) ) ;
#24489=CARTESIAN_POINT ( 'NONE',  ( -11.16934527530000132, -19.15747282889999781, -18.98222458509999910 ) ) ;
#24490=CARTESIAN_POINT ( 'NONE',  ( 22.66044434279999820, -66.11532834579999474, 11.96275783630000156 ) ) ;
#24493=CARTESIAN_POINT ( 'NONE',  ( -20.38120117614986171, -61.35278060542812284, 12.44166777117195544 ) ) ;
#24494=DIRECTION ( 'NONE',  ( 0.000000000000000000, 1.000000000000000000, 0.000000000000000000 ) ) ;
#24495=CARTESIAN_POINT ( 'NONE',  ( -32.08195032130000612, -74.00665451570000641, -21.91676683800000092 ) ) ;
#24499=CARTESIAN_POINT ( 'NONE',  ( -14.48711453910000024, -79.93770852559998730, 37.01826959139999929 ) ) ;
#24501=CARTESIAN_POINT ( 'NONE',  ( 28.08445624330000001, -69.30631424429999754, 2.280942866869999808 ) ) ;
#24503=CARTESIAN_POINT ( 'NONE',  ( 27.75394116159999669, -74.50000000000000000, -27.75394116159999669 ) ) ;
#24504=CARTESIAN_POINT ( 'NONE',  ( -19.65424240801501199, -57.45864753664992008, 13.63538986705772160 ) ) ;
#24506=CARTESIAN_POINT ( 'NONE',  ( 23.33235093769999935, -63.43007729560000740, -8.903997769090000958 ) ) ;
#24510=EDGE_CURVE ( 'NONE', #723, #16270, #144, .T. ) ;
#24513=B_SPLINE_CURVE_WITH_KNOTS ( 'NONE', 5,
 ( #14782, #23826, #3868, #12865, #1695, #10531 ),
 .UNSPECIFIED., .F., .F.,
 ( 6, 6 ),
 ( 0.000000000000000000, 1.000000000000000000 ),
 .UNSPECIFIED. ) ;
#24516=CARTESIAN_POINT ( 'NONE',  ( -47.25000000000000000, -82.25000000000000000, -8.214972755869998945E-15 ) ) ;
#24517=B_SPLINE_SURFACE_WITH_KNOTS ( 'NONE', 5, 5, ( 
 ( #24729, #413, #4764, #564, #4904, #9409 ),
 ( #9263, #22836, #16110, #711, #13639, #20493 ),
 ( #2731, #7393, #18462, #11887, #20653, #22983 ),
 ( #20940, #2881, #13784, #22686, #13935, #18317 ),
 ( #9563, #11738, #16257, #25167, #18162, #20344 ),
 ( #25011, #2591, #27061, #853, #11585, #25317 ) ),
 .UNSPECIFIED., .F., .F., .F.,
 ( 6, 6 ),
 ( 6, 6 ),
 ( 16.61710410409999739, 20.91501685549999934 ),
 ( 0.000000000000000000, 2.000000000000000000 ),
 .UNSPECIFIED. ) ;
#24518=CARTESIAN_POINT ( 'NONE',  ( 22.86947465604172436, -19.47453829777655443, 1.128719766882153364 ) ) ;
#24521=CARTESIAN_POINT ( 'NONE',  ( 26.81678742717032193, -72.67627779146050671, -10.37109992809414827 ) ) ;
#24522=CARTESIAN_POINT ( 'NONE',  ( 9.175366638180001644, -35.90614572970000040, -19.93301557890000097 ) ) ;
#24526=CARTESIAN_POINT ( 'NONE',  ( 21.34453858160000195, -18.50000000000000000, -0.07199018194310001506 ) ) ;
#24534=EDGE_CURVE ( 'NONE', #8919, #13409, #28075, .T. ) ;
#24535=CARTESIAN_POINT ( 'NONE',  ( 7.215414233289999757, -82.25000000000000000, -40.70731707320000226 ) ) ;
#24545=COLOUR_RGB ( '', 0.40784314, 0.44705882, 0.49803922) ;
#24546=EDGE_LOOP ( 'NONE', ( #1491, #23281, #27742 ) ) ;
#24547=CARTESIAN_POINT ( 'NONE',  ( -12.69597419230000135, -65.01950817790000769, 21.68734838749999838 ) ) ;
#24548=CARTESIAN_POINT ( 'NONE',  ( -13.88246128279999958, -63.14781701039999717, 21.47252710969999967 ) ) ;
#24551=CARTESIAN_POINT ( 'NONE',  ( -20.25037018340000117, -54.99674360790000094, 14.65440538810000071 ) ) ;
#24552=CARTESIAN_POINT ( 'NONE',  ( -11.13193851743714191, -32.10667435364714350, -22.10121990970652561 ) ) ;
#24553=ORIENTED_EDGE ( 'NONE', *, *, #21490, .T. ) ;
#24555=CARTESIAN_POINT ( 'NONE',  ( 30.16735348728591504, -74.23014832817669628, -24.98698552860614797 ) ) ;
#24556=TOROIDAL_SURFACE ( 'NONE', #10122, 7.750000000000000000, 0.5000000000000000000 ) ;
#24557=CARTESIAN_POINT ( 'NONE',  ( 7.332363419890000067, -74.23956954040001222, -39.85902549529999561 ) ) ;
#24558=ORIENTED_EDGE ( 'NONE', *, *, #27939, .F. ) ;
#24562=CARTESIAN_POINT ( 'NONE',  ( 19.94281239099999681, -26.09793778660000285, 10.08502759879999999 ) ) ;
#24566=CARTESIAN_POINT ( 'NONE',  ( 20.22035593609999893, -19.15979404320000157, 9.591164680889999516 ) ) ;
#24567=CARTESIAN_POINT ( 'NONE',  ( 8.386163660559999400, -68.18701866809999501, -25.21061429379999907 ) ) ;
#24569=ORIENTED_EDGE ( 'NONE', *, *, #15788, .T. ) ;
#24571=CARTESIAN_POINT ( 'NONE',  ( -14.67079199201519657, -67.87586507525224988, 22.52608771271433596 ) ) ;
#24575=CARTESIAN_POINT ( 'NONE',  ( -39.96405813100000159, -74.08838618849999591, -7.268564243729999319 ) ) ;
#24577=EDGE_CURVE ( 'NONE', #3729, #10287, #2837, .T. ) ;
#24578=B_SPLINE_CURVE_WITH_KNOTS ( 'NONE', 5,
 ( #22302, #22159, #588, #8727, #25036, #22863, #9432, #5070, #735 ),
 .UNSPECIFIED., .F., .F.,
 ( 6, 3, 6 ),
 ( 0.000000000000000000, 0.5000000000000000000, 1.000000000000000000 ),
 .UNSPECIFIED. ) ;
#24581=VERTEX_POINT ( 'NONE', #5077 ) ;
#24584=CARTESIAN_POINT ( 'NONE',  ( 0.000000000000000000, -57.47855601759999900, 0.000000000000000000 ) ) ;
#24587=ORIENTED_EDGE ( 'NONE', *, *, #7215, .F. ) ;
#24589=AXIS2_PLACEMENT_3D ( 'NONE', #6453, #13149, #26141 ) ;
#24593=CARTESIAN_POINT ( 'NONE',  ( -13.16183723299999997, -70.12921532840000793, -24.09258145020000086 ) ) ;
#24597=CARTESIAN_POINT ( 'NONE',  ( -22.19845100579999908, -79.83484740680000868, -32.70622245319999877 ) ) ;
#24598=ADVANCED_FACE ( 'NONE', ( #20232 ), #7273, .F. ) ;
#24599=DIRECTION ( 'NONE',  ( 0.7678754814159398645, 0.000000000000000000, -0.6405991297529514128 ) ) ;
#24601=LINE ( 'NONE', #28660, #19404 ) ;
#24602=ORIENTED_EDGE ( 'NONE', *, *, #28003, .T. ) ;
#24604=CARTESIAN_POINT ( 'NONE',  ( -2.644509777640000170, -62.27955658970000030, -25.79865804869999835 ) ) ;
#24605=CARTESIAN_POINT ( 'NONE',  ( -39.64142120219999299, -73.82497517469998627, 7.260602597430000138 ) ) ;
#24606=CARTESIAN_POINT ( 'NONE',  ( -21.92609131280000057, -74.01492597349999869, -32.13963591329999758 ) ) ;
#24607=CARTESIAN_POINT ( 'NONE',  ( -2.353367408570000041, -57.44036991819999827, -24.34032937810000163 ) ) ;
#24609=CARTESIAN_POINT ( 'NONE',  ( 21.02965361369999897, -18.50000000000000000, -0.4426258060200000122 ) ) ;
#24611=CARTESIAN_POINT ( 'NONE',  ( -18.04642050529999864, -18.61786835250000038, 12.22684699669999908 ) ) ;
#24612=VERTEX_POINT ( 'NONE', #13367 ) ;
#24613=CIRCLE ( 'NONE', #6002, 10.49999999999999822 ) ;
#24614=AXIS2_PLACEMENT_3D ( 'NONE', #8969, #6955, #17875 ) ;
#24621=CARTESIAN_POINT ( 'NONE',  ( 40.65853658540000026, -84.00000000000000000, -6.717799458580000049 ) ) ;
#24622=CARTESIAN_POINT ( 'NONE',  ( 45.99664575370000108, -80.06168502749999050, -4.396813293179999249 ) ) ;
#24623=EDGE_CURVE ( 'NONE', #6901, #19131, #17849, .T. ) ;
#24624=B_SPLINE_CURVE_WITH_KNOTS ( 'NONE', 3,
 ( #24128, #11132, #20198, #15515, #26912, #22098, #24726, #20051, #18013, #24275, #271, #6349 ),
 .UNSPECIFIED., .F., .F.,
 ( 4, 2, 2, 2, 2, 4 ),
 ( 0.000000000000000000, 0.2499999999999988898, 0.3749999999999893974, 0.4374999999999802935, 0.4999999999999711897, 1.000000000000000000 ),
 .UNSPECIFIED. ) ;
#24625=DIRECTION ( 'NONE',  ( 0.7071067811865475727, 0.000000000000000000, -0.7071067811865475727 ) ) ;
#24627=CYLINDRICAL_SURFACE ( 'NONE', #7547, 2.999999999999996447 ) ;
#24628=CARTESIAN_POINT ( 'NONE',  ( 24.39713799250000292, -19.50000027030000282, 1.459766484860000046 ) ) ;
#24629=CIRCLE ( 'NONE', #22774, 22.03370205219999889 ) ;
#24630=ORIENTED_EDGE ( 'NONE', *, *, #16236, .T. ) ;
#24631=DIRECTION ( 'NONE',  ( 0.000000000000000000, -1.000000000000000000, 0.000000000000000000 ) ) ;
#24633=DIRECTION ( 'NONE',  ( 0.000000000000000000, 1.000000000000000000, 0.000000000000000000 ) ) ;
#24635=AXIS2_PLACEMENT_3D ( 'NONE', #7470, #1202, #27273 ) ;
#24636=AXIS2_PLACEMENT_3D ( 'NONE', #9257, #19889, #20046 ) ;
#24637=ADVANCED_FACE ( 'NONE', ( #28077 ), #15725, .T. ) ;
#24638=B_SPLINE_CURVE_WITH_KNOTS ( 'NONE', 5,
 ( #27333, #7803, #7678, #14356, #13920, #25577, #23250, #3294, #9547 ),
 .UNSPECIFIED., .F., .F.,
 ( 6, 3, 6 ),
 ( 0.000000000000000000, 0.3290135944274085733, 1.000000000000000000 ),
 .UNSPECIFIED. ) ;
#24641=DIRECTION ( 'NONE',  ( 1.000000000000000000, 0.000000000000000000, 0.000000000000000000 ) ) ;
#24643=CARTESIAN_POINT ( 'NONE',  ( -10.66538705860000036, -19.49268907760000147, -21.54408461599999924 ) ) ;
#24644=CARTESIAN_POINT ( 'NONE',  ( 21.56055435100278928, -37.66855076750636755, -7.904811894883319923 ) ) ;
#24649=CARTESIAN_POINT ( 'NONE',  ( -32.53182592119999583, -74.14930846740000447, -21.71085396679999846 ) ) ;
#24650=ORIENTED_EDGE ( 'NONE', *, *, #2210, .F. ) ;
#24658=CARTESIAN_POINT ( 'NONE',  ( 22.06429904920000240, -36.00000000000000000, -11.19681729669999903 ) ) ;
#24659=CARTESIAN_POINT ( 'NONE',  ( -10.76183065640000081, -34.65282384500000035, -20.56657588450000063 ) ) ;
#24661=CIRCLE ( 'NONE', #16265, 1.000000000000000888 ) ;
#24663=FACE_OUTER_BOUND ( 'NONE', #21232, .T. ) ;
#24668=CARTESIAN_POINT ( 'NONE',  ( 7.260602597430000138, -73.82497517469998627, 39.64142120219999299 ) ) ;
#24670=CARTESIAN_POINT ( 'NONE',  ( 20.72386479999999764, -35.83655893530000469, -8.803829908180000885 ) ) ;
#24672=CARTESIAN_POINT ( 'NONE',  ( -3.562216332169999777, -80.49999996399999702, 46.31451619710000500 ) ) ;
#24673=CYLINDRICAL_SURFACE ( 'NONE', #23239, 0.5000000000000004441 ) ;
#24674=CARTESIAN_POINT ( 'NONE',  ( 8.236135946259999230, -37.13048524220000246, -21.55877352099999911 ) ) ;
#24675=EDGE_CURVE ( 'NONE', #14159, #13154, #7007, .T. ) ;
#24676=VECTOR ( 'NONE', #22837, 1000.000000000000000 ) ;
#24677=CARTESIAN_POINT ( 'NONE',  ( 45.99664576247111114, -73.93831497102631545, -4.396813278696650507 ) ) ;
#24678=ORIENTED_EDGE ( 'NONE', *, *, #18544, .T. ) ;
#24679=AXIS2_PLACEMENT_3D ( 'NONE', #19112, #5293, #16924 ) ;
#24684=CARTESIAN_POINT ( 'NONE',  ( -2.619606055569999814, -19.50000000000000000, -24.29997775220000023 ) ) ;
#24685=ADVANCED_FACE ( 'NONE', ( #11581 ), #15483, .T. ) ;
#24688=EDGE_CURVE ( 'NONE', #8180, #18987, #11318, .T. ) ;
#24691=CARTESIAN_POINT ( 'NONE',  ( 25.70538116001676343, -61.18778281473014857, 1.399642238291860741 ) ) ;
#24693=CARTESIAN_POINT ( 'NONE',  ( -14.33930122880000013, -18.50000000000000000, 19.87761826330000048 ) ) ;
#24697=AXIS2_PLACEMENT_3D ( 'NONE', #27690, #18798, #16302 ) ;
#24699=ORIENTED_EDGE ( 'NONE', *, *, #7396, .T. ) ;
#24701=CARTESIAN_POINT ( 'NONE',  ( -14.70960788549999876, -64.89138858019998679, 22.30467294780000032 ) ) ;
#24702=CARTESIAN_POINT ( 'NONE',  ( -12.03855289290000030, -63.62219628589998877, 21.32965301300000149 ) ) ;
#24703=DIRECTION ( 'NONE',  ( 0.000000000000000000, -1.000000000000000000, 0.000000000000000000 ) ) ;
#24704=B_SPLINE_CURVE_WITH_KNOTS ( 'NONE', 5,
 ( #23518, #5730, #12409, #1938, #8195, #10361 ),
 .UNSPECIFIED., .F., .F.,
 ( 6, 6 ),
 ( 0.000000000000000000, 1.000000000000000000 ),
 .UNSPECIFIED. ) ;
#24705=CARTESIAN_POINT ( 'NONE',  ( 19.97576656849999921, -72.00000000000000000, -19.97576656849999921 ) ) ;
#24706=CARTESIAN_POINT ( 'NONE',  ( -6.717799458580000049, -84.50000000000000000, 40.65853658540000026 ) ) ;
#24708=ORIENTED_EDGE ( 'NONE', *, *, #11232, .F. ) ;
#24712=ORIENTED_EDGE ( 'NONE', *, *, #20028, .F. ) ;
#24715=EDGE_CURVE ( 'NONE', #6398, #2162, #2511, .T. ) ;
#24718=CARTESIAN_POINT ( 'NONE',  ( 21.88967610470000125, -26.05152176780000062, 9.642051993350001737 ) ) ;
#24721=CARTESIAN_POINT ( 'NONE',  ( -7.248307137522662202, -73.87844996482024840, -39.84323359139859377 ) ) ;
#24722=AXIS2_PLACEMENT_3D ( 'NONE', #17553, #26011, #3866 ) ;
#24723=EDGE_CURVE ( 'NONE', #17228, #17023, #13598, .T. ) ;
#24725=CARTESIAN_POINT ( 'NONE',  ( 21.02834797730000105, -61.82803953129999996, 11.46254203570000030 ) ) ;
#24726=CARTESIAN_POINT ( 'NONE',  ( -32.75213543914213687, -79.89792018864659440, -22.42386398948077186 ) ) ;
#24728=ORIENTED_EDGE ( 'NONE', *, *, #21648, .F. ) ;
#24729=CARTESIAN_POINT ( 'NONE',  ( -12.04650753100000138, -69.29982884310000202, -25.46956806070000212 ) ) ;
#24730=CARTESIAN_POINT ( 'NONE',  ( 46.25000000000000000, -79.00000000000000000, -13.75000000000000000 ) ) ;
#24732=CARTESIAN_POINT ( 'NONE',  ( 20.72577587939499466, -19.47314420526457468, 9.500409951011533849 ) ) ;
#24733=CARTESIAN_POINT ( 'NONE',  ( -39.89376887310000086, -74.19145175629999756, -7.305188533560000863 ) ) ;
#24734=ORIENTED_EDGE ( 'NONE', *, *, #22310, .F. ) ;
#24737=AXIS2_PLACEMENT_3D ( 'NONE', #27893, #3014, #21204 ) ;
#24744=FACE_OUTER_BOUND ( 'NONE', #13844, .T. ) ;
#24745=VERTEX_POINT ( 'NONE', #1780 ) ;
#24746=CARTESIAN_POINT ( 'NONE',  ( -22.49369758140129960, -69.04718673991095557, 14.86230851755990123 ) ) ;
#24748=CARTESIAN_POINT ( 'NONE',  ( 46.63164392270000036, -73.99951332550000416, -3.186587667189999529 ) ) ;
#24751=CARTESIAN_POINT ( 'NONE',  ( -21.91703890630000018, -80.37806415250000214, -32.56305777900000464 ) ) ;
#24755=CARTESIAN_POINT ( 'NONE',  ( -47.25000000000000000, -73.00000000000000000, 3.352534721190000231E-15 ) ) ;
#24756=ORIENTED_EDGE ( 'NONE', *, *, #24577, .T. ) ;
#24757=EDGE_CURVE ( 'NONE', #6342, #5907, #1440, .T. ) ;
#24760=CARTESIAN_POINT ( 'NONE',  ( -38.71641004229999794, -73.65707963269998970, 7.135467526410000261 ) ) ;
#24761=CARTESIAN_POINT ( 'NONE',  ( -21.89190459030000113, -74.01117791779999777, -32.13651045809999829 ) ) ;
#24765=CARTESIAN_POINT ( 'NONE',  ( -7.485783351098411309, -73.99989201511671411, 38.96042338819187023 ) ) ;
#24766=CARTESIAN_POINT ( 'NONE',  ( -18.55525302259999876, -19.15716910929999628, 11.86885460969999784 ) ) ;
#24769=CARTESIAN_POINT ( 'NONE',  ( 10.33697414329999908, -72.00000000000000000, -28.69893982729999848 ) ) ;
#24770=CARTESIAN_POINT ( 'NONE',  ( 7.936588789669999144, -35.30313509529999294, -21.23424077629999829 ) ) ;
#24772=DIRECTION ( 'NONE',  ( 1.000000000000000000, 0.000000000000000000, 0.000000000000000000 ) ) ;
#24773=CARTESIAN_POINT ( 'NONE',  ( 47.25045229320000573, -79.27360113529999808, -0.9350416584460000680 ) ) ;
#24774=B_SPLINE_SURFACE_WITH_KNOTS ( 'NONE', 4, 5, ( 
 ( #5107, #1191, #9613, #7864, #24930, #18374, #13991, #22897, #11797 ),
 ( #20710, #768, #18514, #27407, #28371, #19210, #8264, #28099, #17309 ),
 ( #10715, #12770, #21540, #3767, #12353, #8138, #12487, #4041, #12906 ),
 ( #23724, #21822, #8403, #6229, #24005, #19482, #1872, #26202, #19355 ),
 ( #10159, #19079, #17161, #19630, #12628, #1596, #25782, #1728, #10569 ) ),
 .UNSPECIFIED., .F., .F., .F.,
 ( 5, 5 ),
 ( 6, 3, 6 ),
 ( 8.029182300089999980E-15, 6.855861996789999857 ),
 ( 0.000000000000000000, 1.000000000000000000, 2.000000000000000000 ),
 .UNSPECIFIED. ) ;
#24775=CARTESIAN_POINT ( 'NONE',  ( 25.32712259480000228, -57.40875702469999453, 1.379782074460000230 ) ) ;
#24776=CARTESIAN_POINT ( 'NONE',  ( 8.028473304129999377, -18.50000000000000000, -18.85230009969999898 ) ) ;
#24780=CARTESIAN_POINT ( 'NONE',  ( 47.02585954350560371, -74.18642135858951292, -1.789303680145066355 ) ) ;
#24781=ORIENTED_EDGE ( 'NONE', *, *, #8972, .T. ) ;
#24782=CARTESIAN_POINT ( 'NONE',  ( -11.52020750800000037, -42.27108258110000349, 19.79605168710000029 ) ) ;
#24783=DIRECTION ( 'NONE',  ( 0.000000000000000000, -1.000000000000000000, 0.000000000000000000 ) ) ;
#24784=VERTEX_POINT ( 'NONE', #2360 ) ;
#24785=CIRCLE ( 'NONE', #12636, 7.249999999999999112 ) ;
#24787=ADVANCED_FACE ( 'NONE', ( #28699 ), #17656, .T. ) ;
#24789=FACE_OUTER_BOUND ( 'NONE', #23714, .T. ) ;
#24790=CARTESIAN_POINT ( 'NONE',  ( 8.797620038699999867, -37.04760834070000186, -21.76996719339999942 ) ) ;
#24792=CARTESIAN_POINT ( 'NONE',  ( -10.39471473370000076, -19.47871561450000044, -20.73499808220000062 ) ) ;
#24793=CARTESIAN_POINT ( 'NONE',  ( 22.90783306289999999, -66.63438074019998680, 12.00069599370000084 ) ) ;
#24794=ORIENTED_EDGE ( 'NONE', *, *, #26724, .F. ) ;
#24798=CARTESIAN_POINT ( 'NONE',  ( -32.17258283129999796, -74.02008960720000630, -21.87546129999999778 ) ) ;
#24799=EDGE_LOOP ( 'NONE', ( #1553, #4370, #11071, #10718 ) ) ;
#24800=CARTESIAN_POINT ( 'NONE',  ( 20.17385775081925914, -18.60284042207205601, -7.562753588496645918 ) ) ;
#24802=CARTESIAN_POINT ( 'NONE',  ( -22.33897789299999914, -68.90459131420000460, 16.95310341020000067 ) ) ;
#24803=EDGE_LOOP ( 'NONE', ( #20851, #16338, #10497 ) ) ;
#24804=CARTESIAN_POINT ( 'NONE',  ( 37.17329344845187222, -80.00000002986575964, -13.70472019879660763 ) ) ;
#24805=CIRCLE ( 'NONE', #22967, 0.9999999999999978906 ) ;
#24806=CARTESIAN_POINT ( 'NONE',  ( -19.77751067240000182, -52.59522851920000619, 14.14810317800000128 ) ) ;
#24807=DIRECTION ( 'NONE',  ( -0.9952295494196657932, 0.000000000000000000, -0.09756097560976527416 ) ) ;
#24809=CARTESIAN_POINT ( 'NONE',  ( -14.78607513363078318, -74.25103023226107268, 36.28681140252551529 ) ) ;
#24810=EDGE_CURVE ( 'NONE', #22379, #9997, #22520, .T. ) ;
#24811=DIRECTION ( 'NONE',  ( 0.000000000000000000, 1.000000000000000000, 0.000000000000000000 ) ) ;
#24813=VERTEX_POINT ( 'NONE', #11054 ) ;
#24815=AXIS2_PLACEMENT_3D ( 'NONE', #5168, #14050, #3000 ) ;
#24817=ORIENTED_EDGE ( 'NONE', *, *, #19807, .F. ) ;
#24818=CARTESIAN_POINT ( 'NONE',  ( 7.283536107469999799, -74.14144860030000928, 39.92836808239999868 ) ) ;
#24820=CARTESIAN_POINT ( 'NONE',  ( 23.63066637245063362, -19.48669443993386352, 1.455896856190272537 ) ) ;
#24821=CARTESIAN_POINT ( 'NONE',  ( 26.82037688552241406, -72.68639319731354931, -10.33655577607157561 ) ) ;
#24823=CARTESIAN_POINT ( 'NONE',  ( 9.166432219540000759, -35.89879984470000096, -19.92145671899999826 ) ) ;
#24825=CARTESIAN_POINT ( 'NONE',  ( 8.353998429006537663, -19.47332482891561511, -20.26327805068222432 ) ) ;
#24827=CARTESIAN_POINT ( 'NONE',  ( 23.56413682950000066, -19.48537698630000037, 1.506493335489999863 ) ) ;
#24833=CARTESIAN_POINT ( 'NONE',  ( -32.83566817450000030, -79.25000000000000000, -22.22906645670000003 ) ) ;
#24834=AXIS2_PLACEMENT_3D ( 'NONE', #4934, #1650, #10486 ) ;
#24835=CARTESIAN_POINT ( 'NONE',  ( 25.93686798816709427, -62.33603094518826992, 1.426352254284204202 ) ) ;
#24837=DIRECTION ( 'NONE',  ( 0.000000000000000000, 1.000000000000000000, 0.000000000000000000 ) ) ;
#24840=CARTESIAN_POINT ( 'NONE',  ( 36.61132492839999486, -74.71742460369999606, -14.71192759290000041 ) ) ;
#24841=B_SPLINE_CURVE_WITH_KNOTS ( 'NONE', 3,
 ( #25855, #14758, #9715, #7410 ),
 .UNSPECIFIED., .F., .F.,
 ( 4, 4 ),
 ( -66.18347591719999912, -38.72099908220000231 ),
 .UNSPECIFIED. ) ;
#24843=AXIS2_PLACEMENT_3D ( 'NONE', #17508, #26393, #15008 ) ;
#24844=EDGE_CURVE ( 'NONE', #3611, #898, #19238, .T. ) ;
#24846=CARTESIAN_POINT ( 'NONE',  ( -13.69048216150000030, -61.75768530429999714, 21.15265907719999916 ) ) ;
#24847=DIRECTION ( 'NONE',  ( 0.000000000000000000, 1.000000000000000000, 0.000000000000000000 ) ) ;
#24849=DIRECTION ( 'NONE',  ( 1.000000000000000000, 0.000000000000000000, 0.000000000000000000 ) ) ;
#24850=CARTESIAN_POINT ( 'NONE',  ( 20.59810119160000141, -36.00000000000000000, -9.165580181560001094 ) ) ;
#24851=ADVANCED_FACE ( 'NONE', ( #10769 ), #26538, .T. ) ;
#24856=CARTESIAN_POINT ( 'NONE',  ( 30.51083463210725810, -74.19211354766501643, -24.52263441801099475 ) ) ;
#24858=ORIENTED_EDGE ( 'NONE', *, *, #13684, .F. ) ;
#24860=EDGE_LOOP ( 'NONE', ( #6677, #2886, #26098 ) ) ;
#24865=CARTESIAN_POINT ( 'NONE',  ( -7.241427273170902623, -74.22736093603683116, -40.35276762194584421 ) ) ;
#24867=CARTESIAN_POINT ( 'NONE',  ( -21.51944571800000006, -66.74192463980000412, 15.33029011760000060 ) ) ;
#24870=FACE_OUTER_BOUND ( 'NONE', #12252, .T. ) ;
#24872=CARTESIAN_POINT ( 'NONE',  ( 38.71641004229999794, -73.50000000000000000, -7.135467526410000261 ) ) ;
#24874=CARTESIAN_POINT ( 'NONE',  ( 23.26869159428434131, -63.26419843741122406, -7.439610865658912608 ) ) ;
#24875=ORIENTED_EDGE ( 'NONE', *, *, #10084, .T. ) ;
#24879=EDGE_CURVE ( 'NONE', #8141, #25766, #24208, .T. ) ;
#24880=DIRECTION ( 'NONE',  ( 0.9295286103719511139, 0.000000000000000000, 0.3687499999999862554 ) ) ;
#24881=EDGE_CURVE ( 'NONE', #20540, #10287, #17420, .T. ) ;
#24886=EDGE_LOOP ( 'NONE', ( #17495, #25822, #18805, #28550 ) ) ;
#24887=AXIS2_PLACEMENT_3D ( 'NONE', #27477, #25297, #981 ) ;
#24890=CARTESIAN_POINT ( 'NONE',  ( 23.03829042120000281, -19.50000000000000000, 10.32398954119999956 ) ) ;
#24891=CARTESIAN_POINT ( 'NONE',  ( 47.16762201259999898, -74.53410573390000593, -1.089910948100000221 ) ) ;
#24892=ORIENTED_EDGE ( 'NONE', *, *, #287, .F. ) ;
#24893=CARTESIAN_POINT ( 'NONE',  ( 7.135467304789999687, -73.50000064450000536, -38.71640881029999548 ) ) ;
#24897=B_SPLINE_CURVE_WITH_KNOTS ( 'NONE', 3,
 ( #4099, #12968, #2665, #20732, #24804, #18091 ),
 .UNSPECIFIED., .F., .F.,
 ( 4, 2, 4 ),
 ( 0.000000000000000000, 0.5000000000000000000, 1.000000000000000000 ),
 .UNSPECIFIED. ) ;
#24902=CARTESIAN_POINT ( 'NONE',  ( 36.74383121569999844, -74.66666670279998641, -14.69280906399999864 ) ) ;
#24905=CARTESIAN_POINT ( 'NONE',  ( -21.99985828019999801, -74.00000000000000000, -31.89935321680000158 ) ) ;
#24908=CARTESIAN_POINT ( 'NONE',  ( -7.511960512013370561, -73.99984148058264566, 38.89461421659916596 ) ) ;
#24909=LINE ( 'NONE', #13524, #1065 ) ;
#24910=ORIENTED_EDGE ( 'NONE', *, *, #21169, .F. ) ;
#24913=CARTESIAN_POINT ( 'NONE',  ( 22.62080797870000382, -64.93834956060000252, 11.20705156650000056 ) ) ;
#24914=CARTESIAN_POINT ( 'NONE',  ( 8.489272773159999730, -34.76176403470000054, -20.80005463859999892 ) ) ;
#24916=ADVANCED_FACE ( 'NONE', ( #26108 ), #12820, .F. ) ;
#24917=CARTESIAN_POINT ( 'NONE',  ( -29.16815472389999897, -74.00000000000000000, -29.16815472389999897 ) ) ;
#24919=CARTESIAN_POINT ( 'NONE',  ( 47.25093520489999577, -79.38329488089999586, -0.8867236800390000395 ) ) ;
#24922=CARTESIAN_POINT ( 'NONE',  ( -12.27127883659999874, -64.93834664010000779, -22.06162167850000344 ) ) ;
#24923=CARTESIAN_POINT ( 'NONE',  ( 23.93802380909999883, -64.72767011149998950, -9.438994838039999280 ) ) ;
#24924=DIRECTION ( 'NONE',  ( 0.000000000000000000, 1.000000000000000000, 0.000000000000000000 ) ) ;
#24928=CARTESIAN_POINT ( 'NONE',  ( 40.00000000000000000, -73.00000000000000000, 2.433892081919999696E-15 ) ) ;
#24929=EDGE_LOOP ( 'NONE', ( #18223, #26550, #20107, #10510 ) ) ;
#24930=CARTESIAN_POINT ( 'NONE',  ( 21.50956136780000350, -52.61368720150000655, 10.11639787100000021 ) ) ;
#24931=ORIENTED_EDGE ( 'NONE', *, *, #22043, .F. ) ;
#24937=CARTESIAN_POINT ( 'NONE',  ( -10.33087021410000084, -18.62222165789999906, -21.72933387530000005 ) ) ;
#24938=CARTESIAN_POINT ( 'NONE',  ( 21.62393716137362176, -37.83478482166370327, -8.109578283838366985 ) ) ;
#24945=DIRECTION ( 'NONE',  ( 1.000000000000000000, 0.000000000000000000, 0.000000000000000000 ) ) ;
#24946=CARTESIAN_POINT ( 'NONE',  ( 7.727581852389999284, -65.07443093669999712, -23.93312597839999967 ) ) ;
#24952=CARTESIAN_POINT ( 'NONE',  ( -14.57086084372058998, -74.12888392171852558, 36.26832171247329484 ) ) ;
#24954=CARTESIAN_POINT ( 'NONE',  ( 25.44280605499999837, -65.72122283910000817, -0.3044463870030000296 ) ) ;
#24955=B_SPLINE_CURVE_WITH_KNOTS ( 'NONE', 5,
 ( #6608, #18117, #13142, #220, #7051, #24672 ),
 .UNSPECIFIED., .F., .F.,
 ( 6, 6 ),
 ( 0.000000000000000000, 1.000000000000000000 ),
 .UNSPECIFIED. ) ;
#24956=EDGE_LOOP ( 'NONE', ( #22676, #12237, #751, #5948, #19403, #7462 ) ) ;
#24957=DIRECTION ( 'NONE',  ( 0.000000000000000000, 1.000000000000000000, 0.000000000000000000 ) ) ;
#24958=DIRECTION ( 'NONE',  ( 1.000000000000000000, 0.000000000000000000, 0.000000000000000000 ) ) ;
#24963=CARTESIAN_POINT ( 'NONE',  ( 22.15930751770139295, -19.46518600424841239, 0.2066986137561050429 ) ) ;
#24965=DIRECTION ( 'NONE',  ( -1.000000000000000000, 0.000000000000000000, 0.000000000000000000 ) ) ;
#24966=CARTESIAN_POINT ( 'NONE',  ( 8.694112515909999672, -36.31461050599999396, -21.07880576559999852 ) ) ;
#24971=CARTESIAN_POINT ( 'NONE',  ( 23.40442542150000094, -18.50000000000000000, 2.199655364299999860 ) ) ;
#24973=DIRECTION ( 'NONE',  ( 0.7071067811865475727, 0.000000000000000000, 0.7071067811865475727 ) ) ;
#24975=CARTESIAN_POINT ( 'NONE',  ( -1.468618107569999998, -45.99312545570000310, -23.12288400899999985 ) ) ;
#24977=DIRECTION ( 'NONE',  ( 0.000000000000000000, 1.000000000000000000, 0.000000000000000000 ) ) ;
#24978=CARTESIAN_POINT ( 'NONE',  ( -41.00000000000000000, -84.50000000000000000, 10.20110288159999890 ) ) ;
#24979=CARTESIAN_POINT ( 'NONE',  ( 21.89436955060000045, -49.11506481569999494, -7.274533568899999914 ) ) ;
#24982=VERTEX_POINT ( 'NONE', #9334 ) ;
#24986=DIRECTION ( 'NONE',  ( 0.4794255386042036715, 0.000000000000000000, 0.8775825618903724257 ) ) ;
#24988=CARTESIAN_POINT ( 'NONE',  ( 19.45347853379999847, -35.02802294540000361, -8.988163599090000844 ) ) ;
#24990=EDGE_CURVE ( 'NONE', #26269, #26341, #22072, .T. ) ;
#24991=DIRECTION ( 'NONE',  ( 0.2414462220490755373, 0.000000000000000000, -0.9704142011833033488 ) ) ;
#24992=CARTESIAN_POINT ( 'NONE',  ( 40.00000000000000000, -73.50000000000000000, -9.769962616700000205E-15 ) ) ;
#24996=CARTESIAN_POINT ( 'NONE',  ( 30.67010299991955691, -74.17477598292983032, -24.29988026823843583 ) ) ;
#24999=CARTESIAN_POINT ( 'NONE',  ( -12.89904789370000060, -65.07443093669999712, -21.58991903219999742 ) ) ;
#25001=EDGE_CURVE ( 'NONE', #452, #16695, #26450, .T. ) ;
#25002=CARTESIAN_POINT ( 'NONE',  ( -3.108624468950000298E-16, -74.00000000000000000, -1.554312234480000048E-16 ) ) ;
#25003=CARTESIAN_POINT ( 'NONE',  ( -16.49390888960000368, -79.50000000000000000, 44.28897684009999836 ) ) ;
#25004=CARTESIAN_POINT ( 'NONE',  ( 19.97576656849999921, -38.00000000000000000, -19.97576656849999921 ) ) ;
#25006=CARTESIAN_POINT ( 'NONE',  ( -14.24982662769999919, -74.06193868690000670, 36.58417219249999874 ) ) ;
#25011=CARTESIAN_POINT ( 'NONE',  ( -11.78426840870000092, -72.00000269519999563, -26.58403829429999732 ) ) ;
#25012=LINE ( 'NONE', #9848, #24676 ) ;
#25013=CARTESIAN_POINT ( 'NONE',  ( -9.356041104380000917, -84.50000000000000000, 37.60355029590000697 ) ) ;
#25017=ORIENTED_EDGE ( 'NONE', *, *, #862, .F. ) ;
#25018=AXIS2_PLACEMENT_3D ( 'NONE', #12993, #23663, #6017 ) ;
#25020=ORIENTED_EDGE ( 'NONE', *, *, #7942, .T. ) ;
#25022=CARTESIAN_POINT ( 'NONE',  ( -2.583989732180000498, -57.40875670289999988, -25.23271578160000317 ) ) ;
#25026=ORIENTED_EDGE ( 'NONE', *, *, #3753, .T. ) ;
#25029=CARTESIAN_POINT ( 'NONE',  ( 21.76996726540000182, -37.04760833810000520, -8.797620137550000052 ) ) ;
#25030=CARTESIAN_POINT ( 'NONE',  ( 46.91509368659999524, -74.22322967379999170, -2.558872053950000058 ) ) ;
#25031=ORIENTED_EDGE ( 'NONE', *, *, #18225, .T. ) ;
#25033=CARTESIAN_POINT ( 'NONE',  ( -11.55286930265329559, -62.03412635121320307, 21.09176644221611241 ) ) ;
#25035=CIRCLE ( 'NONE', #3625, 0.9999999999999996669 ) ;
#25036=CARTESIAN_POINT ( 'NONE',  ( 23.02872706138604997, -64.78279487706441842, 10.89319034239515105 ) ) ;
#25038=CARTESIAN_POINT ( 'NONE',  ( -2.037850653060000017, -66.42763100729999337, -25.87181958200000054 ) ) ;
#25039=EDGE_CURVE ( 'NONE', #26675, #14431, #9182, .T. ) ;
#25040=CARTESIAN_POINT ( 'NONE',  ( -16.56294617020000004, -72.37489744399999836, 23.47174545849999916 ) ) ;
#25042=ADVANCED_FACE ( 'NONE', ( #5273 ), #19255, .F. ) ;
#25044=CARTESIAN_POINT ( 'NONE',  ( -2.584575094900000369, -57.80430444439999604, -25.24242493270000054 ) ) ;
#25045=CARTESIAN_POINT ( 'NONE',  ( 25.53682860819999689, -63.14742133130000923, 1.286276417849999909 ) ) ;
#25046=CARTESIAN_POINT ( 'NONE',  ( -21.71458329359999695, -74.41849501830000690, -32.69645379630000548 ) ) ;
#25048=AXIS2_PLACEMENT_3D ( 'NONE', #3380, #18960, #27843 ) ;
#25052=CARTESIAN_POINT ( 'NONE',  ( 36.66944334404606565, -74.23450616714526973, -14.39398667539986576 ) ) ;
#25055=EDGE_CURVE ( 'NONE', #22026, #12661, #3461, .T. ) ;
#25057=CARTESIAN_POINT ( 'NONE',  ( 23.98990767259999757, -64.35840732030000311, 10.71073183010000029 ) ) ;
#25058=CARTESIAN_POINT ( 'NONE',  ( 7.215414233289999757, -77.00000000000000000, 40.70731707320000226 ) ) ;
#25062=CARTESIAN_POINT ( 'NONE',  ( 22.76317971519999972, -52.57401960330000179, 10.17780311019999928 ) ) ;
#25066=CARTESIAN_POINT ( 'NONE',  ( -11.35317482230000152, -18.50000000000000000, 18.33892987359999793 ) ) ;
#25067=CARTESIAN_POINT ( 'NONE',  ( -12.47307779800000027, -62.13475808420000135, -20.48183934720000110 ) ) ;
#25068=CARTESIAN_POINT ( 'NONE',  ( 25.71399229409999876, -69.35813701630000594, -10.31084904409999936 ) ) ;
#25070=ORIENTED_EDGE ( 'NONE', *, *, #23500, .F. ) ;
#25073=B_SPLINE_CURVE_WITH_KNOTS ( 'NONE', 5,
 ( #28380, #16899, #24014, #21548, #28525, #1604 ),
 .UNSPECIFIED., .F., .F.,
 ( 6, 6 ),
 ( 0.000000000000000000, 1.000000000000000000 ),
 .UNSPECIFIED. ) ;
#25075=CARTESIAN_POINT ( 'NONE',  ( -11.68189216550000076, -27.06313277699999986, 19.27199430059999941 ) ) ;
#25076=DIRECTION ( 'NONE',  ( 0.000000000000000000, 1.000000000000000000, 0.000000000000000000 ) ) ;
#25078=CARTESIAN_POINT ( 'NONE',  ( 9.356041104380000917, -84.50000000000000000, 37.60355029590000697 ) ) ;
#25079=CARTESIAN_POINT ( 'NONE',  ( 21.25272724153304438, -34.80518677145862227, -7.596422886174947209 ) ) ;
#25080=CARTESIAN_POINT ( 'NONE',  ( -0.5335602090290000321, -52.63293862049999916, -23.18581005440000098 ) ) ;
#25081=CARTESIAN_POINT ( 'NONE',  ( -10.87809348075558624, -19.46531138871780442, -19.32212505103515099 ) ) ;
#25084=CARTESIAN_POINT ( 'NONE',  ( 46.70429134840502172, -79.89085532618133811, -3.466657557652187194 ) ) ;
#25086=ADVANCED_FACE ( 'NONE', ( #11660 ), #6873, .T. ) ;
#25088=CARTESIAN_POINT ( 'NONE',  ( -32.51122442309999627, -80.25114697639999406, -21.99314580829999954 ) ) ;
#25089=AXIS2_PLACEMENT_3D ( 'NONE', #18850, #18559, #16645 ) ;
#25090=DIRECTION ( 'NONE',  ( 0.000000000000000000, 1.000000000000000000, 0.000000000000000000 ) ) ;
#25091=ORIENTED_EDGE ( 'NONE', *, *, #24688, .T. ) ;
#25092=DIRECTION ( 'NONE',  ( 0.000000000000000000, 1.000000000000000000, 0.000000000000000000 ) ) ;
#25094=CARTESIAN_POINT ( 'NONE',  ( -14.65665288169999947, -79.50000000000000000, 36.94583914790000279 ) ) ;
#25098=CARTESIAN_POINT ( 'NONE',  ( -20.04612630950000352, -45.94038128989999592, 14.54360384760000180 ) ) ;
#25099=CARTESIAN_POINT ( 'NONE',  ( -24.16979293970000242, -74.00000000000000000, -34.06928787630000244 ) ) ;
#25100=DIRECTION ( 'NONE',  ( 5.551115123129999410E-17, 0.000000000000000000, -1.000000000000000000 ) ) ;
#25101=CARTESIAN_POINT ( 'NONE',  ( 23.23323687250000091, -61.84404940159999597, -9.246319667559999900 ) ) ;
#25102=CARTESIAN_POINT ( 'NONE',  ( 25.99978933049999696, -66.93519943790001037, 0.3672536007030000049 ) ) ;
#25103=B_SPLINE_CURVE_WITH_KNOTS ( 'NONE', 3,
 ( #16845, #25735, #5765, #19170 ),
 .UNSPECIFIED., .F., .F.,
 ( 4, 4 ),
 ( 0.000000000000000000, 1.000000000000000000 ),
 .UNSPECIFIED. ) ;
#25104=AXIS2_PLACEMENT_3D ( 'NONE', #20363, #14248, #18773 ) ;
#25105=CARTESIAN_POINT ( 'NONE',  ( 41.00000000000000000, -84.00000000000000000, 10.20110288159999890 ) ) ;
#25108=ORIENTED_EDGE ( 'NONE', *, *, #11452, .T. ) ;
#25111=CARTESIAN_POINT ( 'NONE',  ( 20.64246525220000095, -36.08173683109999530, -8.980509983870000212 ) ) ;
#25114=CARTESIAN_POINT ( 'NONE',  ( 7.255215663259999559, -74.34471143260000758, 40.30304758909999663 ) ) ;
#25119=CARTESIAN_POINT ( 'NONE',  ( 7.960428606499999837, -37.73115151110000198, -21.57372765530000081 ) ) ;
#25121=EDGE_LOOP ( 'NONE', ( #27060, #26840, #26684, #26773 ) ) ;
#25122=EDGE_CURVE ( 'NONE', #5884, #15706, #9017, .T. ) ;
#25124=CARTESIAN_POINT ( 'NONE',  ( -4.439198032609999743E-16, -74.50000000000000000, 47.25000000000000000 ) ) ;
#25128=CARTESIAN_POINT ( 'NONE',  ( 0.000000000000000000, -18.50000000000000000, 0.000000000000000000 ) ) ;
#25130=CARTESIAN_POINT ( 'NONE',  ( -1.489708121969999910, -39.36011816919999973, -22.89876977989999673 ) ) ;
#25135=DIRECTION ( 'NONE',  ( 0.9295286103719527793, 0.000000000000000000, 0.3687499999999814260 ) ) ;
#25136=CARTESIAN_POINT ( 'NONE',  ( 22.13628143409999893, -57.47600051900000295, -7.675802715190000569 ) ) ;
#25138=CARTESIAN_POINT ( 'NONE',  ( 36.74383121569999844, -74.66666669110000498, -14.69280905019999928 ) ) ;
#25139=EDGE_LOOP ( 'NONE', ( #757, #13338, #2423, #26974 ) ) ;
#25142=CARTESIAN_POINT ( 'NONE',  ( -12.91995238960000059, -67.00951448479999328, 22.59957177110000259 ) ) ;
#25143=CARTESIAN_POINT ( 'NONE',  ( 7.289738943409999727, -36.07481395120000656, -21.45633483510000161 ) ) ;
#25144=CARTESIAN_POINT ( 'NONE',  ( 7.248307137522641774, -73.87844996482074578, 39.84323359139695242 ) ) ;
#25146=AXIS2_PLACEMENT_3D ( 'NONE', #26666, #15871, #6707 ) ;
#25147=CARTESIAN_POINT ( 'NONE',  ( 20.21912291310000143, -36.00000000000000000, -9.726844800120000301 ) ) ;
#25148=DIRECTION ( 'NONE',  ( -0.9295286103719533344, 0.000000000000000000, -0.3687499999999802047 ) ) ;
#25151=CARTESIAN_POINT ( 'NONE',  ( -11.29758003760461449, -43.98373191161520879, -22.34159391827311225 ) ) ;
#25157=ADVANCED_FACE ( 'NONE', ( #10042 ), #17348, .T. ) ;
#25160=B_SPLINE_CURVE_WITH_KNOTS ( 'NONE', 3,
 ( #23303, #11790, #9747, #13981, #2928, #12215, #761, #7450, #23170, #25220, #18935, #12074, #20984, #27817, #16017, #2778, #26044, #19072, #27954, #26196, #6070, #4033, #23450, #3487, #7994, #16885, #19203, #3621, #23858 ),
 .UNSPECIFIED., .F., .F.,
 ( 4, 2, 1, 1, 2, 2, 2, 2, 1, 2, 2, 2, 2, 2, 2, 4 ),
 ( 0.000000000000000000, 0.1250000000000235922, 0.1875000000000369982, 0.2187500000000420219, 0.2343750000000474065, 0.2500000000000527911, 0.3750000000000170419, 0.4375000000000062728, 0.4687499999999934497, 0.4843749999999881761, 0.4999999999999829026, 0.6249999999999834577, 0.6874999999999762412, 0.7187499999999853451, 0.7499999999999943379, 1.000000000000000000 ),
 .UNSPECIFIED. ) ;
#25161=DIRECTION ( 'NONE',  ( 0.000000000000000000, 0.000000000000000000, -1.000000000000000000 ) ) ;
#25162=CARTESIAN_POINT ( 'NONE',  ( -7.215414233289999757, -74.50000000000000000, -40.70731707320000226 ) ) ;
#25163=CARTESIAN_POINT ( 'NONE',  ( -14.78710411640000011, -74.50000000000000000, 36.35833236359999887 ) ) ;
#25164=CARTESIAN_POINT ( 'NONE',  ( -21.05833095519999887, -65.01950792369999022, 13.71407545739999989 ) ) ;
#25165=CARTESIAN_POINT ( 'NONE',  ( -13.68516050610000079, -43.03747692219999976, 20.93629851420000065 ) ) ;
#25167=CARTESIAN_POINT ( 'NONE',  ( -12.35346744019999932, -72.02645921720001354, -25.58537703819999720 ) ) ;
#25168=CARTESIAN_POINT ( 'NONE',  ( 8.805020426260000477, -34.63244859009999743, -20.36793841340000100 ) ) ;
#25169=FACE_OUTER_BOUND ( 'NONE', #3356, .T. ) ;
#25171=AXIS2_PLACEMENT_3D ( 'NONE', #8634, #15325, #17252 ) ;
#25172=CARTESIAN_POINT ( 'NONE',  ( 7.498734568567309466, -73.99999920929936081, -38.65106240728522380 ) ) ;
#25173=ORIENTED_EDGE ( 'NONE', *, *, #22374, .T. ) ;
#25174=VECTOR ( 'NONE', #17783, 1000.000000000000000 ) ;
#25176=EDGE_LOOP ( 'NONE', ( #11796, #18303, #15972, #9729 ) ) ;
#25179=EDGE_CURVE ( 'NONE', #24085, #5884, #24327, .T. ) ;
#25185=ORIENTED_EDGE ( 'NONE', *, *, #25916, .F. ) ;
#25187=CARTESIAN_POINT ( 'NONE',  ( -2.790536503729999840, -64.24504439390000243, -26.36014981959999659 ) ) ;
#25188=CARTESIAN_POINT ( 'NONE',  ( 47.04659111560000184, -74.36053120809999939, -1.844552627969999969 ) ) ;
#25191=CARTESIAN_POINT ( 'NONE',  ( 7.244686332491783176, -74.17170883796306669, -40.27753662853213967 ) ) ;
#25193=AXIS2_PLACEMENT_3D ( 'NONE', #23824, #28333, #28751 ) ;
#25194=ORIENTED_EDGE ( 'NONE', *, *, #27470, .T. ) ;
#25197=CARTESIAN_POINT ( 'NONE',  ( -2.372222499579999866, -65.21231684830000574, -25.69919413619999915 ) ) ;
#25198=CARTESIAN_POINT ( 'NONE',  ( -15.70782602609999756, -68.38632221809999123, 23.02257119289999920 ) ) ;
#25202=CARTESIAN_POINT ( 'NONE',  ( 26.04683907640000129, -62.95225063429998613, 1.424128180149999867 ) ) ;
#25203=FACE_OUTER_BOUND ( 'NONE', #2647, .T. ) ;
#25205=CARTESIAN_POINT ( 'NONE',  ( -1.068597827310000081, -18.61776472269999871, -21.62742878349999742 ) ) ;
#25209=CARTESIAN_POINT ( 'NONE',  ( 23.15409266789999876, -63.61851004920001174, 10.62027102839999948 ) ) ;
#25210=CARTESIAN_POINT ( 'NONE',  ( 8.964905012660000949, -34.98556513209999963, -19.94240293869999903 ) ) ;
#25213=ORIENTED_EDGE ( 'NONE', *, *, #3727, .T. ) ;
#25219=CARTESIAN_POINT ( 'NONE',  ( -11.65671671230000150, -61.59933877579999972, -22.96881371439999953 ) ) ;
#25220=CARTESIAN_POINT ( 'NONE',  ( 37.04698255873401536, -79.90156983920238076, -14.18878285662181327 ) ) ;
#25221=CARTESIAN_POINT ( 'NONE',  ( 25.45277885500000181, -67.58729785420000269, -10.39245563309999909 ) ) ;
#25224=VERTEX_POINT ( 'NONE', #15405 ) ;
#25225=CARTESIAN_POINT ( 'NONE',  ( 47.00563892014582024, -74.15410710641695857, -1.866436577246293638 ) ) ;
#25226=ORIENTED_EDGE ( 'NONE', *, *, #20063, .F. ) ;
#25227=CARTESIAN_POINT ( 'NONE',  ( -10.61285196099999872, -19.46348300730000247, 19.30929595470000137 ) ) ;
#25229=VERTEX_POINT ( 'NONE', #20239 ) ;
#25232=ORIENTED_EDGE ( 'NONE', *, *, #11674, .T. ) ;
#25233=CARTESIAN_POINT ( 'NONE',  ( 39.18035607830000089, -73.62951539670000045, 7.219507042780000106 ) ) ;
#25234=CARTESIAN_POINT ( 'NONE',  ( -10.47910890883315993, -19.47294349888635523, -20.23264493352919402 ) ) ;
#25235=DIRECTION ( 'NONE',  ( 0.000000000000000000, -1.000000000000000000, 0.000000000000000000 ) ) ;
#25236=CARTESIAN_POINT ( 'NONE',  ( -9.365829542560001997, -18.50000000000000000, -20.82431110010000097 ) ) ;
#25238=CARTESIAN_POINT ( 'NONE',  ( 46.70777991640400728, -79.88906770808442559, -3.456174201335132423 ) ) ;
#25248=ORIENTED_EDGE ( 'NONE', *, *, #11635, .T. ) ;
#25250=CARTESIAN_POINT ( 'NONE',  ( -19.60499002909999788, -45.96202241439999625, 14.06799618039999977 ) ) ;
#25251=FACE_OUTER_BOUND ( 'NONE', #25385, .T. ) ;
#25253=CARTESIAN_POINT ( 'NONE',  ( -14.82555510052299219, -74.28534546674652006, 36.29020547809800235 ) ) ;
#25254=AXIS2_PLACEMENT_3D ( 'NONE', #5749, #20929, #14360 ) ;
#25255=DIRECTION ( 'NONE',  ( 1.000000000000000000, 0.000000000000000000, 0.000000000000000000 ) ) ;
#25256=FACE_OUTER_BOUND ( 'NONE', #7250, .T. ) ;
#25259=ORIENTED_EDGE ( 'NONE', *, *, #17372, .T. ) ;
#25260=CARTESIAN_POINT ( 'NONE',  ( 20.34628061889999984, -52.63293862049999916, 11.13082833170000008 ) ) ;
#25261=CARTESIAN_POINT ( 'NONE',  ( -39.27497438212488845, -73.60295742112906225, -7.213678002770810060 ) ) ;
#25264=DIRECTION ( 'NONE',  ( 1.000000000000000000, 0.000000000000000000, 0.000000000000000000 ) ) ;
#25267=B_SPLINE_SURFACE_WITH_KNOTS ( 'NONE', 5, 5, ( 
 ( #16155, #25062, #15863, #22441, #13687, #5096, #2924, #11787, #2486 ),
 ( #20698, #13326, #26607, #6798, #2136, #13478, #8664, #11287, #6648 ),
 ( #1995, #15660, #21794, #10689, #28632, #20193, #267, #9108, #15356 ),
 ( #15510, #2433, #2281, #1849, #4457, #17572, #11128, #19608, #18009 ),
 ( #26465, #22385, #24718, #26907, #21948, #8810, #24562, #28491, #17722 ),
 ( #19888, #6948, #15808, #17431, #12878, #26767, #24420, #8528, #22230 ) ),
 .UNSPECIFIED., .F., .F., .F.,
 ( 6, 6 ),
 ( 6, 3, 6 ),
 ( 0.000000000000000000, 46.92994236199999847 ),
 ( 0.000000000000000000, 1.000000000000000000, 2.000000000000000000 ),
 .UNSPECIFIED. ) ;
#25270=CARTESIAN_POINT ( 'NONE',  ( -18.36547013180332399, -18.60284036876689839, 11.26451427426198215 ) ) ;
#25271=FACE_OUTER_BOUND ( 'NONE', #18950, .T. ) ;
#25273=VERTEX_POINT ( 'NONE', #11176 ) ;
#25274=CARTESIAN_POINT ( 'NONE',  ( 7.215414233289999757, -82.25000000000000000, -40.70731707320000226 ) ) ;
#25276=CARTESIAN_POINT ( 'NONE',  ( -12.71855576417205924, -19.47933348071434523, 19.41975311732825560 ) ) ;
#25279=CARTESIAN_POINT ( 'NONE',  ( -1.588567434916923649, -19.46686856772270602, -22.26502320241943522 ) ) ;
#25283=CARTESIAN_POINT ( 'NONE',  ( -2.406257486749999952, -39.32886505749999628, -23.82325412870000036 ) ) ;
#25286=DIRECTION ( 'NONE',  ( 0.000000000000000000, -1.000000000000000000, 0.000000000000000000 ) ) ;
#25287=CARTESIAN_POINT ( 'NONE',  ( 21.74683343679999936, -44.92713668010000561, -7.877988450920000219 ) ) ;
#25292=CARTESIAN_POINT ( 'NONE',  ( -32.67527180329999936, -79.50000000000055422, -22.00249031559999935 ) ) ;
#25293=CIRCLE ( 'NONE', #27150, 7.250000000000000000 ) ;
#25294=ADVANCED_FACE ( 'NONE', ( #15704 ), #18493, .T. ) ;
#25297=DIRECTION ( 'NONE',  ( 0.000000000000000000, -1.000000000000000000, 0.000000000000000000 ) ) ;
#25299=AXIS2_PLACEMENT_3D ( 'NONE', #1425, #28205, #14664 ) ;
#25302=CARTESIAN_POINT ( 'NONE',  ( -7.105427357599999217E-15, -84.00000000000000000, -3.552713678799999608E-15 ) ) ;
#25306=CARTESIAN_POINT ( 'NONE',  ( 30.67453910217138002, -74.17429583352173950, -24.29361569179353353 ) ) ;
#25309=DIRECTION ( 'NONE',  ( 0.000000000000000000, 1.000000000000000000, 0.000000000000000000 ) ) ;
#25311=CARTESIAN_POINT ( 'NONE',  ( -7.528851423409999022, -74.04592585209999811, 39.12588484300000147 ) ) ;
#25312=CARTESIAN_POINT ( 'NONE',  ( -12.89904789370000060, -65.07443093669999712, -21.58991903219999742 ) ) ;
#25313=CARTESIAN_POINT ( 'NONE',  ( 26.51571562290000017, -74.19534091600000636, -28.99561388480000090 ) ) ;
#25314=CARTESIAN_POINT ( 'NONE',  ( 10.16048931789999976, -72.75494322130001024, -26.79207077499999912 ) ) ;
#25317=CARTESIAN_POINT ( 'NONE',  ( -12.84661343289999991, -72.82938918050000154, -25.64624284649999808 ) ) ;
#25318=CARTESIAN_POINT ( 'NONE',  ( 8.132924317199998754, -25.50459660499999970, -20.70967061410000198 ) ) ;
#25319=CARTESIAN_POINT ( 'NONE',  ( -1.156001381987856513, -57.47571023478692354, -23.39939165675805910 ) ) ;
#25320=CIRCLE ( 'NONE', #20173, 0.4999999999999982236 ) ;
#25321=DIRECTION ( 'NONE',  ( 0.000000000000000000, -1.000000000000000000, 0.000000000000000000 ) ) ;
#25324=VERTEX_POINT ( 'NONE', #2764 ) ;
#25325=EDGE_CURVE ( 'NONE', #2790, #24185, #19126, .T. ) ;
#25326=TOROIDAL_SURFACE ( 'NONE', #7184, 43.34897771020000334, 20.00000000000000000 ) ;
#25327=CARTESIAN_POINT ( 'NONE',  ( -1.156026911079999886, -57.91337896769999816, -23.41449751500000076 ) ) ;
#25328=AXIS2_PLACEMENT_3D ( 'NONE', #17407, #4572, #22068 ) ;
#25329=DIRECTION ( 'NONE',  ( 0.000000000000000000, -1.000000000000000000, 0.000000000000000000 ) ) ;
#25330=EDGE_CURVE ( 'NONE', #3267, #12297, #10074, .T. ) ;
#25333=FACE_OUTER_BOUND ( 'NONE', #27696, .T. ) ;
#25334=CARTESIAN_POINT ( 'NONE',  ( 20.58262107270000030, -36.00000000000000000, -9.698193473849999080 ) ) ;
#25337=AXIS2_PLACEMENT_3D ( 'NONE', #14710, #17041, #16485 ) ;
#25341=CARTESIAN_POINT ( 'NONE',  ( -1.816673240429999892, -68.12125821070000598, -26.48053705119999890 ) ) ;
#25342=CARTESIAN_POINT ( 'NONE',  ( -15.36964020949999998, -68.58917995980000626, 22.84471883390000002 ) ) ;
#25343=ORIENTED_EDGE ( 'NONE', *, *, #9071, .T. ) ;
#25344=CARTESIAN_POINT ( 'NONE',  ( 36.62466550090000084, -74.65121098390000043, -14.68734464040000098 ) ) ;
#25345=AXIS2_PLACEMENT_3D ( 'NONE', #20310, #28615, #2404 ) ;
#25347=CARTESIAN_POINT ( 'NONE',  ( -20.73247391559999997, -63.62260287809999681, 13.04049290600000077 ) ) ;
#25348=ADVANCED_FACE ( 'NONE', ( #11924 ), #19202, .T. ) ;
#25351=CARTESIAN_POINT ( 'NONE',  ( 7.215414233289999757, -82.25000000000000000, 40.70731707320000226 ) ) ;
#25352=CARTESIAN_POINT ( 'NONE',  ( -3.667491169959999908, -18.50000000000000000, -24.01996181969999711 ) ) ;
#25353=CARTESIAN_POINT ( 'NONE',  ( 36.22844186549999534, -74.00000000000000000, -13.75000000000000000 ) ) ;
#25354=VERTEX_POINT ( 'NONE', #26329 ) ;
#25357=DIRECTION ( 'NONE',  ( 0.000000000000000000, -1.000000000000000000, 0.000000000000000000 ) ) ;
#25359=DIRECTION ( 'NONE',  ( 0.000000000000000000, 1.000000000000000000, 0.000000000000000000 ) ) ;
#25360=VERTEX_POINT ( 'NONE', #3750 ) ;
#25361=AXIS2_PLACEMENT_3D ( 'NONE', #4578, #2698, #22360 ) ;
#25362=EDGE_CURVE ( 'NONE', #1165, #8148, #14916, .T. ) ;
#25363=CIRCLE ( 'NONE', #11366, 0.5000000000000004441 ) ;
#25364=DIRECTION ( 'NONE',  ( 0.000000000000000000, -1.000000000000000000, 0.000000000000000000 ) ) ;
#25365=DIRECTION ( 'NONE',  ( 0.000000000000000000, 1.000000000000000000, 0.000000000000000000 ) ) ;
#25368=DIRECTION ( 'NONE',  ( -0.7071067811865470176, 0.000000000000000000, 0.7071067811865480168 ) ) ;
#25371=TOROIDAL_SURFACE ( 'NONE', #18396, 7.750000000000000000, 0.5000000000000000000 ) ;
#25372=CARTESIAN_POINT ( 'NONE',  ( -13.46142422580000009, -34.61116027599999256, 20.44677669700000422 ) ) ;
#25373=CARTESIAN_POINT ( 'NONE',  ( 28.69894246159999796, -72.00000000000000000, -10.33698060819999931 ) ) ;
#25376=CARTESIAN_POINT ( 'NONE',  ( 40.70731707320000226, -74.50000000000000000, 7.215414233289999757 ) ) ;
#25377=DIRECTION ( 'NONE',  ( 1.000000000000000000, 0.000000000000000000, 0.000000000000000000 ) ) ;
#25381=CARTESIAN_POINT ( 'NONE',  ( -32.63327488449999692, -79.88238632670000072, -22.07483759460000172 ) ) ;
#25384=DIRECTION ( 'NONE',  ( 0.000000000000000000, 1.000000000000000000, 0.000000000000000000 ) ) ;
#25385=EDGE_LOOP ( 'NONE', ( #20482, #18654, #9010, #18943 ) ) ;
#25386=AXIS2_PLACEMENT_3D ( 'NONE', #2818, #11828, #800 ) ;
#25388=CARTESIAN_POINT ( 'NONE',  ( -6.514305738480000052, -74.00000000000000000, 35.51864961870000315 ) ) ;
#25389=EDGE_LOOP ( 'NONE', ( #24295, #13230, #19658, #8815 ) ) ;
#25391=AXIS2_PLACEMENT_3D ( 'NONE', #26810, #4803, #2327 ) ;
#25392=B_SPLINE_CURVE_WITH_KNOTS ( 'NONE', 5,
 ( #14049, #21191, #27878, #5014, #22805, #2843 ),
 .UNSPECIFIED., .F., .F.,
 ( 6, 6 ),
 ( 0.000000000000000000, 1.000000000000000000 ),
 .UNSPECIFIED. ) ;
#25393=CARTESIAN_POINT ( 'NONE',  ( -20.17987348730000008, -39.29539198449999304, 14.62286557340000215 ) ) ;
#25394=DIRECTION ( 'NONE',  ( -9.436895709310000674E-16, 0.000000000000000000, 1.000000000000000000 ) ) ;
#25396=EDGE_CURVE ( 'NONE', #11515, #21778, #10552, .T. ) ;
#25397=CARTESIAN_POINT ( 'NONE',  ( 23.27434332070000167, -58.85141487709999808, -9.477375906779998971 ) ) ;
#25400=FACE_BOUND ( 'NONE', #25443, .T. ) ;
#25401=CARTESIAN_POINT ( 'NONE',  ( -22.22906643760000023, -79.50000000000000000, -32.83566815539999340 ) ) ;
#25402=ORIENTED_EDGE ( 'NONE', *, *, #2484, .T. ) ;
#25403=CARTESIAN_POINT ( 'NONE',  ( 7.215414233289999757, -74.50000000000000000, 40.70731707320000226 ) ) ;
#25413=ORIENTED_EDGE ( 'NONE', *, *, #14294, .T. ) ;
#25414=CARTESIAN_POINT ( 'NONE',  ( 20.35668408949999986, -18.85700241039999980, -8.076030211610000009 ) ) ;
#25415=ADVANCED_FACE ( 'NONE', ( #26184 ), #6215, .F. ) ;
#25416=DIRECTION ( 'NONE',  ( 0.000000000000000000, 0.000000000000000000, -1.000000000000000000 ) ) ;
#25419=EDGE_CURVE ( 'NONE', #27403, #24185, #28152, .T. ) ;
#25421=CARTESIAN_POINT ( 'NONE',  ( 20.33060048340120574, -36.00000012572794361, -9.320855385822547134 ) ) ;
#25422=CARTESIAN_POINT ( 'NONE',  ( 22.19980545599999999, -53.27760474010000280, -8.563702697329999225 ) ) ;
#25423=EDGE_CURVE ( 'NONE', #4890, #24185, #22540, .T. ) ;
#25424=DIRECTION ( 'NONE',  ( 0.000000000000000000, -1.000000000000000000, 0.000000000000000000 ) ) ;
#25426=ORIENTED_EDGE ( 'NONE', *, *, #10950, .F. ) ;
#25431=AXIS2_PLACEMENT_3D ( 'NONE', #16048, #4980, #13867 ) ;
#25432=DIRECTION ( 'NONE',  ( 0.000000000000000000, 1.000000000000000000, 0.000000000000000000 ) ) ;
#25433=CARTESIAN_POINT ( 'NONE',  ( 8.773402987799999053, -35.75421199320000198, -20.69709838450000206 ) ) ;
#25434=CARTESIAN_POINT ( 'NONE',  ( 7.169550435208813965, -73.50000000000002842, 38.90587669203541310 ) ) ;
#25435=CARTESIAN_POINT ( 'NONE',  ( 22.96745989159999723, -18.50000000000000000, 9.091461454319999191 ) ) ;
#25438=EDGE_LOOP ( 'NONE', ( #3970, #11036, #5764, #10435 ) ) ;
#25439=SPHERICAL_SURFACE ( 'NONE', #17096, 2.000000000000000000 ) ;
#25441=ORIENTED_EDGE ( 'NONE', *, *, #12355, .F. ) ;
#25442=CARTESIAN_POINT ( 'NONE',  ( 27.35691629450000306, -72.00000000000000000, -11.81987123310000065 ) ) ;
#25443=EDGE_LOOP ( 'NONE', ( #27538, #3403 ) ) ;
#25445=CARTESIAN_POINT ( 'NONE',  ( -7.253522899010000025, -73.81625264650000418, 39.23046895160000247 ) ) ;
#25447=CARTESIAN_POINT ( 'NONE',  ( -12.09704001540000107, -80.00000000000000000, 47.10905722069999513 ) ) ;
#25448=CARTESIAN_POINT ( 'NONE',  ( -23.16986609970000188, -72.82938648530000592, 16.90925194980000157 ) ) ;
#25449=CARTESIAN_POINT ( 'NONE',  ( 21.84907504069999717, -73.17614430409999215, -31.22910235029999981 ) ) ;
#25453=FACE_OUTER_BOUND ( 'NONE', #6698, .T. ) ;
#25454=CARTESIAN_POINT ( 'NONE',  ( 8.972032747380000117, -25.54957623849999848, -19.59884268089999892 ) ) ;
#25455=FACE_OUTER_BOUND ( 'NONE', #16632, .T. ) ;
#25461=CARTESIAN_POINT ( 'NONE',  ( -1.449479884000000052, -58.34046154589999844, -23.55113706229999693 ) ) ;
#25462=CARTESIAN_POINT ( 'NONE',  ( 40.00000000000000000, -82.25000000000000000, 0.000000000000000000 ) ) ;
#25466=CARTESIAN_POINT ( 'NONE',  ( -0.5335602090290000321, -52.63293862049999916, -23.18581005440000098 ) ) ;
#25467=CARTESIAN_POINT ( 'NONE',  ( -7.215414233289999757, -74.50000000000000000, -40.70731707320000226 ) ) ;
#25468=VERTEX_POINT ( 'NONE', #15671 ) ;
#25469=CARTESIAN_POINT ( 'NONE',  ( 7.398926161578894600, -36.73003209889780152, -21.48136641451177908 ) ) ;
#25470=CARTESIAN_POINT ( 'NONE',  ( -11.31192030519693326, -60.02098066203591031, 20.72433129729396839 ) ) ;
#25471=CARTESIAN_POINT ( 'NONE',  ( -2.892691684889999948, -71.70959084179999365, -28.02986260229999971 ) ) ;
#25472=CARTESIAN_POINT ( 'NONE',  ( -14.72314245780000164, -71.04327856650000683, 23.66650937980000080 ) ) ;
#25474=CARTESIAN_POINT ( 'NONE',  ( 36.57652955130000549, -74.41832496969999511, -14.62770612210000110 ) ) ;
#25476=MECHANICAL_DESIGN_GEOMETRIC_PRESENTATION_REPRESENTATION('',(#19422),#24059);
#25478=CARTESIAN_POINT ( 'NONE',  ( 25.36165982329999835, -58.81334883509999401, 1.380217915539999840 ) ) ;
#25482=CARTESIAN_POINT ( 'NONE',  ( -3.561278452559999863, -18.50000000000000000, -23.17450688339999942 ) ) ;
#25483=CARTESIAN_POINT ( 'NONE',  ( 36.42686065015308827, -74.03769727758323427, -14.02198836895357026 ) ) ;
#25485=ADVANCED_FACE ( 'NONE', ( #2292 ), #20204, .T. ) ;
#25488=FACE_OUTER_BOUND ( 'NONE', #26519, .T. ) ;
#25493=CARTESIAN_POINT ( 'NONE',  ( -0.6772741170208298467, -79.75814015466558260, 47.21855544081748945 ) ) ;
#25495=AXIS2_PLACEMENT_3D ( 'NONE', #27112, #5394, #469 ) ;
#25497=CARTESIAN_POINT ( 'NONE',  ( -27.04683438039999999, -74.50000000000000000, -36.23922253580000330 ) ) ;
#25500=CARTESIAN_POINT ( 'NONE',  ( -12.43025579110000045, -34.65279261700000291, 19.60331251459999891 ) ) ;
#25502=EDGE_LOOP ( 'NONE', ( #7839, #19429, #18610, #19293, #26006 ) ) ;
#25504=CARTESIAN_POINT ( 'NONE',  ( 39.45579440730000442, -74.12477399299999092, 7.440489808619999756 ) ) ;
#25505=DIRECTION ( 'NONE',  ( -0.09756097560976770278, 0.000000000000000000, 0.9952295494196655712 ) ) ;
#25507=CARTESIAN_POINT ( 'NONE',  ( -13.44405788329999929, -68.28990366489999531, 22.97003105929999833 ) ) ;
#25508=ORIENTED_EDGE ( 'NONE', *, *, #15265, .F. ) ;
#25509=CARTESIAN_POINT ( 'NONE',  ( -32.50321504749999946, -80.12422352349999244, -22.09864494740000040 ) ) ;
#25510=EDGE_CURVE ( 'NONE', #6300, #5390, #18780, .T. ) ;
#25513=DIRECTION ( 'NONE',  ( 1.000000000000000000, 0.000000000000000000, 0.000000000000000000 ) ) ;
#25515=B_SPLINE_CURVE_WITH_KNOTS ( 'NONE', 5,
 ( #2047, #13537, #18066, #6706, #2335, #15869, #11189, #13692, #24775 ),
 .UNSPECIFIED., .F., .F.,
 ( 6, 3, 6 ),
 ( 0.000000000000000000, 0.5000000000000000000, 1.000000000000000000 ),
 .UNSPECIFIED. ) ;
#25516=CARTESIAN_POINT ( 'NONE',  ( -2.155284377200000545, -80.29279205369999772, 46.98362450949999669 ) ) ;
#25517=CARTESIAN_POINT ( 'NONE',  ( 22.35420107259999867, -19.50000000000000000, 9.881343484100000296 ) ) ;
#25518=ORIENTED_EDGE ( 'NONE', *, *, #8866, .T. ) ;
#25519=AXIS2_PLACEMENT_3D ( 'NONE', #14351, #14626, #21335 ) ;
#25523=CARTESIAN_POINT ( 'NONE',  ( 31.03653123039999784, -73.81134274429999209, -23.56262533510000168 ) ) ;
#25524=CARTESIAN_POINT ( 'NONE',  ( -14.34881109840844715, -70.26101182088159192, 23.47553979952874670 ) ) ;
#25526=CARTESIAN_POINT ( 'NONE',  ( 26.03240350960000171, -67.01088404440000090, -0.1105166297070000053 ) ) ;
#25527=ORIENTED_EDGE ( 'NONE', *, *, #10785, .T. ) ;
#25529=CARTESIAN_POINT ( 'NONE',  ( -22.65530694619999963, -72.00000000000000000, 18.22957389299999775 ) ) ;
#25530=CARTESIAN_POINT ( 'NONE',  ( 19.86285231560000142, -35.99517856170000130, -9.398749189900000189 ) ) ;
#25531=DIRECTION ( 'NONE',  ( 0.3687499999999814260, 0.000000000000000000, -0.9295286103719527793 ) ) ;
#25536=ORIENTED_EDGE ( 'NONE', *, *, #28273, .T. ) ;
#25537=DIRECTION ( 'NONE',  ( -1.000000000000000000, 0.000000000000000000, -3.154042683594194627E-16 ) ) ;
#25545=EDGE_LOOP ( 'NONE', ( #8418, #27826, #18958, #23392, #16663 ) ) ;
#25546=CARTESIAN_POINT ( 'NONE',  ( -14.01103650240000142, -74.00781516410000904, 36.37014139069999885 ) ) ;
#25547=B_SPLINE_CURVE_WITH_KNOTS ( 'NONE', 3,
 ( #17047, #27988, #19235, #8161, #1749, #19375 ),
 .UNSPECIFIED., .F., .F.,
 ( 4, 2, 4 ),
 ( 0.000000000000000000, 0.5000000000000000000, 1.000000000000000000 ),
 .UNSPECIFIED. ) ;
#25551=FACE_OUTER_BOUND ( 'NONE', #26670, .T. ) ;
#25552=B_SPLINE_CURVE_WITH_KNOTS ( 'NONE', 5,
 ( #12509, #19505, #5828, #21418, #15111, #1477 ),
 .UNSPECIFIED., .F., .F.,
 ( 6, 6 ),
 ( -46.77973719450000090, 0.000000000000000000 ),
 .UNSPECIFIED. ) ;
#25553=VECTOR ( 'NONE', #10354, 1000.000000000000000 ) ;
#25554=CARTESIAN_POINT ( 'NONE',  ( 40.00000000000000000, -74.00000000000000000, 1.960630394010000073E-15 ) ) ;
#25556=CARTESIAN_POINT ( 'NONE',  ( -38.96762186407187301, -74.02518375728683964, -7.561767224770083118 ) ) ;
#25557=CARTESIAN_POINT ( 'NONE',  ( -11.29865404370000093, -27.06785567070000198, -19.22788970119999874 ) ) ;
#25558=EDGE_LOOP ( 'NONE', ( #27664, #7200, #23011, #8553 ) ) ;
#25559=AXIS2_PLACEMENT_3D ( 'NONE', #25447, #26294, #12574 ) ;
#25567=CARTESIAN_POINT ( 'NONE',  ( 7.356932666920000585, -36.56810636680000215, -21.47791282949999925 ) ) ;
#25571=ADVANCED_FACE ( 'NONE', ( #12026 ), #5487, .F. ) ;
#25572=DIRECTION ( 'NONE',  ( 0.000000000000000000, 1.000000000000000000, 0.000000000000000000 ) ) ;
#25573=EDGE_CURVE ( 'NONE', #7860, #13129, #18363, .T. ) ;
#25574=LINE ( 'NONE', #23385, #8415 ) ;
#25575=ORIENTED_EDGE ( 'NONE', *, *, #4032, .T. ) ;
#25577=CARTESIAN_POINT ( 'NONE',  ( -1.800056393709054570, -69.76823740066200230, -27.23143567540053311 ) ) ;
#25578=CARTESIAN_POINT ( 'NONE',  ( -12.69354235982726742, -63.63799308303316593, -20.95011642351082415 ) ) ;
#25579=ORIENTED_EDGE ( 'NONE', *, *, #24810, .F. ) ;
#25581=DIRECTION ( 'NONE',  ( -1.000000000000000000, 0.000000000000000000, 0.000000000000000000 ) ) ;
#25582=EDGE_CURVE ( 'NONE', #19131, #13461, #3038, .T. ) ;
#25584=AXIS2_PLACEMENT_3D ( 'NONE', #7310, #13855, #7169 ) ;
#25586=B_SPLINE_CURVE_WITH_KNOTS ( 'NONE', 3,
 ( #17257, #12722, #8221, #17113, #8356, #26156, #25870, #5895, #12439, #3579, #19307, #6028, #21775, #6325, #15052, #3996, #23818, #21635, #25730, #1826, #16982, #21351, #28189, #28470, #12857, #26303, #4138, #10669, #19582, #5760, #24101, #3861, #16841, #8508 ),
 .UNSPECIFIED., .F., .F.,
 ( 4, 2, 2, 2, 1, 1, 2, 2, 2, 2, 1, 1, 2, 2, 2, 2, 2, 2, 4 ),
 ( 0.000000000000000000, 0.1249999999999426292, 0.1874999999999139300, 0.2187499999998982481, 0.2343749999998903932, 0.2421874999998879785, 0.2460937499998875622, 0.2499999999998871458, 0.3749999999999151234, 0.4374999999999292233, 0.4687499999999348299, 0.4843749999999376610, 0.4921874999999391598, 0.4999999999999406031, 0.6249999999999575895, 0.6874999999999661382, 0.7187499999999695799, 0.7499999999999729106, 1.000000000000000000 ),
 .UNSPECIFIED. ) ;
#25590=CARTESIAN_POINT ( 'NONE',  ( 20.34158267359999783, -73.93832881409998947, -32.34203349919999937 ) ) ;
#25594=CARTESIAN_POINT ( 'NONE',  ( 4.656214649959999954E-15, -79.00000000000000000, 40.00000000000000000 ) ) ;
#25595=DIRECTION ( 'NONE',  ( -0.7071067811865475727, 0.000000000000000000, 0.7071067811865475727 ) ) ;
#25600=TOROIDAL_SURFACE ( 'NONE', #12999, 7.750000000000000000, 0.5000000000000000000 ) ;
#25602=DIRECTION ( 'NONE',  ( -0.09756097560976716154, 0.000000000000000000, -0.9952295494196655712 ) ) ;
#25605=CARTESIAN_POINT ( 'NONE',  ( 20.01429421219999938, -35.44265673480000345, -8.963580811669999093 ) ) ;
#25607=B_SPLINE_CURVE_WITH_KNOTS ( 'NONE', 3,
 ( #19679, #5854, #21874, #28568, #15284, #24206, #13114, #10348, #10912, #22025, #8183, #14735, #17069, #2073, #25831, #25963, #14866, #5987, #13560, #2658, #9331, #4971, #8886, #16037, #28697, #26535, #27132, #9038, #6579, #19967, #11213, #7022 ),
 .UNSPECIFIED., .F., .F.,
 ( 4, 2, 1, 1, 1, 2, 2, 2, 1, 1, 1, 2, 2, 2, 1, 1, 1, 1, 2, 2, 4 ),
 ( 0.000000000000000000, 0.1250000000001095235, 0.1875000000001643408, 0.2187500000001895428, 0.2343750000002022271, 0.2421875000002085554, 0.2500000000002148837, 0.3750000000003662071, 0.4375000000004459211, 0.4687500000004778400, 0.4843750000004859446, 0.4921875000004900524, 0.5000000000004941603, 0.6250000000006031842, 0.6875000000006669110, 0.7187500000007002177, 0.7343750000007220891, 0.7421875000007379652, 0.7460937500007444045, 0.7500000000007508438, 1.000000000000000000 ),
 .UNSPECIFIED. ) ;
#25608=ORIENTED_EDGE ( 'NONE', *, *, #4342, .F. ) ;
#25609=DIRECTION ( 'NONE',  ( 0.000000000000000000, 0.000000000000000000, 1.000000000000000000 ) ) ;
#25612=CARTESIAN_POINT ( 'NONE',  ( 40.65508461000000295, -79.00000000000000000, -13.75000000000000000 ) ) ;
#25613=ADVANCED_FACE ( 'NONE', ( #9566 ), #17887, .T. ) ;
#25616=CARTESIAN_POINT ( 'NONE',  ( -22.09417056399443169, -74.04315698458545114, -32.28351515837096741 ) ) ;
#25618=TOROIDAL_SURFACE ( 'NONE', #15341, 0.5000000000000000000, 0.5000000000000000000 ) ;
#25621=CARTESIAN_POINT ( 'NONE',  ( 23.97433208980000074, -62.13475808409999956, -0.5610825628509999996 ) ) ;
#25622=CARTESIAN_POINT ( 'NONE',  ( -20.78736624049999904, -63.14819481680000735, 14.88907486529999957 ) ) ;
#25624=DIRECTION ( 'NONE',  ( 1.000000000000000000, 0.000000000000000000, 0.000000000000000000 ) ) ;
#25625=CARTESIAN_POINT ( 'NONE',  ( -3.338365958889999874, -18.50000000000000000, -23.63904113259999917 ) ) ;
#25626=CARTESIAN_POINT ( 'NONE',  ( 36.73433531666305640, -74.37420903145732609, -14.53002935066677459 ) ) ;
#25627=ORIENTED_EDGE ( 'NONE', *, *, #1880, .F. ) ;
#25629=CARTESIAN_POINT ( 'NONE',  ( 36.93547111259999838, -80.07278442950000397, -13.78755837009999929 ) ) ;
#25630=CARTESIAN_POINT ( 'NONE',  ( 36.71193690820000199, -74.86352340930001503, -14.74418008200000152 ) ) ;
#25632=EDGE_CURVE ( 'NONE', #25958, #12242, #23029, .T. ) ;
#25635=CARTESIAN_POINT ( 'NONE',  ( -0.8967168713914961398, -79.84002594721414425, 47.19433117586794424 ) ) ;
#25636=CIRCLE ( 'NONE', #10258, 1.999999999999997558 ) ;
#25638=EDGE_CURVE ( 'NONE', #8854, #10427, #20212, .T. ) ;
#25644=VERTEX_POINT ( 'NONE', #3580 ) ;
#25646=EDGE_CURVE ( 'NONE', #5424, #17168, #7210, .T. ) ;
#25650=CARTESIAN_POINT ( 'NONE',  ( 47.04106180647456625, -79.61201027780809625, -2.182424667423416675 ) ) ;
#25652=DIRECTION ( 'NONE',  ( 0.000000000000000000, 1.000000000000000000, 0.000000000000000000 ) ) ;
#25655=DIRECTION ( 'NONE',  ( 0.000000000000000000, -1.000000000000000000, 0.000000000000000000 ) ) ;
#25656=CARTESIAN_POINT ( 'NONE',  ( -2.358001274529999858, -55.01779585689999408, -24.27108329320000024 ) ) ;
#25657=CIRCLE ( 'NONE', #2872, 3.499999999999999556 ) ;
#25658=CARTESIAN_POINT ( 'NONE',  ( -2.679185798610000444E-13, -79.50000000000000000, 47.25000000000000000 ) ) ;
#25659=CARTESIAN_POINT ( 'NONE',  ( -37.60355029590000697, -84.50000000000000000, -9.356041104380000917 ) ) ;
#25660=ORIENTED_EDGE ( 'NONE', *, *, #24061, .T. ) ;
#25663=AXIS2_PLACEMENT_3D ( 'NONE', #23956, #24384, #4424 ) ;
#25667=CARTESIAN_POINT ( 'NONE',  ( -14.15696331435236033, -74.02271853708172955, 36.23139294035578217 ) ) ;
#25668=B_SPLINE_SURFACE_WITH_KNOTS ( 'NONE', 5, 5, ( 
 ( #16535, #27326, #22812, #27627, #9958, #25567 ),
 ( #16088, #20628, #25433, #20776, #14214, #3288 ),
 ( #686, #5601, #5176, #5023, #16231, #25143 ),
 ( #14058, #3007, #3145, #23381, #14622, #3560 ),
 ( #1251, #19417, #19555, #24073, #12415, #23524 ),
 ( #28298, #23799, #5740, #10090, #19007, #8202 ) ),
 .UNSPECIFIED., .F., .F., .F.,
 ( 6, 6 ),
 ( 6, 6 ),
 ( 1.600842967049999954, 3.163651481680000099 ),
 ( 0.000000000000000000, 2.000000000000000000 ),
 .UNSPECIFIED. ) ;
#25671=ADVANCED_FACE ( 'NONE', ( #28190 ), #8256, .T. ) ;
#25674=CARTESIAN_POINT ( 'NONE',  ( 21.15739348700000377, -35.90623960370000134, -8.363368093209999188 ) ) ;
#25675=CARTESIAN_POINT ( 'NONE',  ( 19.92559242949999998, -35.99861502429999405, -9.426072644010000445 ) ) ;
#25678=EDGE_CURVE ( 'NONE', #26457, #6032, #8569, .T. ) ;
#25679=AXIS2_PLACEMENT_3D ( 'NONE', #10584, #15251, #24172 ) ;
#25683=VERTEX_POINT ( 'NONE', #18131 ) ;
#25690=CARTESIAN_POINT ( 'NONE',  ( 26.68243298039999800, -70.99734270939998737, 10.68791969299999955 ) ) ;
#25693=CARTESIAN_POINT ( 'NONE',  ( 19.88144391770000041, -18.50000000000000000, -7.765653790140000012 ) ) ;
#25695=CARTESIAN_POINT ( 'NONE',  ( -14.38874196869999977, -74.12911414260001663, 36.70801399449999991 ) ) ;
#25698=ORIENTED_EDGE ( 'NONE', *, *, #3312, .F. ) ;
#25699=CARTESIAN_POINT ( 'NONE',  ( -24.21840725559999896, -74.50000000000000000, -34.11790219230000076 ) ) ;
#25700=EDGE_CURVE ( 'NONE', #27727, #15327, #4875, .T. ) ;
#25701=FACE_OUTER_BOUND ( 'NONE', #25121, .T. ) ;
#25702=CARTESIAN_POINT ( 'NONE',  ( 34.06016921999999880, -74.00000000000000000, -9.364021409339999380 ) ) ;
#25703=CARTESIAN_POINT ( 'NONE',  ( 7.135467304789999687, -73.50000064450000536, -38.71640881029999548 ) ) ;
#25704=CARTESIAN_POINT ( 'NONE',  ( 21.30374392919999949, -60.30889230620000063, 10.62872870579999862 ) ) ;
#25705=DIRECTION ( 'NONE',  ( -0.2414462220490755096, 0.000000000000000000, 0.9704142011833032377 ) ) ;
#25706=CIRCLE ( 'NONE', #16853, 22.03370205219999889 ) ;
#25711=DIRECTION ( 'NONE',  ( 1.000000000000000000, 0.000000000000000000, 0.000000000000000000 ) ) ;
#25712=CARTESIAN_POINT ( 'NONE',  ( 23.14416696340000001, -57.40875702419999982, 10.37855830930000067 ) ) ;
#25717=CIRCLE ( 'NONE', #8027, 2.000000000000000000 ) ;
#25721=CIRCLE ( 'NONE', #13126, 30.50381168839999901 ) ;
#25723=DIRECTION ( 'NONE',  ( 0.000000000000000000, -1.000000000000000000, 0.000000000000000000 ) ) ;
#25725=CYLINDRICAL_SURFACE ( 'NONE', #20432, 7.249999999999999112 ) ;
#25730=CARTESIAN_POINT ( 'NONE',  ( -18.62649937282418833, -19.47440675035247537, 13.29909953111004661 ) ) ;
#25731=SPHERICAL_SURFACE ( 'NONE', #7712, 2.000000494509999616 ) ;
#25734=EDGE_CURVE ( 'NONE', #6019, #5317, #11358, .T. ) ;
#25735=CARTESIAN_POINT ( 'NONE',  ( -10.76213870606590106, -31.71488124271929010, 19.71543491739382148 ) ) ;
#25738=EDGE_CURVE ( 'NONE', #6357, #20759, #26880, .T. ) ;
#25742=CARTESIAN_POINT ( 'NONE',  ( -0.8576412294919999457, -60.34598855900000558, -23.61251632689999980 ) ) ;
#25743=CARTESIAN_POINT ( 'NONE',  ( 11.17657069110000023, -36.00000000000000000, -21.93565779399999727 ) ) ;
#25746=CARTESIAN_POINT ( 'NONE',  ( 19.90742232022705593, -19.48077950575742534, -8.670048025615079368 ) ) ;
#25749=FACE_OUTER_BOUND ( 'NONE', #960, .T. ) ;
#25750=ORIENTED_EDGE ( 'NONE', *, *, #14580, .F. ) ;
#25752=CARTESIAN_POINT ( 'NONE',  ( 8.611797725689999794, -36.09912295260000548, -20.95164070679999924 ) ) ;
#25754=CARTESIAN_POINT ( 'NONE',  ( -17.66077618279999939, -18.50000000000000000, 11.53219880630000205 ) ) ;
#25755=ORIENTED_EDGE ( 'NONE', *, *, #23432, .T. ) ;
#25758=CARTESIAN_POINT ( 'NONE',  ( 24.42476877459999685, -57.44036991850000362, 1.191907264949999989 ) ) ;
#25764=CARTESIAN_POINT ( 'NONE',  ( -2.714023266239999899, -18.86472494550000079, -23.42183169720000180 ) ) ;
#25766=VERTEX_POINT ( 'NONE', #20015 ) ;
#25768=CIRCLE ( 'NONE', #24834, 7.750000000000000000 ) ;
#25770=CARTESIAN_POINT ( 'NONE',  ( 21.79230230059999940, -37.95144147500000287, -8.472395268590000583 ) ) ;
#25771=CARTESIAN_POINT ( 'NONE',  ( 7.472970580910000216, -74.00000000000000000, 38.65569705749999940 ) ) ;
#25776=VECTOR ( 'NONE', #22128, 1000.000000000000000 ) ;
#25777=CARTESIAN_POINT ( 'NONE',  ( -0.3844954875762284785, -79.64723206074855000, 47.24135775273278171 ) ) ;
#25782=CARTESIAN_POINT ( 'NONE',  ( 20.84246830320000043, -57.47571038090000428, 10.69856926729999991 ) ) ;
#25784=ORIENTED_EDGE ( 'NONE', *, *, #5181, .F. ) ;
#25786=CARTESIAN_POINT ( 'NONE',  ( 47.25000000000000000, -75.00000000000000000, -1.245115460929999944E-12 ) ) ;
#25789=CARTESIAN_POINT ( 'NONE',  ( -27.40038777100000189, -74.50000000000000000, -36.59277592640000165 ) ) ;
#25791=CARTESIAN_POINT ( 'NONE',  ( 25.54297693993040141, -68.05277662258636440, 10.87142178243190038 ) ) ;
#25796=B_SPLINE_CURVE_WITH_KNOTS ( 'NONE', 5,
 ( #23077, #22783, #18701, #18552, #21032, #3122 ),
 .UNSPECIFIED., .F., .F.,
 ( 6, 6 ),
 ( 0.000000000000000000, 1.000000000000000000 ),
 .UNSPECIFIED. ) ;
#25798=CARTESIAN_POINT ( 'NONE',  ( -2.495716009659999735, -52.58489974430000302, -24.49317771890000017 ) ) ;
#25799=EDGE_CURVE ( 'NONE', #7849, #6001, #17987, .T. ) ;
#25800=AXIS2_PLACEMENT_3D ( 'NONE', #20572, #637, #9486 ) ;
#25804=EDGE_CURVE ( 'NONE', #2204, #3141, #16697, .T. ) ;
#25805=DIRECTION ( 'NONE',  ( 0.000000000000000000, -1.000000000000000000, 0.000000000000000000 ) ) ;
#25806=CIRCLE ( 'NONE', #22564, 3.750000000000000000 ) ;
#25809=CARTESIAN_POINT ( 'NONE',  ( 30.93662943959999723, -73.65801418129998979, -23.56172310960000260 ) ) ;
#25810=CARTESIAN_POINT ( 'NONE',  ( -14.15153136323935712, -74.02196623412419285, 36.23089701056277789 ) ) ;
#25811=EDGE_CURVE ( 'NONE', #5636, #12207, #19742, .T. ) ;
#25813=VERTEX_POINT ( 'NONE', #3416 ) ;
#25815=CARTESIAN_POINT ( 'NONE',  ( 21.29302206940000275, -35.50409515829999663, -7.872116142319999454 ) ) ;
#25816=CARTESIAN_POINT ( 'NONE',  ( 20.93196326829999876, -36.02994400500000438, -8.585833128470001796 ) ) ;
#25822=ORIENTED_EDGE ( 'NONE', *, *, #14056, .F. ) ;
#25823=TOROIDAL_SURFACE ( 'NONE', #25386, 6.750000000000000000, 0.5000000000000000000 ) ;
#25828=ORIENTED_EDGE ( 'NONE', *, *, #21446, .T. ) ;
#25831=CARTESIAN_POINT ( 'NONE',  ( 39.75929607687058365, -73.82871504776804272, 7.246063797165944287 ) ) ;
#25832=ORIENTED_EDGE ( 'NONE', *, *, #27781, .F. ) ;
#25834=CARTESIAN_POINT ( 'NONE',  ( 47.24999999999992184, -74.77408259042933025, -0.4803890690156943921 ) ) ;
#25835=CARTESIAN_POINT ( 'NONE',  ( -14.43678919070000077, -74.15747494800001505, 36.75078895099999698 ) ) ;
#25836=CARTESIAN_POINT ( 'NONE',  ( 1.598721155460000041E-15, -84.50000000000000000, -1.998401444329999950E-16 ) ) ;
#25840=CARTESIAN_POINT ( 'NONE',  ( -2.645751311070000167, -74.00000000000000000, 46.75000000000000000 ) ) ;
#25842=CARTESIAN_POINT ( 'NONE',  ( 9.386750785949999454, -63.25416415669999992, -23.64765651129999924 ) ) ;
#25844=CARTESIAN_POINT ( 'NONE',  ( 21.08560127379999827, -57.47122586340000083, 10.49905553490000187 ) ) ;
#25847=ADVANCED_FACE ( 'NONE', ( #3139 ), #14181, .T. ) ;
#25850=CARTESIAN_POINT ( 'NONE',  ( -9.476764215410000247, -74.50000000000000000, -38.08875739639999836 ) ) ;
#25851=CARTESIAN_POINT ( 'NONE',  ( 23.53639228501841174, -61.46980192603786008, 10.55322908533638859 ) ) ;
#25855=CARTESIAN_POINT ( 'NONE',  ( 9.564509902230000193, -57.40875702419999982, -23.52622212079999997 ) ) ;
#25857=ORIENTED_EDGE ( 'NONE', *, *, #24306, .T. ) ;
#25858=CARTESIAN_POINT ( 'NONE',  ( 7.426814492070000107, -35.28814190290000141, -21.34788074219999743 ) ) ;
#25863=CIRCLE ( 'NONE', #13275, 10.50000000000000000 ) ;
#25865=CARTESIAN_POINT ( 'NONE',  ( 27.75394116159999669, -74.50000000000000000, -27.75394116159999669 ) ) ;
#25866=EDGE_CURVE ( 'NONE', #25229, #11676, #28117, .T. ) ;
#25868=B_SPLINE_CURVE_WITH_KNOTS ( 'NONE', 3,
 ( #6675, #11455, #15686, #24593 ),
 .UNSPECIFIED., .F., .F.,
 ( 4, 4 ),
 ( 0.000000000000000000, 1.000000000000000000 ),
 .UNSPECIFIED. ) ;
#25870=CARTESIAN_POINT ( 'NONE',  ( -19.09898282842726047, -19.48685756512668732, 14.00485772877497048 ) ) ;
#25875=ORIENTED_EDGE ( 'NONE', *, *, #5632, .T. ) ;
#25876=CARTESIAN_POINT ( 'NONE',  ( 9.450751860034793950, -35.99944170493491669, -19.99269604853717297 ) ) ;
#25878=B_SPLINE_CURVE_WITH_KNOTS ( 'NONE', 3,
 ( #26553, #15454, #22481, #7037, #2089, #52 ),
 .UNSPECIFIED., .F., .F.,
 ( 4, 2, 4 ),
 ( 0.000000000000000000, 0.5000000000000000000, 1.000000000000000000 ),
 .UNSPECIFIED. ) ;
#25879=CARTESIAN_POINT ( 'NONE',  ( -0.6273717453279999967, -62.97603269449999885, -24.27362655359999977 ) ) ;
#25883=ORIENTED_EDGE ( 'NONE', *, *, #7993, .F. ) ;
#25885=ADVANCED_FACE ( 'NONE', ( #12281 ), #19281, .F. ) ;
#25888=EDGE_LOOP ( 'NONE', ( #12042, #10568, #27898, #23588 ) ) ;
#25890=LINE ( 'NONE', #13036, #26107 ) ;
#25891=CARTESIAN_POINT ( 'NONE',  ( 23.36166352360000076, -57.47815920179999694, -0.2645301549009999587 ) ) ;
#25895=CARTESIAN_POINT ( 'NONE',  ( 38.08875739639999836, -74.50000000000000000, 9.476764215410000247 ) ) ;
#25897=CARTESIAN_POINT ( 'NONE',  ( -0.5853288072829999633, -19.15810970359999743, -22.01520171810000193 ) ) ;
#25900=B_SPLINE_CURVE_WITH_KNOTS ( 'NONE', 5,
 ( #7758, #21279, #3241, #27982, #12098, #21011 ),
 .UNSPECIFIED., .F., .F.,
 ( 6, 6 ),
 ( 0.000000000000000000, 1.000000000000000000 ),
 .UNSPECIFIED. ) ;
#25901=CARTESIAN_POINT ( 'NONE',  ( -12.24789267329999909, -65.07443093669999712, 21.96586363990000024 ) ) ;
#25902=CARTESIAN_POINT ( 'NONE',  ( -31.99545665129999961, -74.00000000000000000, -22.01100727640000088 ) ) ;
#25903=CARTESIAN_POINT ( 'NONE',  ( 47.25000000000000000, -75.00000000000000000, -1.245115460929999944E-12 ) ) ;
#25904=ORIENTED_EDGE ( 'NONE', *, *, #19562, .F. ) ;
#25907=DIRECTION ( 'NONE',  ( -0.000000000000000000, 1.000000000000000000, 0.000000000000000000 ) ) ;
#25910=ORIENTED_EDGE ( 'NONE', *, *, #8370, .F. ) ;
#25911=B_SPLINE_CURVE_WITH_KNOTS ( 'NONE', 5,
 ( #11685, #15915, #11535, #24670, #20291, #16061 ),
 .UNSPECIFIED., .F., .F.,
 ( 6, 6 ),
 ( 0.000000000000000000, 1.000000000000000000 ),
 .UNSPECIFIED. ) ;
#25913=CARTESIAN_POINT ( 'NONE',  ( 10.20110288159999890, -74.50000000000000000, -41.00000000000000000 ) ) ;
#25914=CARTESIAN_POINT ( 'NONE',  ( -7.627568735119999666, -74.00000000000000000, -38.62788659690000515 ) ) ;
#25916=EDGE_CURVE ( 'NONE', #13332, #3865, #25392, .T. ) ;
#25917=CARTESIAN_POINT ( 'NONE',  ( 9.644866014229998896, -36.00000000000000000, -20.16453884109999706 ) ) ;
#25920=DIRECTION ( 'NONE',  ( 0.000000000000000000, -1.000000000000000000, 0.000000000000000000 ) ) ;
#25921=EDGE_CURVE ( 'NONE', #9163, #7997, #23309, .T. ) ;
#25923=CARTESIAN_POINT ( 'NONE',  ( -3.610293368829999849, -18.50000000000000000, -24.43613445369999937 ) ) ;
#25925=EDGE_CURVE ( 'NONE', #9200, #8106, #24704, .T. ) ;
#25926=CARTESIAN_POINT ( 'NONE',  ( 25.27264893869653051, -64.89166019501105609, 0.6762966387480369157 ) ) ;
#25930=CARTESIAN_POINT ( 'NONE',  ( -2.664535259099999805E-15, -72.00000000000000000, -3.552713678799999608E-15 ) ) ;
#25931=CIRCLE ( 'NONE', #12872, 7.750000000000000000 ) ;
#25932=CARTESIAN_POINT ( 'NONE',  ( -2.939806355540000027, -80.25752946859999781, 46.70460469590000230 ) ) ;
#25933=CARTESIAN_POINT ( 'NONE',  ( -19.23405768510000158, -19.49009541670000445, 14.16176834190000022 ) ) ;
#25934=ORIENTED_EDGE ( 'NONE', *, *, #7215, .T. ) ;
#25938=CARTESIAN_POINT ( 'NONE',  ( 19.42375544529999942, -18.50000000000000000, 8.976408266139999981 ) ) ;
#25940=DIRECTION ( 'NONE',  ( 1.000000000000000000, 0.000000000000000000, 0.000000000000000000 ) ) ;
#25944=CARTESIAN_POINT ( 'NONE',  ( 20.62428382529999737, -35.57628701899999868, -8.744932029230000126 ) ) ;
#25947=CARTESIAN_POINT ( 'NONE',  ( 21.46963261560000191, -36.58933600920000373, -7.659111216379999476 ) ) ;
#25951=EDGE_CURVE ( 'NONE', #10333, #5430, #10693, .T. ) ;
#25953=DIRECTION ( 'NONE',  ( -1.738658080639908902E-17, 0.000000000000000000, 1.000000000000000000 ) ) ;
#25956=FACE_OUTER_BOUND ( 'NONE', #5214, .T. ) ;
#25958=VERTEX_POINT ( 'NONE', #1790 ) ;
#25963=CARTESIAN_POINT ( 'NONE',  ( 39.79858521549137151, -73.85166138343194575, 7.247217007256502974 ) ) ;
#25964=ORIENTED_EDGE ( 'NONE', *, *, #26020, .T. ) ;
#25965=CARTESIAN_POINT ( 'NONE',  ( -14.52836087100000029, -74.22231530550000400, 36.83217634790000261 ) ) ;
#25966=CARTESIAN_POINT ( 'NONE',  ( -14.64485457939999868, -74.39167553240000075, 36.47327398630000062 ) ) ;
#25973=CARTESIAN_POINT ( 'NONE',  ( 23.23309162749999857, -57.41957467990000197, -9.464546293550000655 ) ) ;
#25975=CARTESIAN_POINT ( 'NONE',  ( 22.57886154579999882, -57.83919435140000331, 10.16307356839999798 ) ) ;
#25976=CARTESIAN_POINT ( 'NONE',  ( -10.40309664509999976, -19.44965585980000000, -20.22773501060000001 ) ) ;
#25980=CIRCLE ( 'NONE', #13407, 7.249999999999999112 ) ;
#25981=CARTESIAN_POINT ( 'NONE',  ( -2.664535259099999805E-15, -72.82938648530000592, -3.552713678799999608E-15 ) ) ;
#25982=CARTESIAN_POINT ( 'NONE',  ( 21.02965361369999897, -18.50000000000000000, -0.4426258060200000122 ) ) ;
#25983=ADVANCED_FACE ( 'NONE', ( #1378 ), #20163, .F. ) ;
#25990=ORIENTED_EDGE ( 'NONE', *, *, #4696, .F. ) ;
#25992=VERTEX_POINT ( 'NONE', #18057 ) ;
#25993=EDGE_CURVE ( 'NONE', #20928, #4268, #9303, .T. ) ;
#25995=CARTESIAN_POINT ( 'NONE',  ( -11.40415961587557447, -19.46574740001101844, 19.06929969032851346 ) ) ;
#25997=DIRECTION ( 'NONE',  ( 0.000000000000000000, 1.000000000000000000, 0.000000000000000000 ) ) ;
#25999=CIRCLE ( 'NONE', #24614, 1.999999999999998002 ) ;
#26000=CARTESIAN_POINT ( 'NONE',  ( -22.62751353610000393, -71.52549858170000618, 16.81410928309999875 ) ) ;
#26002=CARTESIAN_POINT ( 'NONE',  ( 9.885503723209998483, -36.00000000000000000, -20.33566493420000043 ) ) ;
#26003=CARTESIAN_POINT ( 'NONE',  ( 3.552713678799999608E-15, -18.50000000000000000, 3.552713678799999608E-15 ) ) ;
#26004=CARTESIAN_POINT ( 'NONE',  ( 7.365644968139999804, -35.41472402500000527, -21.38036730929999862 ) ) ;
#26006=ORIENTED_EDGE ( 'NONE', *, *, #4407, .F. ) ;
#26007=CARTESIAN_POINT ( 'NONE',  ( 8.011707311729999503, -18.50000000000000000, -19.70300569300000149 ) ) ;
#26011=DIRECTION ( 'NONE',  ( 0.9704142011833034598, 0.000000000000000000, -0.2414462220490750932 ) ) ;
#26012=CARTESIAN_POINT ( 'NONE',  ( -2.003725483539999797, -63.79833278959999632, -24.98874254210000245 ) ) ;
#26016=CYLINDRICAL_SURFACE ( 'NONE', #1106, 3.000000000000001332 ) ;
#26018=AXIS2_PLACEMENT_3D ( 'NONE', #6275, #15141, #4089 ) ;
#26019=ADVANCED_FACE ( 'NONE', ( #2481 ), #4193, .T. ) ;
#26020=EDGE_CURVE ( 'NONE', #24085, #15706, #12124, .T. ) ;
#26022=ORIENTED_EDGE ( 'NONE', *, *, #21578, .F. ) ;
#26023=B_SPLINE_CURVE_WITH_KNOTS ( 'NONE', 3,
 ( #16096, #13321, #2715, #6791, #13625, #20037, #20480, #9394, #4451, #26758, #15654, #11424, #22224, #27044, #18301, #2272, #24555, #11569, #20325, #24856, #2425, #396, #9245, #24996, #25306, #20926, #16675, #14222, #3431, #27766, #3154, #16544 ),
 .UNSPECIFIED., .F., .F.,
 ( 4, 2, 2, 1, 1, 1, 1, 1, 2, 2, 2, 2, 1, 1, 1, 1, 1, 2, 2, 2, 4 ),
 ( 0.000000000000000000, 0.1249999999999014400, 0.1874999999998525624, 0.2187499999998276379, 0.2343749999998150091, 0.2421874999998090416, 0.2460937499998054057, 0.2480468749998035738, 0.2490234374998036015, 0.2499999999998036015, 0.3749999999998803735, 0.4374999999999194533, 0.4687499999999386047, 0.4843749999999479861, 0.4921874999999526490, 0.4960937499999552025, 0.4980468749999555911, 0.4990234374999557576, 0.4999999999999559241, 0.7499999999999779066, 1.000000000000000000 ),
 .UNSPECIFIED. ) ;
#26025=CARTESIAN_POINT ( 'NONE',  ( -13.49470513559979956, -57.43018267548258393, 20.74700234779956887 ) ) ;
#26027=CARTESIAN_POINT ( 'NONE',  ( 8.782858223105064255, -69.73938810552070322, -25.82417951732658423 ) ) ;
#26028=CARTESIAN_POINT ( 'NONE',  ( -18.46133609720000024, -18.50000000000000000, 14.80231853080000093 ) ) ;
#26030=CARTESIAN_POINT ( 'NONE',  ( -19.73288567159999829, -59.03018501249999872, 12.72771757599999987 ) ) ;
#26031=ORIENTED_EDGE ( 'NONE', *, *, #10958, .F. ) ;
#26038=AXIS2_PLACEMENT_3D ( 'NONE', #11770, #7422, #595 ) ;
#26041=CARTESIAN_POINT ( 'NONE',  ( -32.33633361700000108, -74.08184093439999174, -21.99126984970000365 ) ) ;
#26043=ORIENTED_EDGE ( 'NONE', *, *, #14157, .F. ) ;
#26044=CARTESIAN_POINT ( 'NONE',  ( 36.90247978408418561, -79.73079169351882456, -14.43263691159852158 ) ) ;
#26046=CARTESIAN_POINT ( 'NONE',  ( -1.791418428495746618, -80.15006986280296530, 47.02519385070965541 ) ) ;
#26047=ORIENTED_EDGE ( 'NONE', *, *, #21490, .F. ) ;
#26048=CARTESIAN_POINT ( 'NONE',  ( 3.393335959449999838E-15, -69.50000000000000000, 46.75000000000000000 ) ) ;
#26049=DIRECTION ( 'NONE',  ( 1.000000000000000000, 0.000000000000000000, 0.000000000000000000 ) ) ;
#26050=ORIENTED_EDGE ( 'NONE', *, *, #24881, .T. ) ;
#26055=CARTESIAN_POINT ( 'NONE',  ( 22.96193664179805793, -37.37167648649992913, -9.452942635469471000 ) ) ;
#26056=VECTOR ( 'NONE', #9469, 1000.000000000000000 ) ;
#26058=LINE ( 'NONE', #12913, #20438 ) ;
#26059=FACE_OUTER_BOUND ( 'NONE', #27272, .T. ) ;
#26061=CARTESIAN_POINT ( 'NONE',  ( -3.588515834300000318, -18.50000000000000000, -23.38914531389999851 ) ) ;
#26062=VERTEX_POINT ( 'NONE', #12209 ) ;
#26065=DIRECTION ( 'NONE',  ( 1.000000000000000000, 0.000000000000000000, 0.000000000000000000 ) ) ;
#26068=CARTESIAN_POINT ( 'NONE',  ( 10.74178339546501348, -72.55263011558345454, -26.81973417036990526 ) ) ;
#26076=CARTESIAN_POINT ( 'NONE',  ( -14.05182617927096977, -69.64987745509210981, 23.32999788250410589 ) ) ;
#26080=VECTOR ( 'NONE', #6432, 1000.000000000000000 ) ;
#26082=ADVANCED_FACE ( 'NONE', ( #17014 ), #13510, .T. ) ;
#26084=ORIENTED_EDGE ( 'NONE', *, *, #27665, .F. ) ;
#26085=CARTESIAN_POINT ( 'NONE',  ( 21.44286899589999962, -36.30033507760000333, -7.882324037790000126 ) ) ;
#26087=CARTESIAN_POINT ( 'NONE',  ( 21.40156196539999911, -36.43444512949999847, -7.913580641820001205 ) ) ;
#26089=ORIENTED_EDGE ( 'NONE', *, *, #23094, .F. ) ;
#26094=CARTESIAN_POINT ( 'NONE',  ( 7.317502146920000783, -53.29669431050000128, -22.03392159830000097 ) ) ;
#26098=ORIENTED_EDGE ( 'NONE', *, *, #20468, .F. ) ;
#26099=AXIS2_PLACEMENT_3D ( 'NONE', #14849, #12379, #12655 ) ;
#26101=AXIS2_PLACEMENT_3D ( 'NONE', #20120, #18528, #2657 ) ;
#26102=CARTESIAN_POINT ( 'NONE',  ( 22.90398887539999961, -42.27112620169999957, 0.07876620758919998522 ) ) ;
#26103=CARTESIAN_POINT ( 'NONE',  ( 23.75597685949999871, -64.47176800949999631, 10.65806687269999919 ) ) ;
#26104=CARTESIAN_POINT ( 'NONE',  ( 47.25000000000000000, -74.50000000000000000, 2.433892081919999696E-15 ) ) ;
#26105=VERTEX_POINT ( 'NONE', #12474 ) ;
#26106=CARTESIAN_POINT ( 'NONE',  ( -39.03055149349999908, -74.00035141509999903, 7.562763921490000207 ) ) ;
#26107=VECTOR ( 'NONE', #8665, 1000.000000000000000 ) ;
#26108=FACE_OUTER_BOUND ( 'NONE', #5106, .T. ) ;
#26112=CARTESIAN_POINT ( 'NONE',  ( -1.606089563071368298, -74.11252154793176317, 47.07538657613434196 ) ) ;
#26114=CARTESIAN_POINT ( 'NONE',  ( 9.477371851879999198, -58.85143836710000187, -23.27434801040000067 ) ) ;
#26115=CARTESIAN_POINT ( 'NONE',  ( -12.78424652700000053, -68.56882598480000013, -23.49261584819999982 ) ) ;
#26116=CARTESIAN_POINT ( 'NONE',  ( 21.64704464699999775, -57.88555731719999642, 10.21083367329999980 ) ) ;
#26117=CARTESIAN_POINT ( 'NONE',  ( -10.44159655029999989, -19.42972408440000009, -20.93628310600000120 ) ) ;
#26118=ORIENTED_EDGE ( 'NONE', *, *, #7254, .T. ) ;
#26119=EDGE_CURVE ( 'NONE', #5636, #10192, #5520, .T. ) ;
#26124=CIRCLE ( 'NONE', #15884, 0.5000000000000004441 ) ;
#26125=AXIS2_PLACEMENT_3D ( 'NONE', #173, #22151, #26668 ) ;
#26128=CARTESIAN_POINT ( 'NONE',  ( 46.25000000000000000, -79.00000000000000000, -13.75000000000000000 ) ) ;
#26129=CARTESIAN_POINT ( 'NONE',  ( 23.42054537965112715, -60.74944441296194242, 10.50581986722356831 ) ) ;
#26130=CARTESIAN_POINT ( 'NONE',  ( 7.627568735119999666, -74.00000000000000000, 38.62788659690000515 ) ) ;
#26133=B_SPLINE_SURFACE_WITH_KNOTS ( 'NONE', 5, 5, ( 
 ( #23105, #3423, #9536, #1120, #9823, #7527 ),
 ( #12147, #18875, #14484, #11865, #12288, #18732 ),
 ( #24988, #18439, #832, #12003, #14347, #18291 ),
 ( #9674, #7367, #18585, #27760, #23242, #9388 ),
 ( #7796, #541, #11714, #2855, #22965, #7670 ),
 ( #13911, #27181, #7221, #16384, #20918, #5461 ) ),
 .UNSPECIFIED., .F., .F., .F.,
 ( 6, 6 ),
 ( 6, 6 ),
 ( 0.000000000000000000, 1.134864905219999942 ),
 ( 0.000000000000000000, 2.000000000000000000 ),
 .UNSPECIFIED. ) ;
#26134=CARTESIAN_POINT ( 'NONE',  ( 21.10194156680000077, -31.56454113959999930, -7.680651150220001000 ) ) ;
#26136=CARTESIAN_POINT ( 'NONE',  ( -35.88566914520000495, -79.50000000000000000, -26.69328098980000163 ) ) ;
#26137=ORIENTED_EDGE ( 'NONE', *, *, #4169, .T. ) ;
#26138=CARTESIAN_POINT ( 'NONE',  ( 40.00000000000000000, -80.00000000000000000, 5.426760838410000257E-16 ) ) ;
#26140=VERTEX_POINT ( 'NONE', #25901 ) ;
#26141=DIRECTION ( 'NONE',  ( 0.9952295494196653491, 0.000000000000000000, -0.09756097560976997873 ) ) ;
#26144=CARTESIAN_POINT ( 'NONE',  ( 22.19353322110000093, -19.46528100780000159, 0.3620904308219999868 ) ) ;
#26152=CARTESIAN_POINT ( 'NONE',  ( -22.33897789299999914, -68.90459131420000460, 16.95310341020000067 ) ) ;
#26156=CARTESIAN_POINT ( 'NONE',  ( -19.11972945367608645, -19.48733830559194047, 14.02465414947584499 ) ) ;
#26157=CARTESIAN_POINT ( 'NONE',  ( 7.151042947790000603, -36.56947956750000372, -21.49478542010000126 ) ) ;
#26159=ORIENTED_EDGE ( 'NONE', *, *, #21609, .T. ) ;
#26161=FACE_OUTER_BOUND ( 'NONE', #10029, .T. ) ;
#26163=CARTESIAN_POINT ( 'NONE',  ( 21.02691855299999801, -36.00000000000000000, -10.65875727889999958 ) ) ;
#26165=EDGE_LOOP ( 'NONE', ( #8677, #23808 ) ) ;
#26166=AXIS2_PLACEMENT_3D ( 'NONE', #8376, #17282, #12875 ) ;
#26167=CARTESIAN_POINT ( 'NONE',  ( -1.469715598349999874, -62.89113864609998927, -24.38506619410000198 ) ) ;
#26169=CARTESIAN_POINT ( 'NONE',  ( -19.52688526260000046, -53.83744478090000030, 12.95367122460000076 ) ) ;
#26172=FACE_BOUND ( 'NONE', #21499, .T. ) ;
#26176=CARTESIAN_POINT ( 'NONE',  ( -14.42818049519999946, -79.93744130869998799, 36.87246981650000777 ) ) ;
#26177=CARTESIAN_POINT ( 'NONE',  ( -17.53900985619999631, -18.50000000000000000, 11.92518103370000127 ) ) ;
#26178=CARTESIAN_POINT ( 'NONE',  ( 22.47829353779999906, -18.50000000000000000, 9.108151049139999955 ) ) ;
#26179=CARTESIAN_POINT ( 'NONE',  ( -20.11613068700000184, -58.88287621140000283, 14.48562127070000116 ) ) ;
#26180=ORIENTED_EDGE ( 'NONE', *, *, #10431, .T. ) ;
#26183=AXIS2_PLACEMENT_3D ( 'NONE', #6336, #13023, #17423 ) ;
#26184=FACE_OUTER_BOUND ( 'NONE', #5121, .T. ) ;
#26189=CARTESIAN_POINT ( 'NONE',  ( 10.62674045640880216, -67.15683218464279491, -25.79505860454265687 ) ) ;
#26190=CARTESIAN_POINT ( 'NONE',  ( -32.70383663730000734, -74.35538279870000622, -22.12063385180000097 ) ) ;
#26191=CARTESIAN_POINT ( 'NONE',  ( -22.49429811570129445, -79.94329726548942006, -32.72109705105904709 ) ) ;
#26193=ADVANCED_FACE ( 'NONE', ( #9881 ), #7936, .T. ) ;
#26196=CARTESIAN_POINT ( 'NONE',  ( 36.83926799238049909, -79.61991127481498154, -14.53746107291068057 ) ) ;
#26198=CARTESIAN_POINT ( 'NONE',  ( -0.6973805902349998753, -64.04267428580000399, -24.66993619630000012 ) ) ;
#26201=VERTEX_POINT ( 'NONE', #14680 ) ;
#26202=CARTESIAN_POINT ( 'NONE',  ( 20.60654921680000129, -56.26681992150000156, 10.91941308990000081 ) ) ;
#26208=DIRECTION ( 'NONE',  ( 0.000000000000000000, 1.000000000000000000, 0.000000000000000000 ) ) ;
#26210=ORIENTED_EDGE ( 'NONE', *, *, #12606, .F. ) ;
#26211=DIRECTION ( 'NONE',  ( 0.000000000000000000, -1.000000000000000000, 0.000000000000000000 ) ) ;
#26213=CARTESIAN_POINT ( 'NONE',  ( 25.57708872518721677, -68.14490930545984781, 10.86928520380060448 ) ) ;
#26215=DIRECTION ( 'NONE',  ( 0.9952295494196654602, 0.000000000000000000, -0.09756097560976760563 ) ) ;
#26217=CARTESIAN_POINT ( 'NONE',  ( 40.00000000000000000, -74.50000000000000000, 2.433892081919999696E-15 ) ) ;
#26219=CARTESIAN_POINT ( 'NONE',  ( 9.809109244645568992, -72.81435126429835236, -26.94740971970348653 ) ) ;
#26220=CARTESIAN_POINT ( 'NONE',  ( -19.47573917819999778, -18.50000000000000000, 15.05374981759999997 ) ) ;
#26221=VERTEX_POINT ( 'NONE', #23995 ) ;
#26226=DIRECTION ( 'NONE',  ( 1.000000000000000000, 0.000000000000000000, 0.000000000000000000 ) ) ;
#26228=VECTOR ( 'NONE', #15442, 1000.000000000000000 ) ;
#26230=EDGE_CURVE ( 'NONE', #26524, #28514, #16312, .T. ) ;
#26231=DIRECTION ( 'NONE',  ( 0.4794255386042040601, 0.000000000000000000, 0.8775825618903720926 ) ) ;
#26232=VERTEX_POINT ( 'NONE', #14946 ) ;
#26234=CARTESIAN_POINT ( 'NONE',  ( 24.48469364033755369, -18.60777261479816502, 1.929692123232705558 ) ) ;
#26235=ORIENTED_EDGE ( 'NONE', *, *, #10146, .T. ) ;
#26236=CIRCLE ( 'NONE', #4849, 38.75000000000000000 ) ;
#26237=CARTESIAN_POINT ( 'NONE',  ( 19.61885648609999677, -35.93737992959999872, -9.235927176200000588 ) ) ;
#26238=DIRECTION ( 'NONE',  ( 1.000000000000000000, 0.000000000000000000, 0.000000000000000000 ) ) ;
#26245=EDGE_CURVE ( 'NONE', #18491, #8501, #5089, .T. ) ;
#26246=CARTESIAN_POINT ( 'NONE',  ( -13.17060483900000101, -68.28989248250000799, -23.12790341000000183 ) ) ;
#26247=CARTESIAN_POINT ( 'NONE',  ( 21.05852160049740007, -34.60505674903147622, -8.113043604740113324 ) ) ;
#26249=CARTESIAN_POINT ( 'NONE',  ( -11.21645807309999832, -18.61794787939999907, -18.51636674970000129 ) ) ;
#26251=ORIENTED_EDGE ( 'NONE', *, *, #11601, .F. ) ;
#26253=FACE_OUTER_BOUND ( 'NONE', #19372, .T. ) ;
#26254=CARTESIAN_POINT ( 'NONE',  ( 22.63432516710000186, -65.53445078089998788, 11.44777113809999847 ) ) ;
#26256=EDGE_LOOP ( 'NONE', ( #18001, #4664, #195, #4296 ) ) ;
#26259=CARTESIAN_POINT ( 'NONE',  ( -15.12141716809999892, -79.25000000000000000, 36.76146410070000314 ) ) ;
#26262=VERTEX_POINT ( 'NONE', #10556 ) ;
#26267=CARTESIAN_POINT ( 'NONE',  ( 22.59576895060000012, -58.24783479010000065, 10.17368905969999915 ) ) ;
#26268=CARTESIAN_POINT ( 'NONE',  ( 23.20779262239999596, -63.55510590220001177, -8.328310080079999622 ) ) ;
#26269=VERTEX_POINT ( 'NONE', #8674 ) ;
#26274=ORIENTED_EDGE ( 'NONE', *, *, #23120, .T. ) ;
#26276=DIRECTION ( 'NONE',  ( -1.000000000000000000, 0.000000000000000000, 0.000000000000000000 ) ) ;
#26277=CIRCLE ( 'NONE', #27221, 7.250000000000000000 ) ;
#26281=DIRECTION ( 'NONE',  ( 0.000000000000000000, 1.000000000000000000, 0.000000000000000000 ) ) ;
#26283=EDGE_LOOP ( 'NONE', ( #8821, #16543, #14571 ) ) ;
#26284=DIRECTION ( 'NONE',  ( 1.000000000000000000, 0.000000000000000000, 0.000000000000000000 ) ) ;
#26286=ORIENTED_EDGE ( 'NONE', *, *, #4342, .T. ) ;
#26291=CARTESIAN_POINT ( 'NONE',  ( 22.06586088140000257, -18.85531889179999965, 0.4226866750830000075 ) ) ;
#26292=CARTESIAN_POINT ( 'NONE',  ( 25.26718046270000073, -72.00000000000000000, 6.129403842640000377 ) ) ;
#26293=CARTESIAN_POINT ( 'NONE',  ( 23.97384489419999909, -61.60336911379999947, -9.719973047129998989 ) ) ;
#26294=DIRECTION ( 'NONE',  ( 0.000000000000000000, -1.000000000000000000, 0.000000000000000000 ) ) ;
#26299=ADVANCED_FACE ( 'NONE', ( #28786, #15373 ), #6662, .T. ) ;
#26302=DIRECTION ( 'NONE',  ( 0.000000000000000000, -1.000000000000000000, 0.000000000000000000 ) ) ;
#26303=CARTESIAN_POINT ( 'NONE',  ( -18.48968691509886852, -19.46809228177112772, 12.68623665592749639 ) ) ;
#26304=CARTESIAN_POINT ( 'NONE',  ( 7.670973119900000192, -34.59820496239999699, -21.21808926869999823 ) ) ;
#26305=CARTESIAN_POINT ( 'NONE',  ( 43.75000000000000000, -79.00000000000000000, 5.357814579270000097E-15 ) ) ;
#26306=ORIENTED_EDGE ( 'NONE', *, *, #5966, .F. ) ;
#26307=CARTESIAN_POINT ( 'NONE',  ( 8.528769598780000294, -19.47487093119999813, -20.20034766559999895 ) ) ;
#26309=ORIENTED_EDGE ( 'NONE', *, *, #21609, .F. ) ;
#26310=CARTESIAN_POINT ( 'NONE',  ( -2.595813266009999953, -59.99252585180000352, -25.40064173880000098 ) ) ;
#26312=CARTESIAN_POINT ( 'NONE',  ( -19.91989157560000123, -56.26715181569999658, 12.12299716169999897 ) ) ;
#26316=CARTESIAN_POINT ( 'NONE',  ( 7.248115061050000030, -74.24288085039999885, -40.37851622839999521 ) ) ;
#26317=VERTEX_POINT ( 'NONE', #26623 ) ;
#26319=EDGE_CURVE ( 'NONE', #5884, #27002, #20042, .T. ) ;
#26321=DIRECTION ( 'NONE',  ( -0.2414462220490753985, 0.000000000000000000, -0.9704142011833032377 ) ) ;
#26324=DIRECTION ( 'NONE',  ( 1.000000000000000000, 0.000000000000000000, 0.000000000000000000 ) ) ;
#26327=DIRECTION ( 'NONE',  ( 0.000000000000000000, -1.000000000000000000, 0.000000000000000000 ) ) ;
#26329=CARTESIAN_POINT ( 'NONE',  ( -14.65665286289999969, -74.50000000000000000, 36.94583910070000599 ) ) ;
#26333=CARTESIAN_POINT ( 'NONE',  ( -32.09164647010000238, -74.00884812510000188, -22.02207427699999798 ) ) ;
#26334=EDGE_LOOP ( 'NONE', ( #24602, #27592, #8753, #24587 ) ) ;
#26336=AXIS2_PLACEMENT_3D ( 'NONE', #16693, #713, #16558 ) ;
#26338=VERTEX_POINT ( 'NONE', #8544 ) ;
#26339=CARTESIAN_POINT ( 'NONE',  ( -19.95527577780000072, -57.47855601759999900, 12.14622656770000120 ) ) ;
#26341=VERTEX_POINT ( 'NONE', #21960 ) ;
#26343=FACE_OUTER_BOUND ( 'NONE', #18177, .T. ) ;
#26345=ORIENTED_EDGE ( 'NONE', *, *, #12586, .F. ) ;
#26347=CARTESIAN_POINT ( 'NONE',  ( -21.71458295470000266, -79.50000022099999342, -32.69645407760000211 ) ) ;
#26348=ADVANCED_FACE ( 'NONE', ( #19759 ), #13342, .T. ) ;
#26349=CARTESIAN_POINT ( 'NONE',  ( 8.645795245420000441, -37.33710341700000157, -21.88811428650000224 ) ) ;
#26351=CARTESIAN_POINT ( 'NONE',  ( -2.125583358770000153, -18.50000000000000000, -21.40767207160000396 ) ) ;
#26362=CARTESIAN_POINT ( 'NONE',  ( 7.992697598190521724, -57.47158968945384316, -22.16163068290176952 ) ) ;
#26364=CARTESIAN_POINT ( 'NONE',  ( 19.97770600910000027, -18.50000000000000000, 8.668758119890000557 ) ) ;
#26365=FACE_OUTER_BOUND ( 'NONE', #17057, .T. ) ;
#26366=B_SPLINE_SURFACE_WITH_KNOTS ( 'NONE', 5, 5, ( 
 ( #11612, #3194, #1030, #25040, #20524, #12052 ),
 ( #20819, #593, #23287, #3060, #9586, #9723 ),
 ( #25472, #9436, #18486, #5074, #20967, #22865 ),
 ( #5227, #18343, #5372, #27796, #16285, #14524 ),
 ( #5507, #16439, #7419, #13959, #25342, #25198 ),
 ( #14255, #10003, #9869, #7270, #18917, #18634 ) ),
 .UNSPECIFIED., .F., .F., .F.,
 ( 6, 6 ),
 ( 6, 6 ),
 ( 38.86449171000000291, 46.02720679840000173 ),
 ( 0.000000000000000000, 2.000000000000000000 ),
 .UNSPECIFIED. ) ;
#26369=CARTESIAN_POINT ( 'NONE',  ( 32.97008227039999895, -72.00000000000000000, -20.36016146999999776 ) ) ;
#26373=ORIENTED_EDGE ( 'NONE', *, *, #28400, .F. ) ;
#26374=CARTESIAN_POINT ( 'NONE',  ( 20.49450488670000325, -35.98895400249999454, -8.959583261280000599 ) ) ;
#26375=CARTESIAN_POINT ( 'NONE',  ( 7.730596333266516851, -19.15810973048309052, -20.62158076667584439 ) ) ;
#26376=EDGE_LOOP ( 'NONE', ( #17941, #8914, #11602, #20252 ) ) ;
#26379=EDGE_CURVE ( 'NONE', #9130, #5488, #2598, .T. ) ;
#26382=B_SPLINE_CURVE_WITH_KNOTS ( 'NONE', 5,
 ( #5374, #16289, #23012, #14257, #2758, #23151 ),
 .UNSPECIFIED., .F., .F.,
 ( 6, 6 ),
 ( 0.000000000000000000, 1.000000000000000000 ),
 .UNSPECIFIED. ) ;
#26384=CARTESIAN_POINT ( 'NONE',  ( 9.564509902250000195, -57.40875702419999982, -23.52622212079999997 ) ) ;
#26385=CARTESIAN_POINT ( 'NONE',  ( -10.96210381709999915, -19.46434222019999893, -19.17795744089999843 ) ) ;
#26387=ORIENTED_EDGE ( 'NONE', *, *, #4641, .F. ) ;
#26389=CARTESIAN_POINT ( 'NONE',  ( 24.50968349569999916, -49.82767789679999737, 1.331815368300000024 ) ) ;
#26390=CARTESIAN_POINT ( 'NONE',  ( 23.42457832669999718, -66.42763100729999337, 11.17107935629999993 ) ) ;
#26393=DIRECTION ( 'NONE',  ( 0.000000000000000000, 1.000000000000000000, 0.000000000000000000 ) ) ;
#26395=DIRECTION ( 'NONE',  ( -1.887379141859999978E-15, 0.000000000000000000, -1.000000000000000000 ) ) ;
#26396=ORIENTED_EDGE ( 'NONE', *, *, #8190, .T. ) ;
#26400=CARTESIAN_POINT ( 'NONE',  ( -40.65853658540000026, -84.00000000000000000, 6.717799458580000049 ) ) ;
#26401=CARTESIAN_POINT ( 'NONE',  ( -13.17786140689999819, -69.76368794990000310, -23.89400643789999990 ) ) ;
#26402=CARTESIAN_POINT ( 'NONE',  ( -9.476764215410000247, -82.25000000000000000, 38.08875739639999836 ) ) ;
#26403=TOROIDAL_SURFACE ( 'NONE', #13845, 39.75000000000000000, 0.5000000000000000000 ) ;
#26404=CARTESIAN_POINT ( 'NONE',  ( 22.72361805330000095, -62.11544144339999463, -7.859435617799999996 ) ) ;
#26406=CARTESIAN_POINT ( 'NONE',  ( -40.00000000000000000, -69.00000000000000000, 5.717648576820000312E-16 ) ) ;
#26417=CARTESIAN_POINT ( 'NONE',  ( 19.39107742150000036, -19.48263940080000012, -8.982220567580000647 ) ) ;
#26418=CARTESIAN_POINT ( 'NONE',  ( -9.476764215410000247, -82.25000000000000000, -38.08875739639999836 ) ) ;
#26422=CARTESIAN_POINT ( 'NONE',  ( 2.042810365310000056E-12, -74.50000000000000000, -2.458477865729999957E-12 ) ) ;
#26425=FACE_OUTER_BOUND ( 'NONE', #11695, .T. ) ;
#26427=ORIENTED_EDGE ( 'NONE', *, *, #23979, .T. ) ;
#26429=CARTESIAN_POINT ( 'NONE',  ( 28.97576656849999566, -36.00000000000000000, -19.97576656850000987 ) ) ;
#26430=CARTESIAN_POINT ( 'NONE',  ( -12.00629479391328225, -19.46993812760626952, 19.10789507585830194 ) ) ;
#26431=CARTESIAN_POINT ( 'NONE',  ( 25.26718046270000073, -18.50000000000000000, 6.129403842640000377 ) ) ;
#26433=AXIS2_PLACEMENT_3D ( 'NONE', #27589, #5562, #25255 ) ;
#26435=CARTESIAN_POINT ( 'NONE',  ( -16.67828388959999941, -80.00000000000000000, 44.75374114529999758 ) ) ;
#26436=CARTESIAN_POINT ( 'NONE',  ( 19.66445149499999800, -18.50000000000000000, -7.467233996350000069 ) ) ;
#26438=PRODUCT ( 'Water Pump Main Cast Housing', 'Water Pump Main Cast Housing', '', ( #18064 ) ) ;
#26441=CARTESIAN_POINT ( 'NONE',  ( 7.857545609690000710, -34.84004015499999696, -21.18059969839999823 ) ) ;
#26442=DIRECTION ( 'NONE',  ( 0.000000000000000000, 1.000000000000000000, 0.000000000000000000 ) ) ;
#26443=ORIENTED_EDGE ( 'NONE', *, *, #19304, .F. ) ;
#26444=CARTESIAN_POINT ( 'NONE',  ( 9.024081076579999916, -19.18584067659999803, -18.94592230760000007 ) ) ;
#26446=VECTOR ( 'NONE', #27802, 1000.000000000000000 ) ;
#26449=CARTESIAN_POINT ( 'NONE',  ( -12.06159505309999957, -57.47122572379999639, 20.23241877790000132 ) ) ;
#26450=B_SPLINE_CURVE_WITH_KNOTS ( 'NONE', 3,
 ( #7175, #27279, #7314, #24800, #11512, #11367 ),
 .UNSPECIFIED., .F., .F.,
 ( 4, 2, 4 ),
 ( 0.000000000000000000, 0.5000000000000000000, 1.000000000000000000 ),
 .UNSPECIFIED. ) ;
#26453=CARTESIAN_POINT ( 'NONE',  ( -19.61988232110000041, -56.24740423709999249, 13.61851891309999907 ) ) ;
#26457=VERTEX_POINT ( 'NONE', #27067 ) ;
#26458=LINE ( 'NONE', #28344, #16288 ) ;
#26459=CARTESIAN_POINT ( 'NONE',  ( 7.305188533800000883, -74.19145175580000284, -39.89376887110000069 ) ) ;
#26460=ORIENTED_EDGE ( 'NONE', *, *, #18441, .F. ) ;
#26461=CARTESIAN_POINT ( 'NONE',  ( -7.627568735119999666, -74.00000000000000000, 38.62788659690000515 ) ) ;
#26462=AXIS2_PLACEMENT_3D ( 'NONE', #24131, #13486, #17580 ) ;
#26463=DIRECTION ( 'NONE',  ( 0.000000000000000000, -1.000000000000000000, 0.000000000000000000 ) ) ;
#26465=CARTESIAN_POINT ( 'NONE',  ( 22.48256761629999900, -26.02764329579999725, 9.981120560429999955 ) ) ;
#26467=CARTESIAN_POINT ( 'NONE',  ( 10.10280028159999866, -66.03737782630000197, -24.89219399830000157 ) ) ;
#26469=CARTESIAN_POINT ( 'NONE',  ( -15.08135542264446016, -67.66819112664462921, 22.63088101126209040 ) ) ;
#26471=CARTESIAN_POINT ( 'NONE',  ( -7.226919149556380262, -73.65985332689392351, 39.42193790014463417 ) ) ;
#26472=CARTESIAN_POINT ( 'NONE',  ( 23.27528716992228297, -63.28488723400939620, -7.442304005261173749 ) ) ;
#26473=VERTEX_POINT ( 'NONE', #1813 ) ;
#26474=AXIS2_PLACEMENT_3D ( 'NONE', #28801, #4187, #24155 ) ;
#26476=CARTESIAN_POINT ( 'NONE',  ( -32.66462566889999408, -74.35538279870000622, -21.73251009970000069 ) ) ;
#26477=CARTESIAN_POINT ( 'NONE',  ( -22.37091525677837467, -79.85009384193479320, -32.77535131886410369 ) ) ;
#26478=ORIENTED_EDGE ( 'NONE', *, *, #234, .F. ) ;
#26484=B_SPLINE_CURVE_WITH_KNOTS ( 'NONE', 5,
 ( #17028, #12228, #25917, #21136, #19359, #21824 ),
 .UNSPECIFIED., .F., .F.,
 ( 6, 6 ),
 ( -3.225498864409999999, -2.709627234730000112 ),
 .UNSPECIFIED. ) ;
#26487=CARTESIAN_POINT ( 'NONE',  ( 41.00000000000000000, -80.00000000000000000, -10.20110288159999890 ) ) ;
#26490=DIRECTION ( 'NONE',  ( 1.000000000000000000, 0.000000000000000000, 0.000000000000000000 ) ) ;
#26496=CARTESIAN_POINT ( 'NONE',  ( 7.215414233289999757, -77.00000000000000000, -40.70731707320000226 ) ) ;
#26498=CIRCLE ( 'NONE', #1400, 7.250000000000000000 ) ;
#26499=TOROIDAL_SURFACE ( 'NONE', #23273, 39.75000000000000000, 0.5000000000000000000 ) ;
#26503=CARTESIAN_POINT ( 'NONE',  ( -0.5388777241750000169, -56.26715181569999658, -23.31263072600000186 ) ) ;
#26504=CARTESIAN_POINT ( 'NONE',  ( 21.32348952719999957, -36.24018116390000444, -9.136262768950000890 ) ) ;
#26505=DIRECTION ( 'NONE',  ( 0.4692400087391608854, 0.000000000000000000, -0.8830706733883039172 ) ) ;
#26507=CARTESIAN_POINT ( 'NONE',  ( -21.99985828019999801, -74.00000000000000000, -31.89935321680000158 ) ) ;
#26508=CARTESIAN_POINT ( 'NONE',  ( -7.615241770509999806E-12, -84.50000000000000000, -9.798384326129999571E-12 ) ) ;
#26510=CARTESIAN_POINT ( 'NONE',  ( 22.62497689329999773, -18.50000000000000000, 8.848724866619999574 ) ) ;
#26512=EDGE_CURVE ( 'NONE', #4763, #24745, #1435, .T. ) ;
#26516=CIRCLE ( 'NONE', #12122, 3.749999999999996447 ) ;
#26518=AXIS2_PLACEMENT_3D ( 'NONE', #11119, #18147, #13770 ) ;
#26519=EDGE_LOOP ( 'NONE', ( #9089, #532, #21537, #13278 ) ) ;
#26522=DIRECTION ( 'NONE',  ( 1.000000000000000000, 0.000000000000000000, 0.000000000000000000 ) ) ;
#26523=DIRECTION ( 'NONE',  ( 0.000000000000000000, -1.000000000000000000, 0.000000000000000000 ) ) ;
#26524=VERTEX_POINT ( 'NONE', #26429 ) ;
#26525=ORIENTED_EDGE ( 'NONE', *, *, #4603, .T. ) ;
#26527=CARTESIAN_POINT ( 'NONE',  ( 40.00000000000000000, -74.00000000000000000, 2.009834509230000106E-15 ) ) ;
#26533=CARTESIAN_POINT ( 'NONE',  ( 23.19209251300000219, -34.65282384500000035, 0.9632692026179999756 ) ) ;
#26534=CARTESIAN_POINT ( 'NONE',  ( -14.75020709650109474, -80.11189707592339460, 36.37309920249453654 ) ) ;
#26535=CARTESIAN_POINT ( 'NONE',  ( 40.26982517594145605, -74.16605908717274076, 7.244980372392263668 ) ) ;
#26538=CYLINDRICAL_SURFACE ( 'NONE', #13664, 7.249999999999999112 ) ;
#26540=DIRECTION ( 'NONE',  ( 1.000000000000000000, 0.000000000000000000, 0.000000000000000000 ) ) ;
#26541=ORIENTED_EDGE ( 'NONE', *, *, #742, .F. ) ;
#26543=CARTESIAN_POINT ( 'NONE',  ( 28.18645782309999959, -71.82886645399999281, 1.608671017380000068 ) ) ;
#26545=B_SPLINE_CURVE_WITH_KNOTS ( 'NONE', 5,
 ( #28288, #5592, #23370, #12406, #3965, #12826 ),
 .UNSPECIFIED., .F., .F.,
 ( 6, 6 ),
 ( 0.000000000000000000, 1.000000000000000000 ),
 .UNSPECIFIED. ) ;
#26547=CARTESIAN_POINT ( 'NONE',  ( 7.992697598190001251, -57.47158968939999824, -22.16163068290000027 ) ) ;
#26548=CARTESIAN_POINT ( 'NONE',  ( -25.98617420859999783, -74.50000000000000000, -36.59277592640000165 ) ) ;
#26549=CARTESIAN_POINT ( 'NONE',  ( -11.90992095799999895, -57.47815921199999423, -20.09952916750000185 ) ) ;
#26550=ORIENTED_EDGE ( 'NONE', *, *, #4914, .T. ) ;
#26551=ADVANCED_FACE ( 'NONE', ( #15626 ), #12563, .T. ) ;
#26552=ADVANCED_FACE ( 'NONE', ( #15474 ), #4562, .F. ) ;
#26553=CARTESIAN_POINT ( 'NONE',  ( 28.63360765790000073, -72.82938648530000592, 1.697648101029999967 ) ) ;
#26554=ADVANCED_FACE ( 'NONE', ( #19851 ), #23623, .T. ) ;
#26555=ORIENTED_EDGE ( 'NONE', *, *, #25362, .F. ) ;
#26562=VECTOR ( 'NONE', #22595, 1000.000000000000000 ) ;
#26563=CARTESIAN_POINT ( 'NONE',  ( 20.47344018690000311, -19.43778597749999903, -8.153551334750000379 ) ) ;
#26564=DIRECTION ( 'NONE',  ( 0.000000000000000000, -1.000000000000000000, 0.000000000000000000 ) ) ;
#26566=DIRECTION ( 'NONE',  ( 0.000000000000000000, 0.000000000000000000, -1.000000000000000000 ) ) ;
#26569=CARTESIAN_POINT ( 'NONE',  ( 7.659450882289999818, -36.59067043469999447, -21.46971212389999906 ) ) ;
#26571=CARTESIAN_POINT ( 'NONE',  ( -12.09704001540000107, -74.00000000000000000, 47.10905722069999513 ) ) ;
#26572=EDGE_CURVE ( 'NONE', #20017, #3141, #11250, .T. ) ;
#26574=CARTESIAN_POINT ( 'NONE',  ( -0.8216735279219999910, -65.07443093669999712, -25.13632616349999793 ) ) ;
#26577=CARTESIAN_POINT ( 'NONE',  ( -12.76410956269999986, -19.16887614239999849, 19.36424863110000061 ) ) ;
#26580=CARTESIAN_POINT ( 'NONE',  ( 36.24656966590000451, -75.00000018780001199, -15.05817676390000059 ) ) ;
#26581=CARTESIAN_POINT ( 'NONE',  ( 25.74462086831581686, -61.40640411929997100, 1.403327536049160607 ) ) ;
#26584=CARTESIAN_POINT ( 'NONE',  ( -14.40572000550000098, -18.50000000000000000, 20.06574520719999910 ) ) ;
#26586=VERTEX_POINT ( 'NONE', #522 ) ;
#26588=CARTESIAN_POINT ( 'NONE',  ( 8.979483994470001562, -19.17889721279999904, -19.39105717750000224 ) ) ;
#26590=CIRCLE ( 'NONE', #22345, 0.5000000000000027756 ) ;
#26591=B_SPLINE_CURVE_WITH_KNOTS ( 'NONE', 5,
 ( #14857, #24, #22296, #11645, #27119, #11798, #20256, #13843, #20403 ),
 .UNSPECIFIED., .F., .F.,
 ( 6, 3, 6 ),
 ( 0.000000000000000000, 0.5538417791012780755, 1.000000000000000000 ),
 .UNSPECIFIED. ) ;
#26592=CARTESIAN_POINT ( 'NONE',  ( 22.70474501079999641, -37.36473932629999695, -9.382534168720001233 ) ) ;
#26593=CARTESIAN_POINT ( 'NONE',  ( -11.45174903020000023, -57.47815880419999957, 20.36405811959999923 ) ) ;
#26594=CARTESIAN_POINT ( 'NONE',  ( 7.230685509108649711, -74.36482065571902922, 40.53346806358988630 ) ) ;
#26596=CARTESIAN_POINT ( 'NONE',  ( -19.65023616090000047, -56.26441942339999969, 12.67997976360000045 ) ) ;
#26597=DIRECTION ( 'NONE',  ( 0.000000000000000000, 1.000000000000000000, 0.000000000000000000 ) ) ;
#26598=VERTEX_POINT ( 'NONE', #13595 ) ;
#26604=AXIS2_PLACEMENT_3D ( 'NONE', #23483, #19104, #15259 ) ;
#26607=CARTESIAN_POINT ( 'NONE',  ( 22.31047812949999809, -45.95149559400000072, 9.984808736899998038 ) ) ;
#26611=CARTESIAN_POINT ( 'NONE',  ( -13.82310862910000004, -74.00000000000000000, 36.20061004779999791 ) ) ;
#26612=CARTESIAN_POINT ( 'NONE',  ( 9.264974235690001336, -69.68028691090000848, -25.63136490189999961 ) ) ;
#26614=ORIENTED_EDGE ( 'NONE', *, *, #14651, .F. ) ;
#26615=CARTESIAN_POINT ( 'NONE',  ( -41.00000000000000000, -74.50000000000000000, -10.20110288159999890 ) ) ;
#26616=DIRECTION ( 'NONE',  ( 0.2414462220490750377, 0.000000000000000000, -0.9704142011833034598 ) ) ;
#26617=CARTESIAN_POINT ( 'NONE',  ( -16.78865735879999832, -72.00000000000000000, 25.46808810279999946 ) ) ;
#26618=EDGE_CURVE ( 'NONE', #18811, #2130, #7347, .T. ) ;
#26620=CARTESIAN_POINT ( 'NONE',  ( 22.78912717118120668, -61.50656701021978279, -7.252352442454050419 ) ) ;
#26623=CARTESIAN_POINT ( 'NONE',  ( -32.39999999999999858, -89.50000000000000000, 0.000000000000000000 ) ) ;
#26624=CARTESIAN_POINT ( 'NONE',  ( -32.32698596700000593, -74.07302383969998516, -21.86563713199999981 ) ) ;
#26625=ORIENTED_EDGE ( 'NONE', *, *, #19347, .F. ) ;
#26626=AXIS2_PLACEMENT_3D ( 'NONE', #22370, #24847, #11562 ) ;
#26627=DIRECTION ( 'NONE',  ( 0.000000000000000000, -1.000000000000000000, 0.000000000000000000 ) ) ;
#26629=CARTESIAN_POINT ( 'NONE',  ( -0.5578430832430000263, -60.34941021230000047, -23.62008496760000043 ) ) ;
#26636=FACE_OUTER_BOUND ( 'NONE', #24053, .T. ) ;
#26637=CARTESIAN_POINT ( 'NONE',  ( 21.63571023749972255, -57.45864773928945368, 10.20337500119981300 ) ) ;
#26640=EDGE_CURVE ( 'NONE', #7572, #27321, #27056, .T. ) ;
#26642=AXIS2_PLACEMENT_3D ( 'NONE', #11419, #11112, #20321 ) ;
#26648=CARTESIAN_POINT ( 'NONE',  ( -21.94076895599999943, -74.04938808419998963, -32.26063837559999570 ) ) ;
#26649=CARTESIAN_POINT ( 'NONE',  ( -2.488381629190000055, -57.43018266639999325, -24.62423963640000224 ) ) ;
#26652=CARTESIAN_POINT ( 'NONE',  ( 11.38886874731390542, -72.26599441443077865, -27.01882936454276063 ) ) ;
#26653=CARTESIAN_POINT ( 'NONE',  ( 7.561767224756156480, -74.02518375726356226, -38.96762186395582006 ) ) ;
#26654=ORIENTED_EDGE ( 'NONE', *, *, #3347, .F. ) ;
#26655=EDGE_CURVE ( 'NONE', #21714, #300, #1925, .T. ) ;
#26656=DIRECTION ( 'NONE',  ( 0.000000000000000000, 1.000000000000000000, 0.000000000000000000 ) ) ;
#26657=CIRCLE ( 'NONE', #10815, 0.5000000000000027756 ) ;
#26658=DIRECTION ( 'NONE',  ( 0.000000000000000000, 1.000000000000000000, 0.000000000000000000 ) ) ;
#26660=FACE_OUTER_BOUND ( 'NONE', #15130, .T. ) ;
#26666=CARTESIAN_POINT ( 'NONE',  ( -7.325370793560000315, -18.50000000000000000, -24.94672208400000102 ) ) ;
#26667=ORIENTED_EDGE ( 'NONE', *, *, #11763, .F. ) ;
#26668=DIRECTION ( 'NONE',  ( 1.000000000000000000, 0.000000000000000000, 0.000000000000000000 ) ) ;
#26670=EDGE_LOOP ( 'NONE', ( #16137, #20200, #19789, #24353 ) ) ;
#26673=VERTEX_POINT ( 'NONE', #25124 ) ;
#26675=VERTEX_POINT ( 'NONE', #2984 ) ;
#26677=AXIS2_PLACEMENT_3D ( 'NONE', #14768, #16683, #14364 ) ;
#26680=DIRECTION ( 'NONE',  ( 1.000000000000000000, 0.000000000000000000, 0.000000000000000000 ) ) ;
#26681=CARTESIAN_POINT ( 'NONE',  ( 26.74759209541820226, -72.18155182615700483, -9.512885920061126654 ) ) ;
#26682=CARTESIAN_POINT ( 'NONE',  ( -10.20538995839999785, -18.50000000000000000, -19.00160311810000024 ) ) ;
#26683=CARTESIAN_POINT ( 'NONE',  ( 47.19235072946354137, -79.33463070164246744, -1.154528427232027310 ) ) ;
#26684=ORIENTED_EDGE ( 'NONE', *, *, #12967, .F. ) ;
#26685=EDGE_CURVE ( 'NONE', #16440, #2786, #5174, .T. ) ;
#26687=CARTESIAN_POINT ( 'NONE',  ( 23.35215130579999965, -19.42972408449999833, 1.425453684350000083 ) ) ;
#26688=CARTESIAN_POINT ( 'NONE',  ( -14.93114631064312547, -79.63213912887773915, 36.29908221780583943 ) ) ;
#26691=AXIS2_PLACEMENT_3D ( 'NONE', #27413, #25235, #3230 ) ;
#26695=VERTEX_POINT ( 'NONE', #8182 ) ;
#26697=CARTESIAN_POINT ( 'NONE',  ( 26.84355716949999859, -67.87585789450000107, 1.442240390609999867 ) ) ;
#26699=CARTESIAN_POINT ( 'NONE',  ( 20.36016146999999776, -74.00000000000000000, -32.97008227039999895 ) ) ;
#26701=CARTESIAN_POINT ( 'NONE',  ( -10.97403643530000039, -42.22519323619999909, -21.72972191419999888 ) ) ;
#26702=AXIS2_PLACEMENT_3D ( 'NONE', #23890, #26656, #21843 ) ;
#26704=CARTESIAN_POINT ( 'NONE',  ( -11.74919335509972207, -57.47571039348258637, 20.26880008289946034 ) ) ;
#26706=ORIENTED_EDGE ( 'NONE', *, *, #25325, .T. ) ;
#26708=CARTESIAN_POINT ( 'NONE',  ( 22.58609710640000046, -18.50000000000000000, 2.144703970959999761 ) ) ;
#26711=AXIS2_PLACEMENT_3D ( 'NONE', #9147, #17914, #6839 ) ;
#26714=CARTESIAN_POINT ( 'NONE',  ( 19.04514928800000106, -22.53353387550000164, -9.014749987960000155 ) ) ;
#26715=CARTESIAN_POINT ( 'NONE',  ( 22.03186001407977201, -19.46468284061640475, -0.3186543872829983859 ) ) ;
#26717=ORIENTED_EDGE ( 'NONE', *, *, #862, .T. ) ;
#26720=ORIENTED_EDGE ( 'NONE', *, *, #19109, .F. ) ;
#26721=CARTESIAN_POINT ( 'NONE',  ( 9.122466984649999944, -36.00948308300000633, -20.42228432030000107 ) ) ;
#26722=CARTESIAN_POINT ( 'NONE',  ( 8.458704334359074650, -19.47547933409599352, -20.16190868471589326 ) ) ;
#26724=EDGE_CURVE ( 'NONE', #26341, #1349, #8400, .T. ) ;
#26729=AXIS2_PLACEMENT_3D ( 'NONE', #6322, #26736, #13453 ) ;
#26733=CARTESIAN_POINT ( 'NONE',  ( -13.43613129169999887, -18.86819671679999999, 19.94230158159999888 ) ) ;
#26736=DIRECTION ( 'NONE',  ( -0.09756097560976716154, 0.000000000000000000, 0.9952295494196655712 ) ) ;
#26743=ORIENTED_EDGE ( 'NONE', *, *, #13024, .T. ) ;
#26744=CARTESIAN_POINT ( 'NONE',  ( 36.49273837329999992, -74.69502841160000628, -14.74290838079999943 ) ) ;
#26745=AXIS2_PLACEMENT_3D ( 'NONE', #25981, #10230, #1388 ) ;
#26749=CARTESIAN_POINT ( 'NONE',  ( -11.75563520630000092, -62.12690044249999488, 20.90240914950000217 ) ) ;
#26750=CARTESIAN_POINT ( 'NONE',  ( 7.241427273140969234, -74.22736093651798228, 40.35276762256386718 ) ) ;
#26755=CARTESIAN_POINT ( 'NONE',  ( -11.22183587504343016, -57.45864774162057387, -21.12541641655958813 ) ) ;
#26756=VERTEX_POINT ( 'NONE', #28011 ) ;
#26758=CARTESIAN_POINT ( 'NONE',  ( 29.27175831897154978, -74.33129955521587817, -26.10413971565343516 ) ) ;
#26759=CARTESIAN_POINT ( 'NONE',  ( 7.472969336320000266, -74.00000023179998720, -38.65569830309999588 ) ) ;
#26760=ORIENTED_EDGE ( 'NONE', *, *, #7325, .F. ) ;
#26763=ADVANCED_FACE ( 'NONE', ( #16939 ), #4573, .T. ) ;
#26766=CIRCLE ( 'NONE', #1639, 39.25000000000000000 ) ;
#26767=CARTESIAN_POINT ( 'NONE',  ( 20.05203108810000145, -19.46163090469999801, 9.717827753279999925 ) ) ;
#26771=CARTESIAN_POINT ( 'NONE',  ( 9.136684621949999752, -66.46876714790001017, -24.36621523620000218 ) ) ;
#26773=ORIENTED_EDGE ( 'NONE', *, *, #23398, .F. ) ;
#26775=CARTESIAN_POINT ( 'NONE',  ( -15.42363691649999957, -67.46051717960000360, 22.84488648889999851 ) ) ;
#26778=CARTESIAN_POINT ( 'NONE',  ( 20.73262506157600882, -19.47322495657922303, 9.499032454948467930 ) ) ;
#26779=CARTESIAN_POINT ( 'NONE',  ( 23.53321159739309820, -64.04625792510528015, -7.550089874302127413 ) ) ;
#26783=ADVANCED_FACE ( 'NONE', ( #26253 ), #1926, .F. ) ;
#26785=CARTESIAN_POINT ( 'NONE',  ( -10.72105426646302817, -19.49371706970953610, -21.56716125212794566 ) ) ;
#26786=CARTESIAN_POINT ( 'NONE',  ( 25.32712259480000228, -57.40875702469999453, 1.379782074460000230 ) ) ;
#26790=CARTESIAN_POINT ( 'NONE',  ( -22.48840494017567693, -69.02525063278224593, 14.85218333891801734 ) ) ;
#26794=VERTEX_POINT ( 'NONE', #19677 ) ;
#26795=LINE ( 'NONE', #22262, #20128 ) ;
#26798=DIRECTION ( 'NONE',  ( 0.000000000000000000, 1.000000000000000000, 0.000000000000000000 ) ) ;
#26799=DIRECTION ( 'NONE',  ( 0.000000000000000000, 1.000000000000000000, 0.000000000000000000 ) ) ;
#26800=ORIENTED_EDGE ( 'NONE', *, *, #10822, .T. ) ;
#26803=CARTESIAN_POINT ( 'NONE',  ( 7.105427357599999217E-15, -74.50000000000000000, 3.552713678799999608E-15 ) ) ;
#26804=CARTESIAN_POINT ( 'NONE',  ( -21.90514033510000047, -74.14434415679998835, -32.45847700809999736 ) ) ;
#26808=CARTESIAN_POINT ( 'NONE',  ( -18.74560011510000024, -18.62107711730000048, 14.23481631049999940 ) ) ;
#26810=CARTESIAN_POINT ( 'NONE',  ( -7.325370793560000315, -18.50000000000000000, -24.94672208400000102 ) ) ;
#26811=CARTESIAN_POINT ( 'NONE',  ( 9.393614001710000494, -38.00000000000000000, -22.97877290430000130 ) ) ;
#26813=CARTESIAN_POINT ( 'NONE',  ( -7.325370793560000315, -45.73899999920000425, -24.94672208400000102 ) ) ;
#26818=CARTESIAN_POINT ( 'NONE',  ( -11.49099193059999813, -57.47122622279999860, -20.56185111770000162 ) ) ;
#26819=EDGE_CURVE ( 'NONE', #23453, #15463, #1636, .T. ) ;
#26822=CARTESIAN_POINT ( 'NONE',  ( 24.58030493329999899, -18.50000000000000000, 2.442848308399999890 ) ) ;
#26824=CARTESIAN_POINT ( 'NONE',  ( 22.70347112454390626, -37.13515264715037034, 10.14607557079202138 ) ) ;
#26827=ORIENTED_EDGE ( 'NONE', *, *, #27466, .T. ) ;
#26829=EDGE_CURVE ( 'NONE', #3916, #9687, #13057, .T. ) ;
#26831=B_SPLINE_CURVE_WITH_KNOTS ( 'NONE', 3,
 ( #28382, #8412, #21829, #28110, #28527, #17033, #16901, #8147, #25791, #17319, #26213, #14701, #6239, #23593, #24016, #19779, #8692 ),
 .UNSPECIFIED., .F., .F.,
 ( 4, 2, 2, 1, 1, 1, 1, 1, 2, 2, 4 ),
 ( 0.000000000000000000, 0.2500000000002183254, 0.3750000000003250733, 0.4375000000003810285, 0.4687500000004065637, 0.4843750000004191092, 0.4921875000004253820, 0.4960937500004258260, 0.4980468750004235501, 0.5000000000004213296, 1.000000000000000000 ),
 .UNSPECIFIED. ) ;
#26832=CARTESIAN_POINT ( 'NONE',  ( 0.000000000000000000, -18.50000000000000000, 0.000000000000000000 ) ) ;
#26834=CARTESIAN_POINT ( 'NONE',  ( -10.34918404329999930, -18.86473257140000115, -21.20072926229999766 ) ) ;
#26840=ORIENTED_EDGE ( 'NONE', *, *, #10555, .T. ) ;
#26841=DIRECTION ( 'NONE',  ( 0.000000000000000000, -1.000000000000000000, 0.000000000000000000 ) ) ;
#26844=VERTEX_POINT ( 'NONE', #18084 ) ;
#26848=CARTESIAN_POINT ( 'NONE',  ( -19.63525383122224710, -57.47122601392510433, 13.01113855736701197 ) ) ;
#26849=CARTESIAN_POINT ( 'NONE',  ( -11.46712328369999945, -34.67035637050000219, -19.43657039250000196 ) ) ;
#26850=CARTESIAN_POINT ( 'NONE',  ( -26.69328098980000163, -77.00000000000000000, -35.88566914520000495 ) ) ;
#26852=EDGE_LOOP ( 'NONE', ( #7910, #22882, #19081, #5495, #21539 ) ) ;
#26856=CARTESIAN_POINT ( 'NONE',  ( 7.318372426699999878, -73.93831497249999529, 38.68350751799999898 ) ) ;
#26857=CARTESIAN_POINT ( 'NONE',  ( 0.000000000000000000, -80.50000000000000000, 0.000000000000000000 ) ) ;
#26859=B_SPLINE_SURFACE_WITH_KNOTS ( 'NONE', 5, 5, ( 
 ( #11951, #23054, #11654, #3236, #20863, #18677 ),
 ( #12093, #923, #27577, #2800, #9623, #2947 ),
 ( #3369, #16479, #25381, #12234, #7749, #1069 ),
 ( #16177, #9908, #16615, #25509, #25088, #14003 ),
 ( #5547, #23323, #21147, #22910, #10037, #18951 ),
 ( #22759, #11810, #20722, #781, #21834, #19090 ) ),
 .UNSPECIFIED., .F., .F., .F.,
 ( 6, 6 ),
 ( 6, 6 ),
 ( 2.659855565630000029, 4.432291325320000475 ),
 ( 0.000000000000000000, 0.5000000000000000000 ),
 .UNSPECIFIED. ) ;
#26860=CARTESIAN_POINT ( 'NONE',  ( 22.12248824515891243, -19.46487770188272393, 0.1046948809405091052 ) ) ;
#26862=EDGE_LOOP ( 'NONE', ( #10450, #20565, #23129, #28072 ) ) ;
#26863=CARTESIAN_POINT ( 'NONE',  ( 26.97099430927276487, -72.31255207680982267, -11.30091564182526653 ) ) ;
#26864=CARTESIAN_POINT ( 'NONE',  ( -21.14183719079999690, -62.95300605010000083, 15.28077941859999989 ) ) ;
#26865=CARTESIAN_POINT ( 'NONE',  ( 8.245988246530000509, -37.92543680059999645, -21.67015450270000088 ) ) ;
#26866=CARTESIAN_POINT ( 'NONE',  ( 8.492728600515889070, -19.47622732623166542, -20.12650533279332876 ) ) ;
#26867=CARTESIAN_POINT ( 'NONE',  ( -9.506169627659998511, -74.00000000000000000, 42.57810630240000194 ) ) ;
#26868=CARTESIAN_POINT ( 'NONE',  ( 23.53496214160000122, -18.86473257140000115, 1.637708341159999970 ) ) ;
#26871=ORIENTED_EDGE ( 'NONE', *, *, #26923, .T. ) ;
#26872=DIRECTION ( 'NONE',  ( 0.000000000000000000, -1.000000000000000000, 0.000000000000000000 ) ) ;
#26873=CARTESIAN_POINT ( 'NONE',  ( 28.00537423697155148, -69.05891618901559070, 2.237991812796679802 ) ) ;
#26877=CARTESIAN_POINT ( 'NONE',  ( 21.89902306919999830, -37.95659433950000050, -8.637924301090000867 ) ) ;
#26880=LINE ( 'NONE', #8785, #1613 ) ;
#26885=CARTESIAN_POINT ( 'NONE',  ( -13.94341442410000020, -60.21477618889999661, 21.38633822419999930 ) ) ;
#26887=CIRCLE ( 'NONE', #25018, 6.750000000000000000 ) ;
#26888=EDGE_LOOP ( 'NONE', ( #22156, #21155, #23978, #27309 ) ) ;
#26889=CARTESIAN_POINT ( 'NONE',  ( -12.45758713059999856, -65.72077506549999271, 22.18618133640000067 ) ) ;
#26890=CARTESIAN_POINT ( 'NONE',  ( -11.74919631470000070, -57.47570992170000181, 20.26880469069999791 ) ) ;
#26896=DIRECTION ( 'NONE',  ( 0.000000000000000000, -1.000000000000000000, 0.000000000000000000 ) ) ;
#26898=ORIENTED_EDGE ( 'NONE', *, *, #27903, .F. ) ;
#26900=CARTESIAN_POINT ( 'NONE',  ( 21.48302419030000010, -36.56890884650000118, -7.253824583220000122 ) ) ;
#26902=ORIENTED_EDGE ( 'NONE', *, *, #11843, .T. ) ;
#26905=CARTESIAN_POINT ( 'NONE',  ( 20.69873715099999956, -52.63055504179948230, 10.61298605969999187 ) ) ;
#26907=CARTESIAN_POINT ( 'NONE',  ( 21.54650012300000128, -26.06274386009999944, 9.572267663609999033 ) ) ;
#26911=CARTESIAN_POINT ( 'NONE',  ( 19.22218838680000275, -18.50000000000000000, 9.014732214529999510 ) ) ;
#26912=CARTESIAN_POINT ( 'NONE',  ( -32.72868145578198096, -79.93462708495536617, -22.47659135972876143 ) ) ;
#26918=CARTESIAN_POINT ( 'NONE',  ( 21.67805398002857586, -19.48685756505367905, 9.537775450224595275 ) ) ;
#26919=CARTESIAN_POINT ( 'NONE',  ( -39.92825895920000079, -74.14144493790000467, -7.283540598980000169 ) ) ;
#26923=EDGE_CURVE ( 'NONE', #6001, #13803, #21929, .T. ) ;
#26928=ORIENTED_EDGE ( 'NONE', *, *, #13993, .T. ) ;
#26929=VECTOR ( 'NONE', #5380, 1000.000000000000000 ) ;
#26930=AXIS2_PLACEMENT_3D ( 'NONE', #21661, #21376, #12609 ) ;
#26934=CARTESIAN_POINT ( 'NONE',  ( 46.25000000000000000, -74.00000000000000000, -4.582575694960000057 ) ) ;
#26935=ORIENTED_EDGE ( 'NONE', *, *, #10151, .F. ) ;
#26937=CARTESIAN_POINT ( 'NONE',  ( -22.43272078519999724, -80.34292036729999609, -32.20769377289999369 ) ) ;
#26945=DIRECTION ( 'NONE',  ( 1.000000000000000000, 0.000000000000000000, 0.000000000000000000 ) ) ;
#26946=CARTESIAN_POINT ( 'NONE',  ( -21.71458329359999695, -74.50000000000000000, -32.69645379630000548 ) ) ;
#26947=EDGE_CURVE ( 'NONE', #8106, #134, #6467, .T. ) ;
#26955=AXIS2_PLACEMENT_3D ( 'NONE', #27206, #11438, #27348 ) ;
#26957=VECTOR ( 'NONE', #28237, 1000.000000000000000 ) ;
#26960=CARTESIAN_POINT ( 'NONE',  ( 8.963945925320000896, -35.29521789780000063, -19.99082963590000261 ) ) ;
#26963=CARTESIAN_POINT ( 'NONE',  ( 46.42255779199999921, -80.25272389239999882, -3.562991745209999728 ) ) ;
#26966=CARTESIAN_POINT ( 'NONE',  ( -12.22420097160000019, -62.12717499380000419, -20.63207585329999816 ) ) ;
#26968=ORIENTED_EDGE ( 'NONE', *, *, #10325, .T. ) ;
#26974=ORIENTED_EDGE ( 'NONE', *, *, #18810, .F. ) ;
#26976=AXIS2_PLACEMENT_3D ( 'NONE', #6154, #12837, #21749 ) ;
#26977=CARTESIAN_POINT ( 'NONE',  ( 1.678657213230000024E-14, -74.00000000000000000, 7.838174553849999450E-15 ) ) ;
#26983=CARTESIAN_POINT ( 'NONE',  ( -17.94180966909999597, -45.73899999920000425, 18.81731824139999887 ) ) ;
#26984=CARTESIAN_POINT ( 'NONE',  ( -20.04435942636430923, -59.05300800389983351, 12.20496567544505062 ) ) ;
#26989=CARTESIAN_POINT ( 'NONE',  ( -22.58183123469999742, -70.96441436690000160, 17.76382364619999876 ) ) ;
#26991=ADVANCED_FACE ( 'NONE', ( #8014 ), #23771, .F. ) ;
#26994=CARTESIAN_POINT ( 'NONE',  ( 26.07303258718441086, -74.32832717789354149, -29.29802673409578517 ) ) ;
#26995=CARTESIAN_POINT ( 'NONE',  ( 20.56993010089999885, -36.00000000000000000, -10.19436680729999978 ) ) ;
#26999=VECTOR ( 'NONE', #25531, 1000.000000000000000 ) ;
#27002=VERTEX_POINT ( 'NONE', #5548 ) ;
#27003=B_SPLINE_CURVE_WITH_KNOTS ( 'NONE', 5,
 ( #15181, #8640, #6173, #15048, #6025, #19579, #3855, #26436, #10813 ),
 .UNSPECIFIED., .F., .F.,
 ( 6, 3, 6 ),
 ( 0.000000000000000000, 1.377214429579999955, 2.292501860869999852 ),
 .UNSPECIFIED. ) ;
#27006=CARTESIAN_POINT ( 'NONE',  ( 7.260248548399999891, -73.97917265380000629, 40.03821526680000176 ) ) ;
#27008=CARTESIAN_POINT ( 'NONE',  ( 23.40535227632090098, -19.48298526462809122, 1.394588373438266693 ) ) ;
#27009=CARTESIAN_POINT ( 'NONE',  ( 27.11562635247914699, -72.17813883581031575, -11.54692017584613772 ) ) ;
#27011=CARTESIAN_POINT ( 'NONE',  ( 9.227003638719999401, -35.93081093159999995, -19.61343128729999918 ) ) ;
#27013=CARTESIAN_POINT ( 'NONE',  ( 8.617475452619551390, -19.47931211704219479, -19.97879563106347334 ) ) ;
#27014=ORIENTED_EDGE ( 'NONE', *, *, #8897, .F. ) ;
#27019=CARTESIAN_POINT ( 'NONE',  ( -2.150719047535482709, -19.47341637985288187, -22.71689757131826326 ) ) ;
#27021=CARTESIAN_POINT ( 'NONE',  ( 28.23243646506086790, -69.78284652344737538, 2.418637941536898150 ) ) ;
#27025=CARTESIAN_POINT ( 'NONE',  ( -13.17062163620000170, -68.28989939179999169, -23.12788393509999807 ) ) ;
#27029=CARTESIAN_POINT ( 'NONE',  ( -10.13149966729999818, -18.50000000000000000, 18.43352823549999897 ) ) ;
#27032=CARTESIAN_POINT ( 'NONE',  ( 36.48289528369999601, -74.76922865969999066, -14.76362601449999801 ) ) ;
#27037=DIRECTION ( 'NONE',  ( 1.000000000000000000, 0.000000000000000000, 0.000000000000000000 ) ) ;
#27038=LINE ( 'NONE', #2567, #601 ) ;
#27039=DIRECTION ( 'NONE',  ( 1.000000000000000000, 0.000000000000000000, 0.000000000000000000 ) ) ;
#27040=CARTESIAN_POINT ( 'NONE',  ( 21.83114860719999939, -37.33500412619999764, -8.564557754590000016 ) ) ;
#27042=ORIENTED_EDGE ( 'NONE', *, *, #9583, .F. ) ;
#27043=CARTESIAN_POINT ( 'NONE',  ( -7.250123090889999844, -74.26791556519999915, -40.35962647450000418 ) ) ;
#27044=CARTESIAN_POINT ( 'NONE',  ( 29.28732071508218837, -74.32953776423283898, -26.08572060009336724 ) ) ;
#27046=VERTEX_POINT ( 'NONE', #540 ) ;
#27048=DIRECTION ( 'NONE',  ( 0.9295286103719511139, 0.000000000000000000, 0.3687499999999862554 ) ) ;
#27055=EDGE_CURVE ( 'NONE', #22777, #11422, #205, .T. ) ;
#27056=CIRCLE ( 'NONE', #18214, 21.03431122519999974 ) ;
#27057=CARTESIAN_POINT ( 'NONE',  ( 19.56503591259999908, -19.46390881170000142, 10.14212564559999841 ) ) ;
#27058=CARTESIAN_POINT ( 'NONE',  ( -22.00722825609999944, -67.14423135289999323, 14.02040059770000191 ) ) ;
#27060=ORIENTED_EDGE ( 'NONE', *, *, #24082, .T. ) ;
#27061=CARTESIAN_POINT ( 'NONE',  ( -12.04566629249999998, -72.37490051890000586, -26.07979331039999948 ) ) ;
#27063=CARTESIAN_POINT ( 'NONE',  ( 21.59803991680463042, -19.48549492419365237, 9.516754966957947204 ) ) ;
#27065=ORIENTED_EDGE ( 'NONE', *, *, #8540, .F. ) ;
#27066=ADVANCED_FACE ( 'NONE', ( #7220 ), #12666, .T. ) ;
#27067=CARTESIAN_POINT ( 'NONE',  ( 36.25000000000000000, -84.50000000000000000, 2.314797894279999601E-15 ) ) ;
#27068=ORIENTED_EDGE ( 'NONE', *, *, #21796, .F. ) ;
#27070=DIRECTION ( 'NONE',  ( 0.000000000000000000, 1.000000000000000000, 0.000000000000000000 ) ) ;
#27071=DIRECTION ( 'NONE',  ( 1.000000000000000000, 0.000000000000000000, -6.106226635439993914E-16 ) ) ;
#27075=ORIENTED_EDGE ( 'NONE', *, *, #12273, .F. ) ;
#27076=ORIENTED_EDGE ( 'NONE', *, *, #22012, .F. ) ;
#27077=CARTESIAN_POINT ( 'NONE',  ( -22.77778991426668043, -70.31271151318118484, 15.47469272077778335 ) ) ;
#27079=CARTESIAN_POINT ( 'NONE',  ( 47.06797221370000273, -74.41279298919998553, -1.870483754820000177 ) ) ;
#27083=CARTESIAN_POINT ( 'NONE',  ( 8.607506958290001009, -36.72040101139999990, -21.55953475569999966 ) ) ;
#27086=ORIENTED_EDGE ( 'NONE', *, *, #6468, .T. ) ;
#27088=CARTESIAN_POINT ( 'NONE',  ( 36.29003938660000017, -73.99962328729999683, -14.01560472500000110 ) ) ;
#27091=CARTESIAN_POINT ( 'NONE',  ( -40.70731707320000226, -74.50000000000000000, 7.215414233289999757 ) ) ;
#27092=CARTESIAN_POINT ( 'NONE',  ( -21.82150020430000126, -74.12815218200000800, -32.45709266180000441 ) ) ;
#27096=ADVANCED_FACE ( 'NONE', ( #17340 ), #17727, .F. ) ;
#27100=DIRECTION ( 'NONE',  ( -1.000000000000000000, 0.000000000000000000, 0.000000000000000000 ) ) ;
#27103=DIRECTION ( 'NONE',  ( 0.9704142011833033488, 0.000000000000000000, 0.2414462220490755373 ) ) ;
#27106=CARTESIAN_POINT ( 'NONE',  ( -11.35954001540000036, -74.00000000000000000, 47.25000000000000000 ) ) ;
#27108=CARTESIAN_POINT ( 'NONE',  ( 46.66864852690000021, -79.99872154319999140, -3.727018626880000074 ) ) ;
#27110=CARTESIAN_POINT ( 'NONE',  ( -11.35747017449999952, -60.48499519860000362, -21.31231279229999842 ) ) ;
#27111=CARTESIAN_POINT ( 'NONE',  ( 24.57984581210000030, -66.63210100880000653, -8.034882954890001372 ) ) ;
#27112=CARTESIAN_POINT ( 'NONE',  ( 10.20110288159999890, -84.50000000000000000, 41.00000000000000000 ) ) ;
#27114=B_SPLINE_CURVE_WITH_KNOTS ( 'NONE', 5,
 ( #24104, #13013, #21924, #28747, #1975, #10819, #8648, #17550, #18284 ),
 .UNSPECIFIED., .F., .F.,
 ( 6, 3, 6 ),
 ( 43.40831274110000493, 61.94013117540000479, 64.87293781380000723 ),
 .UNSPECIFIED. ) ;
#27115=VECTOR ( 'NONE', #25581, 1000.000000000000000 ) ;
#27116=EDGE_CURVE ( 'NONE', #23532, #1349, #17266, .T. ) ;
#27117=VERTEX_POINT ( 'NONE', #23380 ) ;
#27118=CARTESIAN_POINT ( 'NONE',  ( -13.49470513559999851, -57.43018267549999933, 20.74700234780000230 ) ) ;
#27119=CARTESIAN_POINT ( 'NONE',  ( -21.74262969930000011, -74.09723562380000317, -32.46276855370000192 ) ) ;
#27120=ORIENTED_EDGE ( 'NONE', *, *, #364, .T. ) ;
#27121=TOROIDAL_SURFACE ( 'NONE', #23390, 21.03431122519999974, 1.000000000000000000 ) ;
#27122=DIRECTION ( 'NONE',  ( 1.000000000000000000, 0.000000000000000000, 0.000000000000000000 ) ) ;
#27126=CARTESIAN_POINT ( 'NONE',  ( 24.48314189319999912, -69.76823842119999597, 12.05682714019999935 ) ) ;
#27127=ORIENTED_EDGE ( 'NONE', *, *, #21252, .F. ) ;
#27129=EDGE_CURVE ( 'NONE', #22982, #16224, #10260, .T. ) ;
#27131=CARTESIAN_POINT ( 'NONE',  ( 37.29611236860000645, -80.00000000000000000, -13.75000000000000000 ) ) ;
#27132=CARTESIAN_POINT ( 'NONE',  ( 40.27753662827743142, -74.17170883776950063, 7.244686332501536263 ) ) ;
#27133=ORIENTED_EDGE ( 'NONE', *, *, #12765, .F. ) ;
#27136=EDGE_LOOP ( 'NONE', ( #2903, #11860, #20888, #21880 ) ) ;
#27140=CARTESIAN_POINT ( 'NONE',  ( -19.46796618480000163, -32.68478243029999675, 14.19297777630000112 ) ) ;
#27141=CARTESIAN_POINT ( 'NONE',  ( -3.562216332169999777, -80.49999996399999702, 46.31451619710000500 ) ) ;
#27142=CARTESIAN_POINT ( 'NONE',  ( -2.053743188970000031E-15, -82.25000000000000000, 47.25000000000000000 ) ) ;
#27143=CARTESIAN_POINT ( 'NONE',  ( 23.43108223770000009, -60.27873802119999880, -9.526351984520001537 ) ) ;
#27145=CARTESIAN_POINT ( 'NONE',  ( -12.06159284909973906, -57.47122623868258984, 20.23241278189946257 ) ) ;
#27146=VERTEX_POINT ( 'NONE', #16383 ) ;
#27147=EDGE_CURVE ( 'NONE', #321, #22026, #3287, .T. ) ;
#27149=CARTESIAN_POINT ( 'NONE',  ( -1.314504061159999897E-13, -19.46510050329999686, -1.119104808819999722E-13 ) ) ;
#27150=AXIS2_PLACEMENT_3D ( 'NONE', #23482, #3248, #19237 ) ;
#27153=CARTESIAN_POINT ( 'NONE',  ( 7.250123090889999844, -74.26791556519999915, 40.35962647450000418 ) ) ;
#27157=CARTESIAN_POINT ( 'NONE',  ( -20.56018235820000228, -57.40875686090000585, 14.85415984670000000 ) ) ;
#27158=CARTESIAN_POINT ( 'NONE',  ( 8.476165110749999343, -37.64222909819999785, -21.78580730850000080 ) ) ;
#27159=EDGE_CURVE ( 'NONE', #12707, #13695, #21196, .T. ) ;
#27160=AXIS2_PLACEMENT_3D ( 'NONE', #1601, #1878, #14556 ) ;
#27164=CARTESIAN_POINT ( 'NONE',  ( 9.356041104380000917, -84.00000000000000000, -37.60355029590000697 ) ) ;
#27166=CARTESIAN_POINT ( 'NONE',  ( -2.554621587543492556, -19.48534489990609231, -23.45393302294781535 ) ) ;
#27169=CARTESIAN_POINT ( 'NONE',  ( 40.70731707320000226, -82.25000000000000000, 7.215414233289999757 ) ) ;
#27172=CARTESIAN_POINT ( 'NONE',  ( 22.33592606139999859, -44.89607405940000007, -8.998660423470001390 ) ) ;
#27174=DIRECTION ( 'NONE',  ( -0.3438555744121192803, 0.06995790998172438102, 0.9364129616663261491 ) ) ;
#27177=CARTESIAN_POINT ( 'NONE',  ( -32.67527180710000323, -74.50000000430000568, -22.00249031559999935 ) ) ;
#27178=CARTESIAN_POINT ( 'NONE',  ( -22.45768892722265164, -79.92187437579165987, -32.73741433150124180 ) ) ;
#27180=CARTESIAN_POINT ( 'NONE',  ( -15.42363573210000105, -67.46051717960000360, 22.84488635619999997 ) ) ;
#27181=CARTESIAN_POINT ( 'NONE',  ( 20.01429421219999938, -35.44265673480000345, -8.963580811669999093 ) ) ;
#27184=CARTESIAN_POINT ( 'NONE',  ( 21.13310776459999829, -36.23917065820000261, -8.855030636489999551 ) ) ;
#27186=CARTESIAN_POINT ( 'NONE',  ( -40.70731707320000226, -74.50000000000000000, 7.215414233289999757 ) ) ;
#27193=ORIENTED_EDGE ( 'NONE', *, *, #14536, .T. ) ;
#27194=EDGE_CURVE ( 'NONE', #27454, #6381, #9019, .T. ) ;
#27195=CARTESIAN_POINT ( 'NONE',  ( 20.34628061889999984, -52.63293862049999916, 11.13082833170000008 ) ) ;
#27200=DIRECTION ( 'NONE',  ( 0.000000000000000000, 1.000000000000000000, 0.000000000000000000 ) ) ;
#27201=CARTESIAN_POINT ( 'NONE',  ( 18.78522494180000280, -18.50000000000000000, 9.483810324729999408 ) ) ;
#27206=CARTESIAN_POINT ( 'NONE',  ( -26.69328098980000163, -74.50000000000000000, -35.88566914520000495 ) ) ;
#27207=CARTESIAN_POINT ( 'NONE',  ( 9.014750546150001043, -22.53353178400000445, -19.04514867530000188 ) ) ;
#27212=VECTOR ( 'NONE', #6907, 1000.000000000000000 ) ;
#27221=AXIS2_PLACEMENT_3D ( 'NONE', #23936, #8330, #25711 ) ;
#27223=DIRECTION ( 'NONE',  ( 0.000000000000000000, 1.000000000000000000, 0.000000000000000000 ) ) ;
#27224=CARTESIAN_POINT ( 'NONE',  ( 10.18473603500000024, -36.00000000000000000, -20.58226785680000148 ) ) ;
#27225=VERTEX_POINT ( 'NONE', #19941 ) ;
#27226=CARTESIAN_POINT ( 'NONE',  ( 7.248098695798295132, -73.87273571702228026, -39.83391879123477963 ) ) ;
#27228=EDGE_CURVE ( 'NONE', #20825, #19738, #10711, .T. ) ;
#27229=VERTEX_POINT ( 'NONE', #2337 ) ;
#27232=CARTESIAN_POINT ( 'NONE',  ( 9.038647564319999717, -35.72724395809999720, -19.55068592700000352 ) ) ;
#27236=CARTESIAN_POINT ( 'NONE',  ( -2.783420023329999715, -64.17227325300000018, -26.33714589019999863 ) ) ;
#27237=CARTESIAN_POINT ( 'NONE',  ( -21.99985828019999801, -74.00000000000000000, -31.89935321680000158 ) ) ;
#27238=ORIENTED_EDGE ( 'NONE', *, *, #1529, .F. ) ;
#27239=CARTESIAN_POINT ( 'NONE',  ( -0.5372032561875097478, -32.73217874168935992, -22.49059537401083375 ) ) ;
#27241=CARTESIAN_POINT ( 'NONE',  ( 36.74280283558181992, -74.40473351797265877, -14.55378675820746892 ) ) ;
#27243=DIRECTION ( 'NONE',  ( 0.000000000000000000, 1.000000000000000000, 0.000000000000000000 ) ) ;
#27245=CARTESIAN_POINT ( 'NONE',  ( 23.42373825549999822, -62.44588796569999545, 10.52566358100000166 ) ) ;
#27246=CARTESIAN_POINT ( 'NONE',  ( 8.427784894169999319, -35.19242348989999414, -20.91698756690000138 ) ) ;
#27250=FACE_OUTER_BOUND ( 'NONE', #22170, .T. ) ;
#27251=CARTESIAN_POINT ( 'NONE',  ( -11.37864349189999835, -18.61797544070000043, 18.64968536590000170 ) ) ;
#27252=CARTESIAN_POINT ( 'NONE',  ( -11.54937042210000087, -60.21420103860000239, -22.76847067690000159 ) ) ;
#27254=DIRECTION ( 'NONE',  ( -0.9387128607161810967, 0.000000000000000000, -0.3447001089730664103 ) ) ;
#27255=CARTESIAN_POINT ( 'NONE',  ( 26.41739731730000074, -71.28695100890000447, -9.226526782039998764 ) ) ;
#27259=CARTESIAN_POINT ( 'NONE',  ( -14.81112187414681003, -74.50000000000001421, 36.34845292753433199 ) ) ;
#27265=CARTESIAN_POINT ( 'NONE',  ( -2.578307999469999778, -52.56313962710000709, -25.11373953509999879 ) ) ;
#27266=ADVANCED_FACE ( 'NONE', ( #13242 ), #4509, .T. ) ;
#27268=CARTESIAN_POINT ( 'NONE',  ( -11.41594931139999858, -19.46510050329999686, -18.84569254350000023 ) ) ;
#27269=CARTESIAN_POINT ( 'NONE',  ( -16.78865735879999832, -72.00000000000000000, 25.46808810279999946 ) ) ;
#27270=CARTESIAN_POINT ( 'NONE',  ( -10.05111287380000107, -18.50000000000000000, -21.88335580340000064 ) ) ;
#27271=CARTESIAN_POINT ( 'NONE',  ( 9.708867067583597077, -61.04180997458320945, -23.92438532451274114 ) ) ;
#27272=EDGE_LOOP ( 'NONE', ( #10748, #3215, #26478, #4220 ) ) ;
#27273=DIRECTION ( 'NONE',  ( 1.000000000000000000, 0.000000000000000000, 0.000000000000000000 ) ) ;
#27275=DIRECTION ( 'NONE',  ( -1.000000000000000000, 0.000000000000000000, 0.000000000000000000 ) ) ;
#27276=ORIENTED_EDGE ( 'NONE', *, *, #22557, .F. ) ;
#27277=B_SPLINE_CURVE_WITH_KNOTS ( 'NONE', 3,
 ( #4221, #7156, #6713, #13095, #6562, #15876 ),
 .UNSPECIFIED., .F., .F.,
 ( 4, 2, 4 ),
 ( 0.000000000000000000, 0.5000000000000000000, 1.000000000000000000 ),
 .UNSPECIFIED. ) ;
#27278=VECTOR ( 'NONE', #21601, 1000.000000000000000 ) ;
#27279=CARTESIAN_POINT ( 'NONE',  ( 20.62325427951632051, -19.20927481666025827, -7.731222864529065930 ) ) ;
#27284=EDGE_CURVE ( 'NONE', #12242, #8854, #4657, .T. ) ;
#27292=VERTEX_POINT ( 'NONE', #7002 ) ;
#27293=ADVANCED_FACE ( 'NONE', ( #22002, #17779 ), #24330, .F. ) ;
#27294=CARTESIAN_POINT ( 'NONE',  ( -19.59431174800317521, -18.62337006874626155, 14.76282611549721402 ) ) ;
#27295=CARTESIAN_POINT ( 'NONE',  ( 20.45177504849999650, -36.01773751660000045, -9.130641075480001589 ) ) ;
#27297=VERTEX_POINT ( 'NONE', #24776 ) ;
#27299=DIRECTION ( 'NONE',  ( 0.7071067811865492381, 0.000000000000000000, -0.7071067811865457964 ) ) ;
#27302=CARTESIAN_POINT ( 'NONE',  ( -20.88544710529999904, -61.59957509759999539, 15.07454172879999987 ) ) ;
#27303=CARTESIAN_POINT ( 'NONE',  ( 7.999160519940001102, -37.31099427210000385, -21.56623231000000374 ) ) ;
#27304=CARTESIAN_POINT ( 'NONE',  ( 8.783950479490158614, -19.48412239595453599, -19.74263315380339989 ) ) ;
#27305=EDGE_LOOP ( 'NONE', ( #6309, #22075, #23192, #4679 ) ) ;
#27306=CARTESIAN_POINT ( 'NONE',  ( -39.84323359140208254, -73.87844996482343163, 7.248307137522745691 ) ) ;
#27307=CARTESIAN_POINT ( 'NONE',  ( 24.46521773039999914, -18.62337009750000050, 1.825159675170000106 ) ) ;
#27308=CARTESIAN_POINT ( 'NONE',  ( 21.47791241899999903, -36.56811125080000835, -7.356933755090000027 ) ) ;
#27309=ORIENTED_EDGE ( 'NONE', *, *, #7227, .F. ) ;
#27310=CARTESIAN_POINT ( 'NONE',  ( -2.605118868831385104, -19.48886652629414229, -23.65890925434035452 ) ) ;
#27311=B_SPLINE_CURVE_WITH_KNOTS ( 'NONE', 3,
 ( #6788, #13917, #11566, #25151, #13768, #20637, #2713, #20182, #24552, #20478, #13318 ),
 .UNSPECIFIED., .F., .F.,
 ( 4, 1, 1, 1, 2, 2, 4 ),
 ( 0.000000000000000000, 0.2499999999999971689, 0.3749999999999957812, 0.4374999999999950595, 0.4687499999999949485, 0.4999999999999948930, 1.000000000000000000 ),
 .UNSPECIFIED. ) ;
#27313=CARTESIAN_POINT ( 'NONE',  ( -2.363861431289999704, -52.59522851920000619, -24.20187825489999867 ) ) ;
#27316=ADVANCED_FACE ( 'NONE', ( #6397 ), #2049, .T. ) ;
#27318=CARTESIAN_POINT ( 'NONE',  ( 22.87094945020000125, -44.87455296059999910, -9.357772773720000714 ) ) ;
#27321=VERTEX_POINT ( 'NONE', #4216 ) ;
#27325=CARTESIAN_POINT ( 'NONE',  ( -12.08078259732632631, -68.11638242249664188, -25.01700482484572774 ) ) ;
#27326=CARTESIAN_POINT ( 'NONE',  ( 9.018303738449999329, -35.73233772869999569, -20.14104784029999706 ) ) ;
#27327=CARTESIAN_POINT ( 'NONE',  ( 36.24656994149999889, -79.00000000000000000, -15.05817610060000078 ) ) ;
#27328=DIRECTION ( 'NONE',  ( 0.09756097560976705052, 0.000000000000000000, -0.9952295494196654602 ) ) ;
#27329=CARTESIAN_POINT ( 'NONE',  ( 20.16453947749999998, -36.00000000000000000, -9.644867042430000481 ) ) ;
#27332=EDGE_LOOP ( 'NONE', ( #17880, #15381, #1661 ) ) ;
#27333=CARTESIAN_POINT ( 'NONE',  ( -0.8216735279219999910, -65.07443093669999712, -25.13632616349999793 ) ) ;
#27338=CARTESIAN_POINT ( 'NONE',  ( -10.87473961043062509, -19.46454318506218328, 19.18358865193880192 ) ) ;
#27341=CARTESIAN_POINT ( 'NONE',  ( -7.250083186824390680, -73.98707088453728886, -40.01432744588630896 ) ) ;
#27342=CARTESIAN_POINT ( 'NONE',  ( -14.32651846709999965, -74.09825332389999630, 36.37998168949999922 ) ) ;
#27343=CARTESIAN_POINT ( 'NONE',  ( 9.687968342419999601, -71.22032982880000418, -26.22375966410000103 ) ) ;
#27346=ORIENTED_EDGE ( 'NONE', *, *, #27656, .T. ) ;
#27348=DIRECTION ( 'NONE',  ( 1.000000000000000000, 0.000000000000000000, 0.000000000000000000 ) ) ;
#27349=CARTESIAN_POINT ( 'NONE',  ( 8.512197389749998067, -28.54984126589999960, -20.54345199129999600 ) ) ;
#27351=CARTESIAN_POINT ( 'NONE',  ( 38.62788659690000515, -73.50000000000000000, -7.627568735119999666 ) ) ;
#27352=CARTESIAN_POINT ( 'NONE',  ( -38.62788781560000473, -74.00000025069999765, -7.627567457969999687 ) ) ;
#27355=TOROIDAL_SURFACE ( 'NONE', #14324, 0.5000000000000000000, 0.5000000000000000000 ) ;
#27360=AXIS2_PLACEMENT_3D ( 'NONE', #676, #25286, #27618 ) ;
#27361=DIRECTION ( 'NONE',  ( 1.000000000000000000, 0.000000000000000000, 0.000000000000000000 ) ) ;
#27363=ORIENTED_EDGE ( 'NONE', *, *, #18170, .T. ) ;
#27367=CARTESIAN_POINT ( 'NONE',  ( 10.86700788799999984, -36.00000000000000000, -21.35995475889999895 ) ) ;
#27368=ORIENTED_EDGE ( 'NONE', *, *, #14277, .T. ) ;
#27370=CARTESIAN_POINT ( 'NONE',  ( 22.86992907279976350, -57.41946977148945308, 10.24154027049986126 ) ) ;
#27372=CIRCLE ( 'NONE', #12880, 0.5000000000000004441 ) ;
#27376=CARTESIAN_POINT ( 'NONE',  ( -2.143662412449999888, -70.80052042910000409, -27.67943948509999785 ) ) ;
#27379=CARTESIAN_POINT ( 'NONE',  ( 36.54166093210000810, -74.19847614699999383, -14.46229251740000166 ) ) ;
#27381=CARTESIAN_POINT ( 'NONE',  ( 24.13573937880000031, -60.48499519869999830, 0.8202987023390000410 ) ) ;
#27382=CARTESIAN_POINT ( 'NONE',  ( 36.32677412860000032, -74.12275851199999011, -14.57143996970000011 ) ) ;
#27384=CIRCLE ( 'NONE', #7376, 3.750000000000000000 ) ;
#27385=CARTESIAN_POINT ( 'NONE',  ( -19.41486357870000035, -39.36577621589999865, 11.81755283919999933 ) ) ;
#27389=ADVANCED_FACE ( 'NONE', ( #2929 ), #14135, .F. ) ;
#27391=CARTESIAN_POINT ( 'NONE',  ( 21.64198627210000225, -62.93490527480000196, 11.11445933409999931 ) ) ;
#27392=CARTESIAN_POINT ( 'NONE',  ( 8.965966767370000312, -34.65022614779999799, -19.90557425269999925 ) ) ;
#27396=CARTESIAN_POINT ( 'NONE',  ( 45.84677419350000349, -80.50000000000000000, -4.286925650119999709 ) ) ;
#27400=CIRCLE ( 'NONE', #13906, 23.36116116979999902 ) ;
#27401=CARTESIAN_POINT ( 'NONE',  ( 24.36633741079999993, -66.46905249630000867, -9.136733449319999423 ) ) ;
#27403=VERTEX_POINT ( 'NONE', #9607 ) ;
#27404=CARTESIAN_POINT ( 'NONE',  ( 47.12009151217586833, -74.36612146640514709, -1.373451506462775029 ) ) ;
#27405=ORIENTED_EDGE ( 'NONE', *, *, #20028, .T. ) ;
#27407=CARTESIAN_POINT ( 'NONE',  ( 22.16979245059999926, -53.80651132049999319, 10.07374405240000037 ) ) ;
#27409=ORIENTED_EDGE ( 'NONE', *, *, #28273, .F. ) ;
#27411=CARTESIAN_POINT ( 'NONE',  ( 39.89376886939999878, -74.19145175539999570, 7.305188534010000012 ) ) ;
#27412=CARTESIAN_POINT ( 'NONE',  ( -10.56814158951102556, -19.46927975582494952, -19.88243901464971941 ) ) ;
#27413=CARTESIAN_POINT ( 'NONE',  ( -10.20110288159999890, -74.00000000000000000, -41.00000000000000000 ) ) ;
#27416=TOROIDAL_SURFACE ( 'NONE', #8327, 1.500000000000000000, 0.5000000000000000000 ) ;
#27423=CIRCLE ( 'NONE', #15759, 10.00000000000000000 ) ;
#27427=ORIENTED_EDGE ( 'NONE', *, *, #10277, .T. ) ;
#27428=ADVANCED_FACE ( 'NONE', ( #18216 ), #5100, .T. ) ;
#27430=B_SPLINE_CURVE_WITH_KNOTS ( 'NONE', 5,
 ( #11579, #18310, #8216, #17108, #23811, #5889 ),
 .UNSPECIFIED., .F., .F.,
 ( 6, 6 ),
 ( 0.000000000000000000, 1.000000000000000000 ),
 .UNSPECIFIED. ) ;
#27431=ADVANCED_FACE ( 'NONE', ( #905 ), #28266, .T. ) ;
#27432=CARTESIAN_POINT ( 'NONE',  ( -19.12961493519999934, -39.34784663169999419, 13.40230581219999983 ) ) ;
#27438=VECTOR ( 'NONE', #1326, 1000.000000000000000 ) ;
#27439=CIRCLE ( 'NONE', #25584, 10.00000000000000000 ) ;
#27441=CIRCLE ( 'NONE', #24636, 6.750000000000000000 ) ;
#27442=CARTESIAN_POINT ( 'NONE',  ( -39.30828467247898317, -73.61493928634477868, -7.216929735102859844 ) ) ;
#27444=CARTESIAN_POINT ( 'NONE',  ( 19.99313163150000250, -36.00000036840000206, -9.451827061030000365 ) ) ;
#27449=CARTESIAN_POINT ( 'NONE',  ( -21.43329341219999762, -64.24504445130001784, 15.59675287610000005 ) ) ;
#27454=VERTEX_POINT ( 'NONE', #6807 ) ;
#27456=CARTESIAN_POINT ( 'NONE',  ( 23.15439245339999985, -19.47871561450000044, 1.365412016609999890 ) ) ;
#27458=ORIENTED_EDGE ( 'NONE', *, *, #896, .T. ) ;
#27459=CARTESIAN_POINT ( 'NONE',  ( -2.334489330849077504, -19.47731532786916375, -22.96368096735655939 ) ) ;
#27461=CARTESIAN_POINT ( 'NONE',  ( -2.380747058000000305, -45.96202241429999447, -24.01241749629999944 ) ) ;
#27463=AXIS2_PLACEMENT_3D ( 'NONE', #2569, #6931, #24849 ) ;
#27465=EDGE_CURVE ( 'NONE', #16196, #134, #23161, .T. ) ;
#27466=EDGE_CURVE ( 'NONE', #23918, #26338, #27551, .T. ) ;
#27467=DIRECTION ( 'NONE',  ( 0.5895034617991800063, 0.000000000000000000, 0.8077658500622459936 ) ) ;
#27469=CARTESIAN_POINT ( 'NONE',  ( 21.93056824629999824, -44.91471496930000029, -8.496651354669999989 ) ) ;
#27470=EDGE_CURVE ( 'NONE', #28564, #4268, #3725, .T. ) ;
#27471=CARTESIAN_POINT ( 'NONE',  ( -40.35498444542948704, -74.39270540183063929, -7.250043397214241736 ) ) ;
#27472=CARTESIAN_POINT ( 'NONE',  ( -32.77174707999999725, -82.25000000000000000, -21.60034937969999902 ) ) ;
#27477=CARTESIAN_POINT ( 'NONE',  ( -4.085620730619999885E-15, -74.00000000000000000, 1.176836406100000135E-15 ) ) ;
#27479=CYLINDRICAL_SURFACE ( 'NONE', #14852, 1.000000000000000888 ) ;
#27482=CARTESIAN_POINT ( 'NONE',  ( -38.62788659690000515, -74.00000000000000000, 7.627568735119999666 ) ) ;
#27483=AXIS2_PLACEMENT_3D ( 'NONE', #3802, #26523, #11035 ) ;
#27484=AXIS2_PLACEMENT_3D ( 'NONE', #16994, #4306, #1701 ) ;
#27485=DIRECTION ( 'NONE',  ( 0.000000000000000000, -1.000000000000000000, 0.000000000000000000 ) ) ;
#27487=CARTESIAN_POINT ( 'NONE',  ( -32.77174707999999725, -79.81706294759999309, -21.60034937969999902 ) ) ;
#27489=ORIENTED_EDGE ( 'NONE', *, *, #3818, .T. ) ;
#27492=CARTESIAN_POINT ( 'NONE',  ( -11.15184145912447811, -19.46488291679582261, 19.10630597097677352 ) ) ;
#27493=CARTESIAN_POINT ( 'NONE',  ( -7.415354059669999387, -73.99652904559999911, 39.14864742849999857 ) ) ;
#27495=DIRECTION ( 'NONE',  ( 1.000000000000000000, 0.000000000000000000, -1.261617073437678048E-15 ) ) ;
#27496=CARTESIAN_POINT ( 'NONE',  ( -7.242418265013072620, -74.21175622381174719, -40.33192879111471996 ) ) ;
#27497=EDGE_CURVE ( 'NONE', #6367, #898, #26590, .T. ) ;
#27499=DIRECTION ( 'NONE',  ( 0.000000000000000000, -1.000000000000000000, 0.000000000000000000 ) ) ;
#27501=ORIENTED_EDGE ( 'NONE', *, *, #5287, .F. ) ;
#27503=CYLINDRICAL_SURFACE ( 'NONE', #9844, 3.749999999999996447 ) ;
#27506=AXIS2_PLACEMENT_3D ( 'NONE', #22384, #4755, #702 ) ;
#27510=EDGE_LOOP ( 'NONE', ( #28766, #1345, #5417, #9022, #8274 ) ) ;
#27511=CARTESIAN_POINT ( 'NONE',  ( -2.352695545230000018, -57.85578495419999712, -24.35231633660000128 ) ) ;
#27512=DIRECTION ( 'NONE',  ( 1.000000000000000000, 0.000000000000000000, 0.000000000000000000 ) ) ;
#27517=VERTEX_POINT ( 'NONE', #11296 ) ;
#27518=CARTESIAN_POINT ( 'NONE',  ( 0.000000000000000000, -65.07443093669999712, 0.000000000000000000 ) ) ;
#27520=CARTESIAN_POINT ( 'NONE',  ( 21.30683598400000278, -36.18102154449999830, -9.649494700380000012 ) ) ;
#27523=AXIS2_PLACEMENT_3D ( 'NONE', #23325, #635, #27275 ) ;
#27528=CARTESIAN_POINT ( 'NONE',  ( -14.58849462870000124, -79.93035050890000548, 36.50501630579999812 ) ) ;
#27529=CARTESIAN_POINT ( 'NONE',  ( -1.469312066619999912, -66.04885972420001394, -25.55659601380000012 ) ) ;
#27533=ORIENTED_EDGE ( 'NONE', *, *, #8275, .T. ) ;
#27536=CARTESIAN_POINT ( 'NONE',  ( 23.40870129169999814, -59.03921360480000402, -0.5708451045399999257 ) ) ;
#27537=CARTESIAN_POINT ( 'NONE',  ( -21.09230234119999992, -65.00127803149999295, 13.73520459809999927 ) ) ;
#27538=ORIENTED_EDGE ( 'NONE', *, *, #7608, .T. ) ;
#27540=CARTESIAN_POINT ( 'NONE',  ( -7.283077424107684550, -73.99998247163075860, 39.66139668322427525 ) ) ;
#27541=CARTESIAN_POINT ( 'NONE',  ( 36.71809979542844360, -74.32420712084812919, -14.48873512655322671 ) ) ;
#27543=DIRECTION ( 'NONE',  ( 0.000000000000000000, -1.000000000000000000, 0.000000000000000000 ) ) ;
#27545=CARTESIAN_POINT ( 'NONE',  ( 8.468983517309998987, -34.90594137040000078, -20.83695881339999900 ) ) ;
#27548=EDGE_LOOP ( 'NONE', ( #4172, #23218, #19262, #9026 ) ) ;
#27549=VECTOR ( 'NONE', #4397, 1000.000000000000000 ) ;
#27551=CIRCLE ( 'NONE', #2876, 1.000000000000000888 ) ;
#27553=CARTESIAN_POINT ( 'NONE',  ( -11.39898658829999967, -18.85531877220000041, 18.89825401980000308 ) ) ;
#27558=ORIENTED_EDGE ( 'NONE', *, *, #4749, .T. ) ;
#27559=CARTESIAN_POINT ( 'NONE',  ( -11.33386635579999790, -27.06678469999999948, 19.29914645179999866 ) ) ;
#27560=CARTESIAN_POINT ( 'NONE',  ( 8.289122765224647083, -18.50000007361606436, -18.87681024063931545 ) ) ;
#27566=TOROIDAL_SURFACE ( 'NONE', #25299, 3.750000000000000000, 1.000000000000000000 ) ;
#27569=CARTESIAN_POINT ( 'NONE',  ( -10.55455086157921940, -19.48670042615375309, -21.19291729735819274 ) ) ;
#27574=CARTESIAN_POINT ( 'NONE',  ( 47.05374491310924157, -79.59514489290765482, -2.116163992179171949 ) ) ;
#27576=ADVANCED_FACE ( 'NONE', ( #11739 ), #12898, .T. ) ;
#27577=CARTESIAN_POINT ( 'NONE',  ( -32.67527180340000825, -79.69119431650000251, -22.00249031550000112 ) ) ;
#27579=B_SPLINE_CURVE_WITH_KNOTS ( 'NONE', 3,
 ( #5871, #10502, #3834, #12835, #14751, #23654 ),
 .UNSPECIFIED., .F., .F.,
 ( 4, 2, 4 ),
 ( 0.000000000000000000, 0.5000000000000000000, 1.000000000000000000 ),
 .UNSPECIFIED. ) ;
#27582=CARTESIAN_POINT ( 'NONE',  ( 32.39999999999999858, -82.50000000000000000, 3.967724586379999025E-15 ) ) ;
#27583=ORIENTED_EDGE ( 'NONE', *, *, #4603, .F. ) ;
#27585=CARTESIAN_POINT ( 'NONE',  ( -18.70529629369999824, -26.09793778670000108, 12.22846835330000026 ) ) ;
#27586=CARTESIAN_POINT ( 'NONE',  ( 40.70731707320000226, -82.25000000000000000, -7.215414233289999757 ) ) ;
#27588=CARTESIAN_POINT ( 'NONE',  ( 22.31839213210000139, -59.04258408700000160, -7.084352054500000051 ) ) ;
#27589=CARTESIAN_POINT ( 'NONE',  ( 0.000000000000000000, 0.000000000000000000, 0.000000000000000000 ) ) ;
#27590=CARTESIAN_POINT ( 'NONE',  ( -10.85441475189999849, -19.15747270589999829, 19.16405033270000047 ) ) ;
#27591=AXIS2_PLACEMENT_3D ( 'NONE', #18139, #13614, #15940 ) ;
#27592=ORIENTED_EDGE ( 'NONE', *, *, #25646, .F. ) ;
#27593=CARTESIAN_POINT ( 'NONE',  ( 8.797620038699999867, -37.04760834070000186, -21.76996719339999942 ) ) ;
#27594=FACE_BOUND ( 'NONE', #20110, .T. ) ;
#27595=CARTESIAN_POINT ( 'NONE',  ( 21.27769661889999853, -36.50665358839999897, -8.736999621189999843 ) ) ;
#27602=CARTESIAN_POINT ( 'NONE',  ( 47.11548663039999951, -79.82827424500000291, -1.752954514250000040 ) ) ;
#27603=CARTESIAN_POINT ( 'NONE',  ( 9.175396146610001580, -40.70401306919999485, -22.46104921330000082 ) ) ;
#27606=ADVANCED_FACE ( 'NONE', ( #9410 ), #27503, .F. ) ;
#27607=CARTESIAN_POINT ( 'NONE',  ( -40.35276762241279869, -74.22736093640011745, 7.241427273148282495 ) ) ;
#27610=EDGE_LOOP ( 'NONE', ( #13702, #27427, #20973, #2543 ) ) ;
#27611=CARTESIAN_POINT ( 'NONE',  ( 19.07516306020000130, -18.50000000000000000, -8.007516059049999413 ) ) ;
#27614=AXIS2_PLACEMENT_3D ( 'NONE', #21404, #26208, #28233 ) ;
#27615=CARTESIAN_POINT ( 'NONE',  ( -2.582078993590000149, -32.66150190429999611, -24.62446518169999976 ) ) ;
#27618=DIRECTION ( 'NONE',  ( 1.000000000000000000, 0.000000000000000000, 0.000000000000000000 ) ) ;
#27619=CARTESIAN_POINT ( 'NONE',  ( 22.93608650079999833, -36.50000000029999825, -9.381593461610000517 ) ) ;
#27620=CARTESIAN_POINT ( 'NONE',  ( -39.31221710997630936, -74.09469053470054689, -7.479534728624519957 ) ) ;
#27622=ORIENTED_EDGE ( 'NONE', *, *, #25799, .F. ) ;
#27624=CARTESIAN_POINT ( 'NONE',  ( 47.16974535660000356, -74.50000000000000000, -1.075756255579999987 ) ) ;
#27627=CARTESIAN_POINT ( 'NONE',  ( 8.396977894420000865, -36.03998444319999805, -21.19011196440000333 ) ) ;
#27629=B_SPLINE_CURVE_WITH_KNOTS ( 'NONE', 3,
 ( #15374, #20467, #8676, #18288, #535, #6222, #5019, #17588, #13908, #26477, #17299, #15936, #27178, #12894, #26191, #22810, #24287, #4329, #15087, #2848, #22111 ),
 .UNSPECIFIED., .F., .F.,
 ( 4, 2, 2, 1, 2, 2, 2, 2, 2, 2, 4 ),
 ( 0.000000000000000000, 0.2499999999999882316, 0.3749999999999823475, 0.4374999999999761302, 0.4687499999999980016, 0.5000000000000199840, 0.6250000000000873746, 0.6875000000000981437, 0.7187500000000924816, 0.7500000000000868194, 1.000000000000000000 ),
 .UNSPECIFIED. ) ;
#27631=TOROIDAL_SURFACE ( 'NONE', #15470, 3.750000000000000000, 1.000000000000000000 ) ;
#27635=ORIENTED_EDGE ( 'NONE', *, *, #3856, .T. ) ;
#27636=CARTESIAN_POINT ( 'NONE',  ( -32.77174707999999725, -79.50000000000000000, -21.60034937969999902 ) ) ;
#27638=CARTESIAN_POINT ( 'NONE',  ( -12.89904789370000060, -65.07443093669999712, -21.58991903219999742 ) ) ;
#27639=ORIENTED_EDGE ( 'NONE', *, *, #21386, .T. ) ;
#27640=FACE_OUTER_BOUND ( 'NONE', #10150, .T. ) ;
#27642=CARTESIAN_POINT ( 'NONE',  ( -7.310176754529999599, -73.98157068460000119, 39.44185033859999834 ) ) ;
#27645=DIRECTION ( 'NONE',  ( 0.000000000000000000, 1.000000000000000000, 0.000000000000000000 ) ) ;
#27646=CARTESIAN_POINT ( 'NONE',  ( 26.61374759190000105, -73.81001964159999318, -28.89513312169999892 ) ) ;
#27652=AXIS2_PLACEMENT_3D ( 'NONE', #16944, #17072, #10624 ) ;
#27654=ORIENTED_EDGE ( 'NONE', *, *, #8825, .T. ) ;
#27655=CARTESIAN_POINT ( 'NONE',  ( 9.444187806723459033, -35.99901531098080909, -19.97576011151723563 ) ) ;
#27656=EDGE_CURVE ( 'NONE', #5033, #10479, #4656, .T. ) ;
#27658=CIRCLE ( 'NONE', #26702, 39.25000000000000000 ) ;
#27661=CARTESIAN_POINT ( 'NONE',  ( 11.31764183700000004, -36.00000000000000000, -22.43277176020000141 ) ) ;
#27664=ORIENTED_EDGE ( 'NONE', *, *, #12445, .F. ) ;
#27665=EDGE_CURVE ( 'NONE', #1691, #4525, #25012, .T. ) ;
#27666=EDGE_CURVE ( 'NONE', #7650, #16368, #12105, .T. ) ;
#27668=CARTESIAN_POINT ( 'NONE',  ( -7.135467692470220946, -73.63090023098223469, 38.71641001238775459 ) ) ;
#27669=CYLINDRICAL_SURFACE ( 'NONE', #21013, 4.750000000000001776 ) ;
#27675=CARTESIAN_POINT ( 'NONE',  ( -36.59277592640000165, -74.50000000000000000, -25.98617420859999783 ) ) ;
#27677=CARTESIAN_POINT ( 'NONE',  ( 36.49700125519999716, -74.06833701100001122, -14.20639533249999964 ) ) ;
#27680=ORIENTED_EDGE ( 'NONE', *, *, #22748, .T. ) ;
#27683=CARTESIAN_POINT ( 'NONE',  ( -7.250391496897478305, -74.00000000000000000, 39.93225832964911604 ) ) ;
#27684=CARTESIAN_POINT ( 'NONE',  ( 36.61782233228550609, -74.16892777906130618, -14.30620871315702658 ) ) ;
#27688=CARTESIAN_POINT ( 'NONE',  ( -31.99304886599999875, -74.00000000020000357, -21.98470665500000010 ) ) ;
#27689=DIRECTION ( 'NONE',  ( 0.000000000000000000, 1.000000000000000000, 0.000000000000000000 ) ) ;
#27690=CARTESIAN_POINT ( 'NONE',  ( 0.000000000000000000, -18.50000000000000000, 0.000000000000000000 ) ) ;
#27692=VECTOR ( 'NONE', #16260, 1000.000000000000114 ) ;
#27693=AXIS2_PLACEMENT_3D ( 'NONE', #3975, #17233, #8072 ) ;
#27694=EDGE_CURVE ( 'NONE', #17770, #26105, #25586, .T. ) ;
#27696=EDGE_LOOP ( 'NONE', ( #2276, #6857, #20398, #16321 ) ) ;
#27697=CARTESIAN_POINT ( 'NONE',  ( 47.16888291020000423, -74.56821585100000505, -1.104556675960000067 ) ) ;
#27698=ORIENTED_EDGE ( 'NONE', *, *, #6345, .T. ) ;
#27699=AXIS2_PLACEMENT_3D ( 'NONE', #12543, #14876, #5862 ) ;
#27700=CARTESIAN_POINT ( 'NONE',  ( -11.25709297429999900, -19.46485661140000190, 19.04110009109999879 ) ) ;
#27703=CARTESIAN_POINT ( 'NONE',  ( 45.84677420572959505, -80.34292036800317760, -4.286925633470588082 ) ) ;
#27704=CARTESIAN_POINT ( 'NONE',  ( 40.28438195609999894, -74.37144044050000957, 7.256982118289999839 ) ) ;
#27705=CARTESIAN_POINT ( 'NONE',  ( -10.51051889136755513, -19.48405220144317695, -21.03322345498822443 ) ) ;
#27706=CARTESIAN_POINT ( 'NONE',  ( 25.53957162523754576, -69.04156329992152052, -8.628252605428819777 ) ) ;
#27707=CARTESIAN_POINT ( 'NONE',  ( -11.67416330133831437, -61.62341122741943877, -23.03586770298056052 ) ) ;
#27710=CARTESIAN_POINT ( 'NONE',  ( -6.322973885729999743, -74.00000000000000000, 35.51864961870000315 ) ) ;
#27711=CARTESIAN_POINT ( 'NONE',  ( 8.508194237257523440, -34.61672934516087707, -20.76917592404496204 ) ) ;
#27714=ORIENTED_EDGE ( 'NONE', *, *, #14200, .T. ) ;
#27715=CARTESIAN_POINT ( 'NONE',  ( -2.874157831770000282, -80.49856749429999070, 46.70286942899999616 ) ) ;
#27720=DIRECTION ( 'NONE',  ( 0.000000000000000000, 1.000000000000000000, 0.000000000000000000 ) ) ;
#27721=FACE_OUTER_BOUND ( 'NONE', #22158, .T. ) ;
#27725=ADVANCED_FACE ( 'NONE', ( #10254 ), #19437, .T. ) ;
#27727=VERTEX_POINT ( 'NONE', #13455 ) ;
#27728=CARTESIAN_POINT ( 'NONE',  ( 20.43617771219999923, -55.54030921969999923, 11.17804412479999954 ) ) ;
#27729=FACE_OUTER_BOUND ( 'NONE', #13056, .T. ) ;
#27730=AXIS2_PLACEMENT_3D ( 'NONE', #13399, #13550, #26680 ) ;
#27733=CARTESIAN_POINT ( 'NONE',  ( 8.028473304129999377, -18.50000000000000000, -18.85230009969999898 ) ) ;
#27736=CARTESIAN_POINT ( 'NONE',  ( 9.449797638950000689, -44.86350384200000008, -23.17371582650000050 ) ) ;
#27738=ORIENTED_EDGE ( 'NONE', *, *, #7421, .F. ) ;
#27739=CARTESIAN_POINT ( 'NONE',  ( -39.65872146214135796, -73.77182148721053068, 7.242474372565215646 ) ) ;
#27740=CARTESIAN_POINT ( 'NONE',  ( 23.69918219720000252, -19.41822431039999941, 1.513728844550000119 ) ) ;
#27742=ORIENTED_EDGE ( 'NONE', *, *, #12736, .F. ) ;
#27744=DIRECTION ( 'NONE',  ( -0.3687499999999825917, 0.000000000000000000, 0.9295286103719523352 ) ) ;
#27745=CARTESIAN_POINT ( 'NONE',  ( -0.5567039383430000266, -26.09744228910000174, -22.25837505089999979 ) ) ;
#27746=FACE_OUTER_BOUND ( 'NONE', #19629, .T. ) ;
#27747=CARTESIAN_POINT ( 'NONE',  ( -0.3035179129464828374, -74.42029229106765342, 47.25000000000000000 ) ) ;
#27749=CARTESIAN_POINT ( 'NONE',  ( 22.33517371069999768, -36.52243084719999899, -9.146761579799999708 ) ) ;
#27753=EDGE_CURVE ( 'NONE', #5069, #4593, #13754, .T. ) ;
#27757=VECTOR ( 'NONE', #643, 1000.000000000000000 ) ;
#27760=CARTESIAN_POINT ( 'NONE',  ( 20.87697854030000144, -35.04923858010000970, -8.448077735809999211 ) ) ;
#27763=CYLINDRICAL_SURFACE ( 'NONE', #14211, 1.000000000000000000 ) ;
#27766=CARTESIAN_POINT ( 'NONE',  ( 32.43349014520016027, -74.01270418637506054, -21.45979546804144178 ) ) ;
#27767=CARTESIAN_POINT ( 'NONE',  ( 18.94592261899999741, -19.50000000000000000, -9.024080787800000891 ) ) ;
#27769=CARTESIAN_POINT ( 'NONE',  ( -25.98617420859999783, -77.00000000000000000, -36.59277592640000165 ) ) ;
#27771=CARTESIAN_POINT ( 'NONE',  ( -7.319780978429999863, -73.91748504689999777, 39.18460075750000016 ) ) ;
#27774=CARTESIAN_POINT ( 'NONE',  ( 20.36016146999999776, -74.00000000000000000, -32.97008227039999895 ) ) ;
#27776=CARTESIAN_POINT ( 'NONE',  ( -12.17175180279999935, -57.47855601759999900, -19.93971687999999887 ) ) ;
#27777=DIRECTION ( 'NONE',  ( 1.000000000000000000, 0.000000000000000000, 0.000000000000000000 ) ) ;
#27778=CARTESIAN_POINT ( 'NONE',  ( 8.976488324580000011, -22.51608882080000029, -19.49531134190000259 ) ) ;
#27779=DIRECTION ( 'NONE',  ( 0.000000000000000000, -1.000000000000000000, 0.000000000000000000 ) ) ;
#27780=EDGE_LOOP ( 'NONE', ( #1638, #21617, #10068, #17160, #26717, #25402 ) ) ;
#27781=EDGE_CURVE ( 'NONE', #20206, #12333, #10817, .T. ) ;
#27782=DIRECTION ( 'NONE',  ( 0.000000000000000000, 1.000000000000000000, 0.000000000000000000 ) ) ;
#27783=ORIENTED_EDGE ( 'NONE', *, *, #25419, .T. ) ;
#27784=EDGE_CURVE ( 'NONE', #20968, #26598, #28713, .T. ) ;
#27786=LINE ( 'NONE', #12178, #21614 ) ;
#27789=CARTESIAN_POINT ( 'NONE',  ( -20.45998242170000125, -52.56313962710000709, 14.78974999389999923 ) ) ;
#27791=LINE ( 'NONE', #7832, #18100 ) ;
#27793=CARTESIAN_POINT ( 'NONE',  ( -37.60355029590000697, -84.00000000000000000, 9.356041104380000917 ) ) ;
#27794=CARTESIAN_POINT ( 'NONE',  ( 7.707964880030000465, -36.74561153859999507, -21.48083100459999883 ) ) ;
#27796=CARTESIAN_POINT ( 'NONE',  ( -15.31688208200000112, -69.70331854509998948, 22.99240601979999710 ) ) ;
#27798=CARTESIAN_POINT ( 'NONE',  ( 46.25000000000000000, -75.00000000000000000, -13.75000000000000000 ) ) ;
#27799=AXIS2_PLACEMENT_3D ( 'NONE', #10798, #15033, #23948 ) ;
#27801=CARTESIAN_POINT ( 'NONE',  ( 23.62253742169999882, -60.59277760239999822, -0.2692575271260000402 ) ) ;
#27802=DIRECTION ( 'NONE',  ( 1.000000000000000000, 0.000000000000000000, 0.000000000000000000 ) ) ;
#27803=ORIENTED_EDGE ( 'NONE', *, *, #4198, .T. ) ;
#27804=FACE_OUTER_BOUND ( 'NONE', #16349, .T. ) ;
#27805=CARTESIAN_POINT ( 'NONE',  ( 18.93437244977972611, -18.87168146926155643, -8.901252598746989264 ) ) ;
#27807=ORIENTED_EDGE ( 'NONE', *, *, #24306, .F. ) ;
#27812=CARTESIAN_POINT ( 'NONE',  ( 7.318372426699999878, -73.93831497249999529, 38.68350751799999898 ) ) ;
#27816=B_SPLINE_SURFACE_WITH_KNOTS ( 'NONE', 5, 5, ( 
 ( #10633, #6589, #19547, #15451, #19977, #15015 ),
 ( #17371, #22036, #13270, #50, #26115, #10494 ),
 ( #3967, #28579, #2219, #28435, #8895, #12689 ),
 ( #19409, #17809, #19689, #8613, #14879, #23787 ),
 ( #28290, #6142, #23929, #17515, #2084, #26401 ),
 ( #6431, #19830, #17954, #4845, #5134, #11519 ) ),
 .UNSPECIFIED., .F., .F., .F.,
 ( 6, 6 ),
 ( 6, 6 ),
 ( 13.75601705980000133, 16.62037739340000186 ),
 ( 0.000000000000000000, 2.000000000000000000 ),
 .UNSPECIFIED. ) ;
#27817=CARTESIAN_POINT ( 'NONE',  ( 36.92830089767138446, -79.76883227166896972, -14.38962487061029272 ) ) ;
#27819=PLANE ( 'NONE',  #22235 ) ;
#27826=ORIENTED_EDGE ( 'NONE', *, *, #7093, .T. ) ;
#27828=ADVANCED_FACE ( 'NONE', ( #2555 ), #6472, .F. ) ;
#27832=CYLINDRICAL_SURFACE ( 'NONE', #18104, 4.750000000000000888 ) ;
#27833=CARTESIAN_POINT ( 'NONE',  ( 47.02598405681334981, -79.63081725461873361, -2.257492274610140015 ) ) ;
#27834=ORIENTED_EDGE ( 'NONE', *, *, #1133, .T. ) ;
#27835=CARTESIAN_POINT ( 'NONE',  ( 46.25000000000000000, -79.00000000000000000, -13.75000000000000000 ) ) ;
#27836=DIRECTION ( 'NONE',  ( 0.7071067811865475727, 0.000000000000000000, -0.7071067811865475727 ) ) ;
#27838=CARTESIAN_POINT ( 'NONE',  ( -1.157192565939999973, -53.84184168659999870, -23.27396048310000154 ) ) ;
#27839=CARTESIAN_POINT ( 'NONE',  ( -1.540392455020000106, -79.77809169310000925, 47.20175211690000339 ) ) ;
#27842=DIRECTION ( 'NONE',  ( 1.000000000000000000, 0.000000000000000000, 0.000000000000000000 ) ) ;
#27843=DIRECTION ( 'NONE',  ( 0.000000000000000000, 0.000000000000000000, -1.000000000000000000 ) ) ;
#27845=CARTESIAN_POINT ( 'NONE',  ( 29.82685776330000138, -73.10703858080000828, -25.25856749939999801 ) ) ;
#27847=( LENGTH_UNIT ( ) NAMED_UNIT ( * ) SI_UNIT ( .MILLI., .METRE. ) );
#27850=CARTESIAN_POINT ( 'NONE',  ( -40.08893529113748855, -74.03750509262607693, -7.249551406113103447 ) ) ;
#27851=ORIENTED_EDGE ( 'NONE', *, *, #13945, .F. ) ;
#27853=TOROIDAL_SURFACE ( 'NONE', #14813, 3.500000000000000000, 0.5000000000000000000 ) ;
#27856=CARTESIAN_POINT ( 'NONE',  ( 3.907985046679999924E-15, -73.50000000000000000, -40.00000000000000000 ) ) ;
#27858=ORIENTED_EDGE ( 'NONE', *, *, #9782, .T. ) ;
#27864=CARTESIAN_POINT ( 'NONE',  ( -40.39659210501955044, -74.26034152734142424, 7.239203719547485427 ) ) ;
#27868=CARTESIAN_POINT ( 'NONE',  ( 18.94592261899999741, -19.18584073480000285, -9.024080787970000017 ) ) ;
#27869=EDGE_CURVE ( 'NONE', #19768, #28710, #2996, .T. ) ;
#27870=CARTESIAN_POINT ( 'NONE',  ( -14.06220372179999956, -74.01102208230000201, 36.25327798059999651 ) ) ;
#27872=CARTESIAN_POINT ( 'NONE',  ( 7.627566167509999495, -74.00000000000000000, -38.62788938250000115 ) ) ;
#27873=EDGE_CURVE ( 'NONE', #10298, #14992, #5010, .T. ) ;
#27874=CARTESIAN_POINT ( 'NONE',  ( -1.328705758835786233, -74.17186053442132732, 47.12725970932369535 ) ) ;
#27876=CARTESIAN_POINT ( 'NONE',  ( 22.33353630010000046, -57.45905992459999823, -8.600016955360000992 ) ) ;
#27878=CARTESIAN_POINT ( 'NONE',  ( 8.408940298597524787, -35.33620340784488434, -20.95510887256177313 ) ) ;
#27879=CARTESIAN_POINT ( 'NONE',  ( -10.83788578300000083, -34.62274519420000018, -21.57372758079999997 ) ) ;
#27889=LINE ( 'NONE', #3290, #22800 ) ;
#27892=CARTESIAN_POINT ( 'NONE',  ( 20.82664911639999872, -28.53805357630000117, -8.124862095080001012 ) ) ;
#27893=CARTESIAN_POINT ( 'NONE',  ( 27.89292634430000106, -72.00000000000000000, 12.34776042340000046 ) ) ;
#27895=CIRCLE ( 'NONE', #12970, 6.749999999999999112 ) ;
#27897=DIRECTION ( 'NONE',  ( 1.000000000000000000, 0.000000000000000000, 0.000000000000000000 ) ) ;
#27898=ORIENTED_EDGE ( 'NONE', *, *, #9274, .T. ) ;
#27900=CARTESIAN_POINT ( 'NONE',  ( 7.215414233289999757, -74.50000000000000000, -40.70731707320000226 ) ) ;
#27901=ORIENTED_EDGE ( 'NONE', *, *, #23120, .F. ) ;
#27903=EDGE_CURVE ( 'NONE', #1018, #10833, #847, .T. ) ;
#27904=AXIS2_PLACEMENT_3D ( 'NONE', #18346, #5510, #7272 ) ;
#27908=B_SPLINE_CURVE_WITH_KNOTS ( 'NONE', 5,
 ( #10163, #19634, #26055, #19217, #10573, #3909, #21685, #3499, #28104 ),
 .UNSPECIFIED., .F., .F.,
 ( 6, 3, 6 ),
 ( 0.000000000000000000, 0.5000000000000000000, 1.000000000000000000 ),
 .UNSPECIFIED. ) ;
#27910=EDGE_CURVE ( 'NONE', #28554, #25683, #15798, .T. ) ;
#27911=CARTESIAN_POINT ( 'NONE',  ( 26.58635620580000136, -73.91993066429999715, -28.92424498180000114 ) ) ;
#27916=CARTESIAN_POINT ( 'NONE',  ( -11.91832687610000185, -65.33654462490000014, -22.94749264700000069 ) ) ;
#27917=DIRECTION ( 'NONE',  ( 0.5503789995269310342, 0.000000000000000000, -0.8349149399068952482 ) ) ;
#27918=CARTESIAN_POINT ( 'NONE',  ( 19.36781163719999910, -19.46510053389999939, 10.50580276810000058 ) ) ;
#27919=VERTEX_POINT ( 'NONE', #22803 ) ;
#27920=CARTESIAN_POINT ( 'NONE',  ( 32.75000000000000000, -73.00000000000000000, 1.546052475400000102E-15 ) ) ;
#27922=AXIS2_PLACEMENT_3D ( 'NONE', #8588, #17491, #15424 ) ;
#27924=FACE_OUTER_BOUND ( 'NONE', #21007, .T. ) ;
#27926=CARTESIAN_POINT ( 'NONE',  ( 46.25000000000000000, -77.00000000000000000, -14.75000000000000000 ) ) ;
#27934=ADVANCED_FACE ( 'NONE', ( #2841 ), #7811, .T. ) ;
#27935=TOROIDAL_SURFACE ( 'NONE', #1430, 10.50000000000000000, 0.5000000000000000000 ) ;
#27938=CIRCLE ( 'NONE', #24212, 11.00000000000000000 ) ;
#27939=EDGE_CURVE ( 'NONE', #13659, #17905, #28245, .T. ) ;
#27940=DIRECTION ( 'NONE',  ( -1.000000000000000000, 0.000000000000000000, 0.000000000000000000 ) ) ;
#27945=VERTEX_POINT ( 'NONE', #9526 ) ;
#27947=CARTESIAN_POINT ( 'NONE',  ( -1.684828471230000124, -18.50000000000000000, -21.44817583509999892 ) ) ;
#27950=CARTESIAN_POINT ( 'NONE',  ( 0.000000000000000000, -84.00000000000000000, 40.00000000000000000 ) ) ;
#27951=CARTESIAN_POINT ( 'NONE',  ( -9.597487326430000465, -80.00000000000000000, 38.57396449699999863 ) ) ;
#27952=DIRECTION ( 'NONE',  ( 0.000000000000000000, -1.000000000000000000, 0.000000000000000000 ) ) ;
#27953=VERTEX_POINT ( 'NONE', #23096 ) ;
#27954=CARTESIAN_POINT ( 'NONE',  ( 36.86594131523432338, -79.67252481679619791, -14.49340671423261462 ) ) ;
#27956=TOROIDAL_SURFACE ( 'NONE', #16791, 3.500000000000000000, 0.5000000000000000000 ) ;
#27958=CIRCLE ( 'NONE', #18685, 2.000000000000000000 ) ;
#27959=ORIENTED_EDGE ( 'NONE', *, *, #27666, .T. ) ;
#27961=CARTESIAN_POINT ( 'NONE',  ( 47.18156631880000162, -74.63487131880000902, -1.134746784699999900 ) ) ;
#27965=ORIENTED_EDGE ( 'NONE', *, *, #21438, .F. ) ;
#27970=CARTESIAN_POINT ( 'NONE',  ( 40.70731707320000226, -74.50000000000000000, 7.215414233289999757 ) ) ;
#27972=EDGE_CURVE ( 'NONE', #3865, #23386, #26545, .T. ) ;
#27973=CARTESIAN_POINT ( 'NONE',  ( 20.34628061889999984, -52.63293862049999916, 11.13082833170000008 ) ) ;
#27974=CARTESIAN_POINT ( 'NONE',  ( 4.929390229339999696E-15, -84.50000000000000000, 40.00000000000000000 ) ) ;
#27975=ORIENTED_EDGE ( 'NONE', *, *, #19305, .F. ) ;
#27977=CARTESIAN_POINT ( 'NONE',  ( 8.988996100299999625, -34.66800400750000222, -19.43643858049999906 ) ) ;
#27981=CARTESIAN_POINT ( 'NONE',  ( -3.072375608539999803, -79.99928376260000107, 46.95756812850000017 ) ) ;
#27982=CARTESIAN_POINT ( 'NONE',  ( -15.04362262010000073, -66.18012799950000158, 22.59069390079999806 ) ) ;
#27983=ORIENTED_EDGE ( 'NONE', *, *, #27129, .T. ) ;
#27985=CARTESIAN_POINT ( 'NONE',  ( -17.42343749999999858, -77.00000000000000000, 43.92022684009999978 ) ) ;
#27987=DIRECTION ( 'NONE',  ( 1.000000000000000000, 0.000000000000000000, 0.000000000000000000 ) ) ;
#27988=CARTESIAN_POINT ( 'NONE',  ( 38.65106240728522380, -73.99999920929936081, 7.498734568567305914 ) ) ;
#27989=CARTESIAN_POINT ( 'NONE',  ( 29.90404901189999620, -73.44398176539999668, -25.16348247620000222 ) ) ;
#27990=CARTESIAN_POINT ( 'NONE',  ( -14.47589974207729568, -74.09467030769806684, 36.25997764697337544 ) ) ;
#27991=DIRECTION ( 'NONE',  ( 1.000000000000000000, 0.000000000000000000, 0.000000000000000000 ) ) ;
#27995=CARTESIAN_POINT ( 'NONE',  ( 20.57859482010000107, -35.48124439810000297, -8.749812979389998802 ) ) ;
#28000=AXIS2_PLACEMENT_3D ( 'NONE', #2369, #25100, #4691 ) ;
#28003=EDGE_CURVE ( 'NONE', #3837, #17168, #25931, .T. ) ;
#28011=CARTESIAN_POINT ( 'NONE',  ( 7.215414233289999757, -74.50000000000000000, -40.70731707320000226 ) ) ;
#28012=CARTESIAN_POINT ( 'NONE',  ( -13.00673796568629648, -19.48509974121062172, 19.66549047931116689 ) ) ;
#28015=CARTESIAN_POINT ( 'NONE',  ( 18.94592261899999741, -19.50000000009999823, -9.024080787920000901 ) ) ;
#28016=FACE_OUTER_BOUND ( 'NONE', #28225, .T. ) ;
#28017=DIRECTION ( 'NONE',  ( 0.000000000000000000, 1.000000000000000000, 0.000000000000000000 ) ) ;
#28021=CYLINDRICAL_SURFACE ( 'NONE', #17439, 0.4999999999999982236 ) ;
#28025=CARTESIAN_POINT ( 'NONE',  ( 21.12062292599999580, -58.34046154589999844, 10.52028212929999995 ) ) ;
#28026=DIRECTION ( 'NONE',  ( 0.000000000000000000, 1.000000000000000000, 0.000000000000000000 ) ) ;
#28027=TOROIDAL_SURFACE ( 'NONE', #16396, 9.000000000000000000, 2.000000000000000000 ) ;
#28028=EDGE_LOOP ( 'NONE', ( #3705, #28521, #18768, #8402 ) ) ;
#28029=ADVANCED_FACE ( 'NONE', ( #12280 ), #12434, .T. ) ;
#28034=ADVANCED_FACE ( 'NONE', ( #25701 ), #22697, .T. ) ;
#28037=DIRECTION ( 'NONE',  ( 0.000000000000000000, -1.000000000000000000, 0.000000000000000000 ) ) ;
#28046=CARTESIAN_POINT ( 'NONE',  ( -7.346953802149999824, -74.24999999150000463, 39.87739400550000113 ) ) ;
#28047=CARTESIAN_POINT ( 'NONE',  ( 46.25000000000000000, -80.00000000000000000, -4.582575694960000057 ) ) ;
#28049=CARTESIAN_POINT ( 'NONE',  ( 27.75394116159999669, -74.50000000000000000, -27.75394116159999669 ) ) ;
#28050=CARTESIAN_POINT ( 'NONE',  ( 10.20110288159999890, -74.00000000000000000, -41.00000000000000000 ) ) ;
#28051=PRODUCT_DEFINITION_SHAPE ( 'NONE', 'NONE',  #28060 ) ;
#28052=CYLINDRICAL_SURFACE ( 'NONE', #5546, 39.24999999999998579 ) ;
#28053=CARTESIAN_POINT ( 'NONE',  ( -11.77695074510000062, -64.47177033809998647, -23.22164031879999868 ) ) ;
#28056=EDGE_LOOP ( 'NONE', ( #22446, #17526, #6084, #21990, #17017 ) ) ;
#28058=AXIS2_PLACEMENT_3D ( 'NONE', #26857, #22490, #6752 ) ;
#28060=PRODUCT_DEFINITION ( 'UNKNOWN', '', #2266, #4506 ) ;
#28061=AXIS2_PLACEMENT_3D ( 'NONE', #3326, #14252, #23141 ) ;
#28062=ADVANCED_FACE ( 'NONE', ( #19133 ), #24070, .F. ) ;
#28063=CARTESIAN_POINT ( 'NONE',  ( -2.605870651600000087, -64.47177090210000472, -25.91540045190000185 ) ) ;
#28066=CARTESIAN_POINT ( 'NONE',  ( -19.54048411319999801, -52.63055504209999924, 12.61913916920000034 ) ) ;
#28069=AXIS2_PLACEMENT_3D ( 'NONE', #16377, #19412, #25705 ) ;
#28071=CARTESIAN_POINT ( 'NONE',  ( -7.627568735119999666, -74.00000000000000000, -38.62788659690000515 ) ) ;
#28072=ORIENTED_EDGE ( 'NONE', *, *, #27159, .T. ) ;
#28073=CARTESIAN_POINT ( 'NONE',  ( 7.533204440554428061, -37.08603407206901892, -21.49405318675248822 ) ) ;
#28074=CARTESIAN_POINT ( 'NONE',  ( -14.59919346459999900, -79.65691081869999834, 36.80099829179999205 ) ) ;
#28075=CIRCLE ( 'NONE', #3879, 1.999999999999999112 ) ;
#28077=FACE_OUTER_BOUND ( 'NONE', #19228, .T. ) ;
#28079=CARTESIAN_POINT ( 'NONE',  ( -20.00096871140000232, -59.03952408640000016, 12.17600098870000203 ) ) ;
#28080=EDGE_LOOP ( 'NONE', ( #3583, #6762, #9098 ) ) ;
#28081=CARTESIAN_POINT ( 'NONE',  ( 23.73263625450000092, -64.92652906329999496, -8.873745374080000303 ) ) ;
#28083=CARTESIAN_POINT ( 'NONE',  ( -1.797800075250000074, -19.46723765599999822, -22.31531904799999921 ) ) ;
#28085=ORIENTED_EDGE ( 'NONE', *, *, #24110, .F. ) ;
#28086=CIRCLE ( 'NONE', #10367, 3.749999999999996447 ) ;
#28090=EDGE_LOOP ( 'NONE', ( #10548, #2937, #16799, #7230 ) ) ;
#28091=ADVANCED_FACE ( 'NONE', ( #5133 ), #17839, .F. ) ;
#28093=AXIS2_PLACEMENT_3D ( 'NONE', #18087, #26841, #2512 ) ;
#28097=CARTESIAN_POINT ( 'NONE',  ( 47.25003994149999897, -74.79572188120000931, -0.5609601642099999452 ) ) ;
#28099=CARTESIAN_POINT ( 'NONE',  ( 20.53262164509999721, -53.84414347720000649, 10.87832573719999907 ) ) ;
#28101=CARTESIAN_POINT ( 'NONE',  ( -7.261004788010000155, -74.03378462380000258, -40.00100507770000036 ) ) ;
#28104=CARTESIAN_POINT ( 'NONE',  ( 22.43277176080000146, -36.00000000000000000, -11.31764183710000005 ) ) ;
#28108=DIRECTION ( 'NONE',  ( 0.4794255386042040601, 0.000000000000000000, 0.8775825618903720926 ) ) ;
#28110=CARTESIAN_POINT ( 'NONE',  ( 25.04851980253549470, -66.68373043499040875, 10.87574838088278106 ) ) ;
#28112=CARTESIAN_POINT ( 'NONE',  ( 9.393614001710000494, -38.00000000000000000, -22.97877290430000130 ) ) ;
#28117=CIRCLE ( 'NONE', #239, 6.749999999999999112 ) ;
#28119=CARTESIAN_POINT ( 'NONE',  ( -19.23238473919999691, -19.17792668139999890, 14.16443425210000129 ) ) ;
#28120=ORIENTED_EDGE ( 'NONE', *, *, #5966, .T. ) ;
#28124=CARTESIAN_POINT ( 'NONE',  ( 8.563236930420002224, -35.95760432990000055, -20.91612140590000024 ) ) ;
#28129=AXIS2_PLACEMENT_3D ( 'NONE', #107, #8955, #27048 ) ;
#28135=CARTESIAN_POINT ( 'NONE',  ( 20.19624812569999861, -35.90543013560000674, -9.066694748779999813 ) ) ;
#28139=CARTESIAN_POINT ( 'NONE',  ( 7.595444726729600567E-15, -73.50000000000000000, 32.25000000000000000 ) ) ;
#28140=CARTESIAN_POINT ( 'NONE',  ( -0.5856137342820000313, -19.46510053389999939, -22.02591827759999887 ) ) ;
#28141=TOROIDAL_SURFACE ( 'NONE', #14659, 0.5000000000000000000, 0.5000000000000000000 ) ;
#28143=CARTESIAN_POINT ( 'NONE',  ( 9.307783803350000440, -57.43039249360000298, -22.95932595720000080 ) ) ;
#28145=ORIENTED_EDGE ( 'NONE', *, *, #25811, .F. ) ;
#28146=CARTESIAN_POINT ( 'NONE',  ( -40.00000000000000000, -82.25000000000000000, 0.000000000000000000 ) ) ;
#28149=ORIENTED_EDGE ( 'NONE', *, *, #3151, .T. ) ;
#28152=B_SPLINE_CURVE_WITH_KNOTS ( 'NONE', 3,
 ( #28641, #19616, #22106, #15218, #12888, #15369, #17583, #19900, #26471, #6508, #17009, #5922, #14806, #17734 ),
 .UNSPECIFIED., .F., .F.,
 ( 4, 2, 1, 1, 1, 1, 2, 2, 4 ),
 ( 0.000000000000000000, 0.2499999999998663291, 0.3749999999998062661, 0.4374999999997802869, 0.4687499999997731814, 0.4843749999997706279, 0.4921874999997750688, 0.4999999999997795097, 1.000000000000000000 ),
 .UNSPECIFIED. ) ;
#28153=CARTESIAN_POINT ( 'NONE',  ( -14.57172147319999844, -74.36322263760000340, 36.76767988459999970 ) ) ;
#28156=VERTEX_POINT ( 'NONE', #17185 ) ;
#28157=B_SPLINE_CURVE_WITH_KNOTS ( 'NONE', 5,
 ( #7582, #3201, #27239, #5516, #7277, #14403 ),
 .UNSPECIFIED., .F., .F.,
 ( 6, 6 ),
 ( 0.000000000000000000, 1.000000000000000000 ),
 .UNSPECIFIED. ) ;
#28158=CARTESIAN_POINT ( 'NONE',  ( -4.439198032609999743E-16, -74.50000000000000000, 47.25000000000000000 ) ) ;
#28160=CARTESIAN_POINT ( 'NONE',  ( 9.864792964790000340, -62.95257329789999545, -24.33712608820000156 ) ) ;
#28161=CARTESIAN_POINT ( 'NONE',  ( -38.71640869449999656, -73.50000064450000536, -7.135466578850000019 ) ) ;
#28162=CARTESIAN_POINT ( 'NONE',  ( 20.51027264869999911, -57.91805294160000273, 11.21560916570000010 ) ) ;
#28163=CARTESIAN_POINT ( 'NONE',  ( -10.93265203729999868, -19.39368411250000079, -21.85641315899999881 ) ) ;
#28174=CARTESIAN_POINT ( 'NONE',  ( 20.76917537310000128, -34.61672842239999426, -8.508194708340001355 ) ) ;
#28176=DIRECTION ( 'NONE',  ( 0.000000000000000000, 1.000000000000000000, 0.000000000000000000 ) ) ;
#28177=EDGE_LOOP ( 'NONE', ( #17341, #16678, #14949, #24156 ) ) ;
#28183=DIRECTION ( 'NONE',  ( 0.9923152162251017705, 0.000000000000000000, 0.1237356522920117774 ) ) ;
#28184=AXIS2_PLACEMENT_3D ( 'NONE', #776, #5116, #18817 ) ;
#28186=CARTESIAN_POINT ( 'NONE',  ( 25.08988466659999972, -73.89104832229999431, -30.05843389639999685 ) ) ;
#28187=CARTESIAN_POINT ( 'NONE',  ( -22.58183123469999742, -70.96441436690000160, 17.76382364619999876 ) ) ;
#28189=CARTESIAN_POINT ( 'NONE',  ( -18.59048430349110959, -19.47314420526488021, 13.19884344879934090 ) ) ;
#28190=FACE_OUTER_BOUND ( 'NONE', #25389, .T. ) ;
#28192=ORIENTED_EDGE ( 'NONE', *, *, #419, .T. ) ;
#28193=EDGE_LOOP ( 'NONE', ( #5302, #910, #342, #4809, #16846 ) ) ;
#28194=CARTESIAN_POINT ( 'NONE',  ( -13.87613801740000063, -58.81368956530000247, 21.27373992140000070 ) ) ;
#28195=CARTESIAN_POINT ( 'NONE',  ( -2.349289058739999714, -62.62089253250000098, -25.05573335040000060 ) ) ;
#28196=CARTESIAN_POINT ( 'NONE',  ( 10.95532170329999921, -36.00000000000000000, -21.46129409690000145 ) ) ;
#28198=CARTESIAN_POINT ( 'NONE',  ( -40.00000000000000000, -69.50000000000000000, 2.464695114669999848E-15 ) ) ;
#28202=CARTESIAN_POINT ( 'NONE',  ( 21.37275086740000063, -35.46743101519999897, -7.456866577549999597 ) ) ;
#28203=DIRECTION ( 'NONE',  ( 0.000000000000000000, 1.000000000000000000, 0.000000000000000000 ) ) ;
#28205=DIRECTION ( 'NONE',  ( 0.000000000000000000, -1.000000000000000000, 0.000000000000000000 ) ) ;
#28206=ORIENTED_EDGE ( 'NONE', *, *, #27159, .F. ) ;
#28207=DIRECTION ( 'NONE',  ( -0.2414462220490755373, 0.000000000000000000, 0.9704142011833033488 ) ) ;
#28208=ADVANCED_FACE ( 'NONE', ( #8022 ), #1304, .F. ) ;
#28209=CARTESIAN_POINT ( 'NONE',  ( -32.18583505495173114, -74.02375072073509443, -22.07098972207143106 ) ) ;
#28213=CYLINDRICAL_SURFACE ( 'NONE', #17597, 1.000000000000000888 ) ;
#28218=ORIENTED_EDGE ( 'NONE', *, *, #17692, .F. ) ;
#28220=CARTESIAN_POINT ( 'NONE',  ( 8.677144207910000517, -37.95796631070000160, -21.92880662259999980 ) ) ;
#28222=CARTESIAN_POINT ( 'NONE',  ( 36.47289904670000027, -79.00000000000000000, -14.78463635570000001 ) ) ;
#28223=ORIENTED_EDGE ( 'NONE', *, *, #8722, .T. ) ;
#28224=FACE_BOUND ( 'NONE', #21959, .T. ) ;
#28225=EDGE_LOOP ( 'NONE', ( #13257, #24712 ) ) ;
#28227=CARTESIAN_POINT ( 'NONE',  ( 47.25012594850000625, -74.74525943189999566, -0.5385019865560000119 ) ) ;
#28228=ORIENTED_EDGE ( 'NONE', *, *, #21327, .F. ) ;
#28230=CARTESIAN_POINT ( 'NONE',  ( -7.332335648789999993, -74.23958658489999607, -39.85912817280000553 ) ) ;
#28233=DIRECTION ( 'NONE',  ( 1.000000000000000000, 0.000000000000000000, 0.000000000000000000 ) ) ;
#28237=DIRECTION ( 'NONE',  ( 0.000000000000000000, 1.000000000000000000, 0.000000000000000000 ) ) ;
#28240=CARTESIAN_POINT ( 'NONE',  ( 25.99900676471481731, -64.47177303794710213, 1.411681790086568355 ) ) ;
#28245=CIRCLE ( 'NONE', #27360, 3.000000000000002665 ) ;
#28247=FACE_OUTER_BOUND ( 'NONE', #15742, .T. ) ;
#28250=CARTESIAN_POINT ( 'NONE',  ( -5.329070518200000398E-15, -19.50000000000000000, 0.000000000000000000 ) ) ;
#28253=CARTESIAN_POINT ( 'NONE',  ( -17.94180966909999597, -19.50000000000000000, 18.81731824139999887 ) ) ;
#28254=CARTESIAN_POINT ( 'NONE',  ( -13.61185859470209891, -68.68656850711893469, 23.08127642874307028 ) ) ;
#28255=( NAMED_UNIT ( * ) SI_UNIT ( $, .STERADIAN. ) SOLID_ANGLE_UNIT ( ) );
#28256=FACE_OUTER_BOUND ( 'NONE', #18149, .T. ) ;
#28257=VERTEX_POINT ( 'NONE', #14441 ) ;
#28259=CARTESIAN_POINT ( 'NONE',  ( 21.34306235150000219, -35.70901436039999766, -7.836671688740000974 ) ) ;
#28261=CIRCLE ( 'NONE', #15222, 38.75000000000000000 ) ;
#28262=CARTESIAN_POINT ( 'NONE',  ( 21.36168465690000318, -36.64960054550000024, -8.292164435260001909 ) ) ;
#28263=CARTESIAN_POINT ( 'NONE',  ( 9.107729735749998667, -35.83389485320000034, -19.55231199680000387 ) ) ;
#28266=B_SPLINE_SURFACE_WITH_KNOTS ( 'NONE', 5, 5, ( 
 ( #2779, #20549, #16308, #24923, #18507, #762 ),
 ( #27111, #9748, #27401, #5393, #11934, #7451 ),
 ( #7151, #20986, #20843, #616, #25221, #7594 ),
 ( #468, #13836, #18368, #25068, #14274, #23171 ),
 ( #27255, #7292, #3213, #11486, #20395, #9312 ),
 ( #4953, #10983, #13194, #7105, #6656, #2442 ) ),
 .UNSPECIFIED., .F., .F., .F.,
 ( 6, 6 ),
 ( 6, 6 ),
 ( 28.77370706320000338, 40.74965893960000329 ),
 ( 0.000000000000000000, 2.000000000000000000 ),
 .UNSPECIFIED. ) ;
#28267=CARTESIAN_POINT ( 'NONE',  ( -2.790536503729999840, -64.24504439390000243, -26.36014981959999659 ) ) ;
#28269=ADVANCED_FACE ( 'NONE', ( #12512 ), #23334, .F. ) ;
#28270=CARTESIAN_POINT ( 'NONE',  ( 7.066909182049999849, -57.47855601759999900, -22.26662627820000040 ) ) ;
#28272=EDGE_LOOP ( 'NONE', ( #26427, #3523, #5800, #24728, #26251, #15234, #6030, #28693 ) ) ;
#28273=EDGE_CURVE ( 'NONE', #9035, #23613, #8717, .T. ) ;
#28274=AXIS2_PLACEMENT_3D ( 'NONE', #16704, #5494, #20955 ) ;
#28277=CARTESIAN_POINT ( 'NONE',  ( 24.11323408290000003, -67.98014023149998764, 11.30446450930000069 ) ) ;
#28281=CARTESIAN_POINT ( 'NONE',  ( -39.45553247920000217, -74.12472287219999600, 7.440556932039999793 ) ) ;
#28283=DIRECTION ( 'NONE',  ( 0.000000000000000000, 0.000000000000000000, -1.000000000000000000 ) ) ;
#28285=ORIENTED_EDGE ( 'NONE', *, *, #15508, .T. ) ;
#28286=EDGE_CURVE ( 'NONE', #3896, #18698, #27384, .T. ) ;
#28287=CARTESIAN_POINT ( 'NONE',  ( -1.269269612537524239, -74.18468793103146197, 47.13810727879495488 ) ) ;
#28288=CARTESIAN_POINT ( 'NONE',  ( 8.986258419809999509, -35.50000000000000000, -19.49544308430000328 ) ) ;
#28289=CARTESIAN_POINT ( 'NONE',  ( 8.328365334949999976, -63.55534151250000008, -23.20786089210000114 ) ) ;
#28290=CARTESIAN_POINT ( 'NONE',  ( -12.06225679689999986, -68.93430146459999719, -25.32738640609999692 ) ) ;
#28291=CARTESIAN_POINT ( 'NONE',  ( 23.29550765120000122, -59.99252585180000352, 10.45228063749999947 ) ) ;
#28292=CARTESIAN_POINT ( 'NONE',  ( -15.57528087630000080, -80.00000000000000000, 40.61740797039999507 ) ) ;
#28296=CARTESIAN_POINT ( 'NONE',  ( -34.89999999999999858, -84.50000000000000000, 0.000000000000000000 ) ) ;
#28298=CARTESIAN_POINT ( 'NONE',  ( 8.986258609349999205, -35.49999998740000251, -19.49544309740000259 ) ) ;
#28299=CARTESIAN_POINT ( 'NONE',  ( 22.23400538530000148, -18.50000000000000000, 1.911111031959999984 ) ) ;
#28303=CARTESIAN_POINT ( 'NONE',  ( 19.90557383419999837, -34.65022531199999634, -8.965967189899998857 ) ) ;
#28306=ORIENTED_EDGE ( 'NONE', *, *, #7185, .T. ) ;
#28307=CARTESIAN_POINT ( 'NONE',  ( -36.59277592640000165, -74.50000000000000000, -27.40038777100000189 ) ) ;
#28311=ORIENTED_EDGE ( 'NONE', *, *, #24510, .F. ) ;
#28312=EDGE_CURVE ( 'NONE', #19001, #27953, #2242, .T. ) ;
#28315=CARTESIAN_POINT ( 'NONE',  ( 22.03468988030000020, -19.46429362099999949, -0.1835573589099999958 ) ) ;
#28316=DIRECTION ( 'NONE',  ( 0.000000000000000000, 1.000000000000000000, 0.000000000000000000 ) ) ;
#28319=EDGE_CURVE ( 'NONE', #8501, #14660, #18562, .T. ) ;
#28323=CARTESIAN_POINT ( 'NONE',  ( -22.57449023189999693, -71.67452784319999637, 17.69693788339999685 ) ) ;
#28325=B_SPLINE_CURVE_WITH_KNOTS ( 'NONE', 5,
 ( #9323, #4521, #4670, #24790, #4828, #10903, #24487, #2502, #13253 ),
 .UNSPECIFIED., .F., .F.,
 ( 6, 3, 6 ),
 ( 0.000000000000000000, 0.5000000000000000000, 1.000000000000000000 ),
 .UNSPECIFIED. ) ;
#28328=CARTESIAN_POINT ( 'NONE',  ( 6.846103682120000755, -36.12241484350000320, -21.55427193710000111 ) ) ;
#28330=ORIENTED_EDGE ( 'NONE', *, *, #19241, .F. ) ;
#28331=CARTESIAN_POINT ( 'NONE',  ( 7.765654448670000320, -18.50000000000000000, -19.88144340339999872 ) ) ;
#28332=ORIENTED_EDGE ( 'NONE', *, *, #10628, .T. ) ;
#28333=DIRECTION ( 'NONE',  ( 0.000000000000000000, 1.000000000000000000, 0.000000000000000000 ) ) ;
#28335=CARTESIAN_POINT ( 'NONE',  ( -2.698605191359999544, -63.31646347429999366, -26.06520130500000221 ) ) ;
#28339=CARTESIAN_POINT ( 'NONE',  ( -20.45998242170000125, -52.56313962710000709, 14.78974999389999923 ) ) ;
#28340=AXIS2_PLACEMENT_3D ( 'NONE', #25462, #3454, #1420 ) ;
#28342=AXIS2_PLACEMENT_3D ( 'NONE', #25004, #16552, #27495 ) ;
#28344=CARTESIAN_POINT ( 'NONE',  ( 47.25000000000000000, -73.00000000000000000, 2.433892081919999696E-15 ) ) ;
#28350=CARTESIAN_POINT ( 'NONE',  ( 22.42985924190000091, -18.87168151170000030, 9.783895484440000345 ) ) ;
#28352=CARTESIAN_POINT ( 'NONE',  ( -19.90266458450000187, -57.44036972699999666, 14.20824301549999902 ) ) ;
#28354=CARTESIAN_POINT ( 'NONE',  ( 23.93802380909999883, -64.72767011149998950, -9.438994838039999280 ) ) ;
#28360=DIRECTION ( 'NONE',  ( 0.000000000000000000, -1.000000000000000000, 0.000000000000000000 ) ) ;
#28361=CARTESIAN_POINT ( 'NONE',  ( -32.59032919970000108, -74.28456446479999897, -21.87590318590000038 ) ) ;
#28362=CARTESIAN_POINT ( 'NONE',  ( 37.29611236860000645, -79.99999990109998294, -13.74999974979999884 ) ) ;
#28364=EDGE_CURVE ( 'NONE', #2148, #16095, #20299, .T. ) ;
#28366=CARTESIAN_POINT ( 'NONE',  ( -0.8787802303807957793, -79.83340751218206321, 47.19654850980432315 ) ) ;
#28367=ORIENTED_EDGE ( 'NONE', *, *, #27147, .T. ) ;
#28369=DIRECTION ( 'NONE',  ( -0.09756097560976770278, 0.000000000000000000, -0.9952295494196654602 ) ) ;
#28371=CARTESIAN_POINT ( 'NONE',  ( 21.54084985340000102, -53.82492386869999734, 10.13856859999999926 ) ) ;
#28372=DIRECTION ( 'NONE',  ( 0.9952295494196655712, 0.000000000000000000, 0.09756097560976655092 ) ) ;
#28375=ORIENTED_EDGE ( 'NONE', *, *, #8190, .F. ) ;
#28376=AXIS2_PLACEMENT_3D ( 'NONE', #26003, #23963, #1550 ) ;
#28378=DIRECTION ( 'NONE',  ( 0.000000000000000000, -1.000000000000000000, 0.000000000000000000 ) ) ;
#28380=CARTESIAN_POINT ( 'NONE',  ( -21.60034894820000062, -79.50000026560000776, -32.77174736439999947 ) ) ;
#28382=CARTESIAN_POINT ( 'NONE',  ( 24.22382764319999993, -64.24504439390000243, 10.76339940740000145 ) ) ;
#28383=ORIENTED_EDGE ( 'NONE', *, *, #742, .T. ) ;
#28384=DIRECTION ( 'NONE',  ( 0.4794255386042038936, 0.000000000000000000, 0.8775825618903723147 ) ) ;
#28386=CARTESIAN_POINT ( 'NONE',  ( 25.14694229440000228, -65.07443093669999712, -0.3759436444569999591 ) ) ;
#28387=DIRECTION ( 'NONE',  ( 0.000000000000000000, -1.000000000000000000, 0.000000000000000000 ) ) ;
#28388=CARTESIAN_POINT ( 'NONE',  ( 10.77859369565145897, -72.53894543248756577, -26.82390758811301623 ) ) ;
#28392=CARTESIAN_POINT ( 'NONE',  ( 8.793068625647139314, -37.96202148991682890, -22.01683846075131967 ) ) ;
#28394=DIRECTION ( 'NONE',  ( 1.000000000000000000, 0.000000000000000000, -1.261617073437678048E-15 ) ) ;
#28397=CIRCLE ( 'NONE', #14893, 39.75000000000000000 ) ;
#28398=AXIS2_PLACEMENT_3D ( 'NONE', #10634, #21740, #6144 ) ;
#28400=EDGE_CURVE ( 'NONE', #24581, #7391, #4061, .T. ) ;
#28402=CARTESIAN_POINT ( 'NONE',  ( 20.72386479999999764, -35.83655893530000469, -8.803829908180000885 ) ) ;
#28404=CARTESIAN_POINT ( 'NONE',  ( 19.56129018700000088, -35.88702891199999812, -9.158871637020000733 ) ) ;
#28406=EDGE_CURVE ( 'NONE', #5383, #10466, #13371, .T. ) ;
#28407=EDGE_LOOP ( 'NONE', ( #5058, #2133, #23330, #10349, #11600 ) ) ;
#28411=CARTESIAN_POINT ( 'NONE',  ( -0.5658552861894227126, -18.49999996075941411, -21.28277172089477887 ) ) ;
#28413=CARTESIAN_POINT ( 'NONE',  ( 7.215414233289999757, -74.50000000000000000, -40.70731707320000226 ) ) ;
#28414=CARTESIAN_POINT ( 'NONE',  ( 7.675802715190000569, -57.47600051900000295, -22.13628143409999893 ) ) ;
#28415=CARTESIAN_POINT ( 'NONE',  ( -11.08724219600000183, -18.85485920039999996, -18.88147462500000273 ) ) ;
#28416=CIRCLE ( 'NONE', #8396, 7.250000000000000000 ) ;
#28421=AXIS2_PLACEMENT_3D ( 'NONE', #5715, #3541, #23502 ) ;
#28422=CARTESIAN_POINT ( 'NONE',  ( 22.78606152149999886, -34.66500525210000205, 0.4244034508280000173 ) ) ;
#28423=CARTESIAN_POINT ( 'NONE',  ( 24.61976394740000273, -69.66720773109999243, 11.67393097119999901 ) ) ;
#28425=ORIENTED_EDGE ( 'NONE', *, *, #13200, .T. ) ;
#28426=CARTESIAN_POINT ( 'NONE',  ( -40.70731707320000226, -74.50000000000000000, 7.215414233289999757 ) ) ;
#28428=DIRECTION ( 'NONE',  ( 0.000000000000000000, -1.000000000000000000, 0.000000000000000000 ) ) ;
#28429=CARTESIAN_POINT ( 'NONE',  ( -0.5856201115350000430, -19.46363745430000236, -22.02586699820000149 ) ) ;
#28430=CARTESIAN_POINT ( 'NONE',  ( 4.037078284719999375E-15, -74.00000000000000000, -40.00000000000000000 ) ) ;
#28431=ORIENTED_EDGE ( 'NONE', *, *, #17942, .F. ) ;
#28432=CARTESIAN_POINT ( 'NONE',  ( 26.13146017414465305, -67.22652123492960641, -0.08258631501461731472 ) ) ;
#28433=DIRECTION ( 'NONE',  ( 0.000000000000000000, 1.000000000000000000, 0.000000000000000000 ) ) ;
#28434=CARTESIAN_POINT ( 'NONE',  ( 9.160187750109999527, -60.39422136570000532, -22.93664085480000381 ) ) ;
#28435=CARTESIAN_POINT ( 'NONE',  ( -12.45933098930000149, -68.79094677780000211, -23.93918507130000251 ) ) ;
#28436=CARTESIAN_POINT ( 'NONE',  ( 21.63571321169999706, -57.45864736019999697, 10.20337583880000132 ) ) ;
#28437=CARTESIAN_POINT ( 'NONE',  ( -12.17175116130000134, -57.47855602620000326, -19.93971707270000238 ) ) ;
#28439=CIRCLE ( 'NONE', #24737, 1.999999999999999334 ) ;
#28442=CIRCLE ( 'NONE', #1475, 3.499999999999999556 ) ;
#28443=EDGE_CURVE ( 'NONE', #15667, #1954, #20378, .T. ) ;
#28445=DIRECTION ( 'NONE',  ( -8.326672684689999093E-17, 0.000000000000000000, -1.000000000000000000 ) ) ;
#28448=ORIENTED_EDGE ( 'NONE', *, *, #6726, .F. ) ;
#28450=ADVANCED_FACE ( 'NONE', ( #4806 ), #18543, .T. ) ;
#28454=EDGE_LOOP ( 'NONE', ( #242, #11747, #25070, #20209 ) ) ;
#28456=VERTEX_POINT ( 'NONE', #16300 ) ;
#28457=CARTESIAN_POINT ( 'NONE',  ( 8.670860352240000068, -36.23359953109999765, -21.01414488289999838 ) ) ;
#28461=CARTESIAN_POINT ( 'NONE',  ( 22.46071958670000157, -18.85738404119999956, 1.064556727120000046 ) ) ;
#28464=ORIENTED_EDGE ( 'NONE', *, *, #27910, .T. ) ;
#28465=DIRECTION ( 'NONE',  ( 0.000000000000000000, -1.000000000000000000, 0.000000000000000000 ) ) ;
#28466=AXIS2_PLACEMENT_3D ( 'NONE', #13081, #21696, #2038 ) ;
#28467=CARTESIAN_POINT ( 'NONE',  ( -7.615241770509999806E-12, -84.00000000000000000, -9.798384326129999571E-12 ) ) ;
#28470=CARTESIAN_POINT ( 'NONE',  ( -18.54060892918908721, -19.47131810279708830, 13.04730683233061583 ) ) ;
#28471=CARTESIAN_POINT ( 'NONE',  ( 7.664900609720000091, -35.15980160819999867, -21.28729237769999827 ) ) ;
#28473=EDGE_LOOP ( 'NONE', ( #19537, #14863, #8127, #20293 ) ) ;
#28474=CARTESIAN_POINT ( 'NONE',  ( 7.730596112549999788, -19.15810972889999775, -20.62158084869999897 ) ) ;
#28475=CARTESIAN_POINT ( 'NONE',  ( 22.96193664180000127, -37.37167648650000018, -9.452942635470000354 ) ) ;
#28477=ORIENTED_EDGE ( 'NONE', *, *, #27465, .F. ) ;
#28480=CARTESIAN_POINT ( 'NONE',  ( -1.447122895489999950, -60.30889230620000063, -23.76394779129999790 ) ) ;
#28481=CARTESIAN_POINT ( 'NONE',  ( 9.063914967340000572, -37.97325489250000174, -22.27494422110000016 ) ) ;
#28484=FACE_OUTER_BOUND ( 'NONE', #17636, .T. ) ;
#28487=CARTESIAN_POINT ( 'NONE',  ( 21.18684992340000051, -34.75995393510000042, -7.793340637920000091 ) ) ;
#28488=CARTESIAN_POINT ( 'NONE',  ( 7.135466514619999145, -73.65708014139998738, -38.71640952649999434 ) ) ;
#28489=ORIENTED_EDGE ( 'NONE', *, *, #18509, .T. ) ;
#28491=CARTESIAN_POINT ( 'NONE',  ( 19.71712935880000117, -26.09894693429999890, 10.34883699620000108 ) ) ;
#28493=CARTESIAN_POINT ( 'NONE',  ( 21.60905208779999853, -19.48534420260000033, 9.488781546969999425 ) ) ;
#28497=VERTEX_POINT ( 'NONE', #2632 ) ;
#28501=AXIS2_PLACEMENT_3D ( 'NONE', #1838, #6639, #28759 ) ;
#28504=CARTESIAN_POINT ( 'NONE',  ( 11.51925138921799352, -70.92537290725283583, -27.02474293696387520 ) ) ;
#28505=CARTESIAN_POINT ( 'NONE',  ( -32.47291160230000173, -74.11800272920001476, -21.73792012110000016 ) ) ;
#28506=CARTESIAN_POINT ( 'NONE',  ( 36.75261502460000429, -80.49999978700000725, -13.77875165610000074 ) ) ;
#28507=VERTEX_POINT ( 'NONE', #25058 ) ;
#28508=ADVANCED_FACE ( 'NONE', ( #5092 ), #8505, .T. ) ;
#28512=CARTESIAN_POINT ( 'NONE',  ( 19.92559242949999998, -35.99861502429999405, -9.426072644010000445 ) ) ;
#28514=VERTEX_POINT ( 'NONE', #5387 ) ;
#28516=DIRECTION ( 'NONE',  ( -1.000000000000000000, 0.000000000000000000, -5.551115123129999410E-17 ) ) ;
#28521=ORIENTED_EDGE ( 'NONE', *, *, #24039, .T. ) ;
#28523=CARTESIAN_POINT ( 'NONE',  ( -34.47145558279999733, -74.50000000000000000, -23.86485386499999706 ) ) ;
#28525=CARTESIAN_POINT ( 'NONE',  ( -22.17563740510000159, -80.50000000000000000, -32.38675284270000532 ) ) ;
#28527=CARTESIAN_POINT ( 'NONE',  ( 25.16030248577766670, -66.99910240652532423, 10.87945431192736301 ) ) ;
#28528=ORIENTED_EDGE ( 'NONE', *, *, #20744, .T. ) ;
#28535=CARTESIAN_POINT ( 'NONE',  ( 10.94782719350765632, -72.47277773194394968, -26.85191487759274409 ) ) ;
#28537=EDGE_LOOP ( 'NONE', ( #8042, #5251, #20217, #28670 ) ) ;
#28539=CARTESIAN_POINT ( 'NONE',  ( 8.408333318189998979E-15, -74.00000000000000000, 40.00000000000000000 ) ) ;
#28550=ORIENTED_EDGE ( 'NONE', *, *, #18163, .T. ) ;
#28552=CARTESIAN_POINT ( 'NONE',  ( 21.42228108240000140, -36.78979570469999771, -8.360528863789999932 ) ) ;
#28554=VERTEX_POINT ( 'NONE', #25770 ) ;
#28555=CARTESIAN_POINT ( 'NONE',  ( 8.472395020760000506, -37.95144078679999922, -21.79230213740000011 ) ) ;
#28557=DIRECTION ( 'NONE',  ( 0.000000000000000000, 1.000000000000000000, 0.000000000000000000 ) ) ;
#28560=CARTESIAN_POINT ( 'NONE',  ( 8.496651354449999971, -44.91471497059999507, -21.93056824609999822 ) ) ;
#28561=AXIS2_PLACEMENT_3D ( 'NONE', #2805, #20123, #192 ) ;
#28562=CARTESIAN_POINT ( 'NONE',  ( -11.41039530250000134, -19.15810975349999978, -18.83652256670000114 ) ) ;
#28564=VERTEX_POINT ( 'NONE', #27951 ) ;
#28566=CARTESIAN_POINT ( 'NONE',  ( 22.11862230030000021, -19.46485671829999831, 0.2283802166510000287 ) ) ;
#28567=CARTESIAN_POINT ( 'NONE',  ( 24.39287928049999721, -64.76590626969999676, 10.80146537900000148 ) ) ;
#28568=CARTESIAN_POINT ( 'NONE',  ( 39.06010443568764856, -73.53996501802137686, 7.188997797742533891 ) ) ;
#28570=ADVANCED_FACE ( 'NONE', ( #1044 ), #24556, .F. ) ;
#28571=DIRECTION ( 'NONE',  ( 0.000000000000000000, -1.000000000000000000, 0.000000000000000000 ) ) ;
#28575=EDGE_CURVE ( 'NONE', #134, #3865, #24477, .T. ) ;
#28576=CARTESIAN_POINT ( 'NONE',  ( 25.64005057298560786, -66.15241698523519176, -0.2567751734516250939 ) ) ;
#28578=CARTESIAN_POINT ( 'NONE',  ( 7.379008025240000102, -59.04182300869999978, -22.22481934930000236 ) ) ;
#28579=CARTESIAN_POINT ( 'NONE',  ( -12.08593779409999946, -68.40342018370000687, -24.66380339859999893 ) ) ;
#28580=ADVANCED_FACE ( 'NONE', ( #14538 ), #1305, .T. ) ;
#28581=CARTESIAN_POINT ( 'NONE',  ( 21.15302165019999947, -58.77396426510000538, 10.53974575699999860 ) ) ;
#28582=FACE_OUTER_BOUND ( 'NONE', #15230, .T. ) ;
#28584=ADVANCED_FACE ( 'NONE', ( #12068 ), #5929, .T. ) ;
#28587=AXIS2_PLACEMENT_3D ( 'NONE', #22987, #11890, #7397 ) ;
#28588=CARTESIAN_POINT ( 'NONE',  ( 9.734617625879998830E-15, -69.50000000000000000, -46.75000000000000000 ) ) ;
#28590=CIRCLE ( 'NONE', #26745, 28.68388914670000034 ) ;
#28593=DIRECTION ( 'NONE',  ( 0.000000000000000000, 1.000000000000000000, 0.000000000000000000 ) ) ;
#28595=ORIENTED_EDGE ( 'NONE', *, *, #7861, .F. ) ;
#28596=DIRECTION ( 'NONE',  ( 0.000000000000000000, 1.000000000000000000, 0.000000000000000000 ) ) ;
#28598=ORIENTED_EDGE ( 'NONE', *, *, #6345, .F. ) ;
#28599=CARTESIAN_POINT ( 'NONE',  ( 8.229163310540000609, -36.50138226700000388, -21.31937092320000104 ) ) ;
#28602=CARTESIAN_POINT ( 'NONE',  ( 20.33060048479999793, -36.00000012589999443, -9.320855386229998985 ) ) ;
#28603=CARTESIAN_POINT ( 'NONE',  ( 22.18378897850000442, -19.15825174789999963, 0.3668181516639999473 ) ) ;
#28604=CARTESIAN_POINT ( 'NONE',  ( -7.135466514619999145, -73.65708014139998738, 38.71640952649999434 ) ) ;
#28606=ORIENTED_EDGE ( 'NONE', *, *, #14886, .T. ) ;
#28607=CARTESIAN_POINT ( 'NONE',  ( -2.131628207279999844E-14, -80.50000000000000000, 1.776356839399999922E-14 ) ) ;
#28608=CARTESIAN_POINT ( 'NONE',  ( -12.98525885659999979, -18.62004674389999792, 19.04822181160000483 ) ) ;
#28610=ADVANCED_FACE ( 'NONE', ( #2847 ), #21193, .F. ) ;
#28615=DIRECTION ( 'NONE',  ( 0.000000000000000000, -1.000000000000000000, 0.000000000000000000 ) ) ;
#28618=CARTESIAN_POINT ( 'NONE',  ( 8.007516345569998251, -18.50000000000000000, -19.07516293619999814 ) ) ;
#28619=CARTESIAN_POINT ( 'NONE',  ( 22.06017367829999998, -36.00000000000000000, -10.88627920610000110 ) ) ;
#28621=CARTESIAN_POINT ( 'NONE',  ( -1.972916809350000023, -62.77692288639999418, -24.64506619409999999 ) ) ;
#28623=CARTESIAN_POINT ( 'NONE',  ( -20.02271108649999576, -55.00753887609999992, 14.43701757890000081 ) ) ;
#28624=DIRECTION ( 'NONE',  ( 0.9704142011833034598, 0.000000000000000000, -0.2414462220490750377 ) ) ;
#28627=CARTESIAN_POINT ( 'NONE',  ( 21.38036727909999613, -35.41472438419999946, -7.365645260430000008 ) ) ;
#28628=CARTESIAN_POINT ( 'NONE',  ( 7.229366192820000592, -73.50064222369999811, -39.23631979990000218 ) ) ;
#28631=CARTESIAN_POINT ( 'NONE',  ( -14.23452928849999921, -80.18504828089999137, 36.64500871850000152 ) ) ;
#28632=CARTESIAN_POINT ( 'NONE',  ( 21.17154477089999887, -39.34784663159999951, 9.865579592129998687 ) ) ;
#28634=DIRECTION ( 'NONE',  ( 0.000000000000000000, 1.000000000000000000, 0.000000000000000000 ) ) ;
#28637=CARTESIAN_POINT ( 'NONE',  ( 7.135467304789999687, -73.50000064450000536, -38.71640881029999548 ) ) ;
#28638=ORIENTED_EDGE ( 'NONE', *, *, #19091, .F. ) ;
#28641=CARTESIAN_POINT ( 'NONE',  ( -7.135467304789999687, -73.50000064450000536, 38.71640881029999548 ) ) ;
#28644=ADVANCED_FACE ( 'NONE', ( #17956 ), #24092, .T. ) ;
#28645=CARTESIAN_POINT ( 'NONE',  ( 11.81986579350000000, -72.00000321289999761, -27.35691362350000233 ) ) ;
#28646=ORIENTED_EDGE ( 'NONE', *, *, #13728, .F. ) ;
#28649=VERTEX_POINT ( 'NONE', #4405 ) ;
#28651=ORIENTED_EDGE ( 'NONE', *, *, #26618, .T. ) ;
#28656=PLANE ( 'NONE',  #2965 ) ;
#28657=B_SPLINE_CURVE_WITH_KNOTS ( 'NONE', 5,
 ( #8237, #17130, #26025, #6046, #14929, #27145, #26704, #22041, #6594 ),
 .UNSPECIFIED., .F., .F.,
 ( 6, 3, 6 ),
 ( 0.000000000000000000, 0.5000000000000000000, 1.000000000000000000 ),
 .UNSPECIFIED. ) ;
#28660=CARTESIAN_POINT ( 'NONE',  ( -7.955258795889999845, -74.00000000000000000, 36.66863921009999672 ) ) ;
#28661=ORIENTED_EDGE ( 'NONE', *, *, #21870, .T. ) ;
#28662=CARTESIAN_POINT ( 'NONE',  ( 36.22844186549999534, -74.00000000000000000, -13.75000000000000000 ) ) ;
#28663=EDGE_CURVE ( 'NONE', #8713, #12443, #8465, .T. ) ;
#28667=CARTESIAN_POINT ( 'NONE',  ( -34.89999999999999858, -86.00000000000000000, 0.000000000000000000 ) ) ;
#28668=CARTESIAN_POINT ( 'NONE',  ( 10.24074127443738824, -72.71346136330345189, -26.83295873777677443 ) ) ;
#28669=CARTESIAN_POINT ( 'NONE',  ( -18.80282716219999983, -18.50000000000000000, 14.71063029340000128 ) ) ;
#28670=ORIENTED_EDGE ( 'NONE', *, *, #8722, .F. ) ;
#28671=DIRECTION ( 'NONE',  ( 0.4794255386042036715, 0.000000000000000000, 0.8775825618903724257 ) ) ;
#28673=DIRECTION ( 'NONE',  ( 0.000000000000000000, 1.000000000000000000, 0.000000000000000000 ) ) ;
#28674=CARTESIAN_POINT ( 'NONE',  ( -0.5413028987460000163, -57.47855601759999900, -23.35488904649999853 ) ) ;
#28677=B_SPLINE_CURVE_WITH_KNOTS ( 'NONE', 3,
 ( #9360, #26715, #15764, #2535, #26860, #24963, #18261, #13287, #6900, #11076, #4860, #8912, #13585, #13433, #19993, #22190, #6755, #66, #17967, #24518, #22493, #13738, #15618, #656, #27008, #4555, #2385, #11241, #7195, #7049, #24820, #20147, #4993, #22638, #2678 ),
 .UNSPECIFIED., .F., .F.,
 ( 4, 2, 2, 2, 2, 2, 2, 1, 1, 2, 2, 2, 2, 1, 1, 1, 2, 2, 2, 4 ),
 ( 0.000000000000000000, 0.1249999999999757139, 0.1874999999999635847, 0.2187499999999575062, 0.2499999999999514277, 0.3749999999999258926, 0.4374999999999140687, 0.4687499999999091282, 0.4843749999999067413, 0.4921874999999054645, 0.4999999999999042988, 0.6249999999999072964, 0.6874999999999088507, 0.7187499999999096278, 0.7343749999999100719, 0.7421874999999102940, 0.7460937499999104050, 0.7499999999999105160, 0.8749999999999552580, 1.000000000000000000 ),
 .UNSPECIFIED. ) ;
#28679=EDGE_LOOP ( 'NONE', ( #21205, #23744, #13950, #8238, #3219 ) ) ;
#28683=CARTESIAN_POINT ( 'NONE',  ( -12.58874986569999876, -49.85661345660000165, 20.06068440369999806 ) ) ;
#28684=CARTESIAN_POINT ( 'NONE',  ( 9.270471387543576469, -35.95566652371019956, -19.65325541728526915 ) ) ;
#28685=ORIENTED_EDGE ( 'NONE', *, *, #11674, .F. ) ;
#28686=CARTESIAN_POINT ( 'NONE',  ( 30.97095665689999677, -72.00000182920000213, -20.30102787789999752 ) ) ;
#28687=CARTESIAN_POINT ( 'NONE',  ( -3.375526912685365755, -68.14528050418705618, -27.58514050670897788 ) ) ;
#28690=CARTESIAN_POINT ( 'NONE',  ( -47.25000000000000000, -74.50000000000000000, 3.352534721190000231E-15 ) ) ;
#28691=CARTESIAN_POINT ( 'NONE',  ( 9.391640714739999396, -49.05622624330000292, -22.99217564430000138 ) ) ;
#28693=ORIENTED_EDGE ( 'NONE', *, *, #22511, .T. ) ;
#28696=CARTESIAN_POINT ( 'NONE',  ( -14.13576225364580097, -80.50000169811967510, 36.61638830656482213 ) ) ;
#28697=CARTESIAN_POINT ( 'NONE',  ( 40.25190969013254971, -74.15297958022469516, 7.245634850467974175 ) ) ;
#28698=EDGE_LOOP ( 'NONE', ( #8997, #9499, #2761, #9659, #28489 ) ) ;
#28699=FACE_OUTER_BOUND ( 'NONE', #27780, .T. ) ;
#28701=CARTESIAN_POINT ( 'NONE',  ( -14.47984945249999988, -79.50000000000000000, 46.16378133559999952 ) ) ;
#28702=ORIENTED_EDGE ( 'NONE', *, *, #17104, .F. ) ;
#28704=CARTESIAN_POINT ( 'NONE',  ( 27.13959279059999830, -67.66818392540000104, 1.745401794850000021 ) ) ;
#28706=CARTESIAN_POINT ( 'NONE',  ( 24.11566500995067841, -74.16082669357513169, -30.79957691333705938 ) ) ;
#28709=CARTESIAN_POINT ( 'NONE',  ( -11.02548659089999994, -34.66500525210000205, -19.94550985520000097 ) ) ;
#28710=VERTEX_POINT ( 'NONE', #13573 ) ;
#28713=CIRCLE ( 'NONE', #17565, 0.5000000000000027756 ) ;
#28715=EDGE_CURVE ( 'NONE', #19884, #26794, #25878, .T. ) ;
#28716=CARTESIAN_POINT ( 'NONE',  ( -3.299060192128916658, -18.50000000000001776, -24.39335967336940314 ) ) ;
#28721=ADVANCED_FACE ( 'NONE', ( #2221 ), #19982, .T. ) ;
#28723=CARTESIAN_POINT ( 'NONE',  ( 20.86759588749999850, -25.49730385779999864, -7.704475033939999662 ) ) ;
#28726=ORIENTED_EDGE ( 'NONE', *, *, #22594, .F. ) ;
#28727=FACE_OUTER_BOUND ( 'NONE', #25139, .T. ) ;
#28730=CYLINDRICAL_SURFACE ( 'NONE', #3867, 0.9999999999999991118 ) ;
#28732=ORIENTED_EDGE ( 'NONE', *, *, #25678, .T. ) ;
#28734=CARTESIAN_POINT ( 'NONE',  ( 21.33676307760000057, -18.50000000000000000, -0.4490903458859999975 ) ) ;
#28738=VECTOR ( 'NONE', #26658, 1000.000000000000000 ) ;
#28742=B_SPLINE_SURFACE_WITH_KNOTS ( 'NONE', 5, 5, ( 
 ( #9052, #14172, #3112, #2815, #647, #16194 ),
 ( #22925, #5137, #9783, #23203, #16630, #24954 ),
 ( #21023, #20584, #16347, #3249, #9635, #20879 ),
 ( #11521, #18249, #7765, #14017, #25102, #25526 ),
 ( #7327, #2967, #939, #11966, #20428, #11825 ),
 ( #500, #9348, #20738, #13870, #797, #1082 ) ),
 .UNSPECIFIED., .F., .F., .F.,
 ( 6, 6 ),
 ( 6, 6 ),
 ( 26.13957982990000062, 31.08299525729999857 ),
 ( 0.000000000000000000, 2.000000000000000000 ),
 .UNSPECIFIED. ) ;
#28744=CARTESIAN_POINT ( 'NONE',  ( -12.04235212070000216, -66.18149755920001098, -24.32398530919999757 ) ) ;
#28745=CARTESIAN_POINT ( 'NONE',  ( 19.97576656849999921, -55.50000000000000000, -19.97576656849999921 ) ) ;
#28747=CARTESIAN_POINT ( 'NONE',  ( 19.18395247690000360, -26.81058807039999792, -9.003807793969999196 ) ) ;
#28748=ORIENTED_EDGE ( 'NONE', *, *, #8478, .F. ) ;
#28749=CARTESIAN_POINT ( 'NONE',  ( 26.22877582859999990, -72.82938648530000592, 11.61106434019999867 ) ) ;
#28751=DIRECTION ( 'NONE',  ( 1.000000000000000000, 0.000000000000000000, 0.000000000000000000 ) ) ;
#28752=CARTESIAN_POINT ( 'NONE',  ( -14.39036416260000095, -64.35840737179999849, 21.98073843050000065 ) ) ;
#28755=CARTESIAN_POINT ( 'NONE',  ( 9.067410242710000290, -37.66179406690000064, -22.27253134700000103 ) ) ;
#28758=CARTESIAN_POINT ( 'NONE',  ( -20.19582590579999959, -52.57401960349999825, 14.62459034920000001 ) ) ;
#28759=DIRECTION ( 'NONE',  ( 1.000000000000000000, 0.000000000000000000, 0.000000000000000000 ) ) ;
#28761=CARTESIAN_POINT ( 'NONE',  ( 20.29489564980377025, -19.47276819030039618, -8.375690697078448821 ) ) ;
#28765=CARTESIAN_POINT ( 'NONE',  ( 7.283540599140000182, -74.14144493730000818, -39.92825895720000062 ) ) ;
#28766=ORIENTED_EDGE ( 'NONE', *, *, #4069, .F. ) ;
#28767=EDGE_CURVE ( 'NONE', #10513, #28649, #28261, .T. ) ;
#28768=CARTESIAN_POINT ( 'NONE',  ( -40.70731707320000226, -84.00000000000000000, -7.215414233289999757 ) ) ;
#28769=EDGE_CURVE ( 'NONE', #19738, #20825, #16195, .T. ) ;
#28771=CIRCLE ( 'NONE', #3666, 0.4999999999999982236 ) ;
#28772=CARTESIAN_POINT ( 'NONE',  ( -10.39027439690000065, -18.50000000000000000, -18.36289120799999708 ) ) ;
#28773=CARTESIAN_POINT ( 'NONE',  ( 19.97576656849999921, -18.50000000000000000, -19.97576656849999921 ) ) ;
#28776=DIRECTION ( 'NONE',  ( 0.000000000000000000, -1.000000000000000000, 0.000000000000000000 ) ) ;
#28781=FACE_OUTER_BOUND ( 'NONE', #26256, .T. ) ;
#28782=DIRECTION ( 'NONE',  ( 0.09756097560976760563, 0.000000000000000000, 0.9952295494196654602 ) ) ;
#28786=FACE_BOUND ( 'NONE', #4015, .T. ) ;
#28787=CARTESIAN_POINT ( 'NONE',  ( 36.82078951440000480, -80.19526215299998739, -13.76146197529999959 ) ) ;
#28788=ORIENTED_EDGE ( 'NONE', *, *, #16653, .F. ) ;
#28789=CIRCLE ( 'NONE', #18601, 3.750000000000000000 ) ;
#28792=DIRECTION ( 'NONE',  ( 1.000000000000000000, 0.000000000000000000, 0.000000000000000000 ) ) ;
#28794=CARTESIAN_POINT ( 'NONE',  ( -0.5413028987460000163, -57.47855601759999900, -23.35488904649999853 ) ) ;
#28795=ORIENTED_EDGE ( 'NONE', *, *, #7604, .F. ) ;
#28796=ADVANCED_FACE ( 'NONE', ( #4256 ), #6743, .T. ) ;
#28799=ORIENTED_EDGE ( 'NONE', *, *, #23398, .T. ) ;
#28801=CARTESIAN_POINT ( 'NONE',  ( -40.00000000000000000, -69.50000000000000000, 1.332267629549999902E-15 ) ) ;
#28802=CARTESIAN_POINT ( 'NONE',  ( 36.22844186549999534, -74.00000000000000000, -13.75000000000000000 ) ) ;
ENDSEC;
END-ISO-10303-21;
